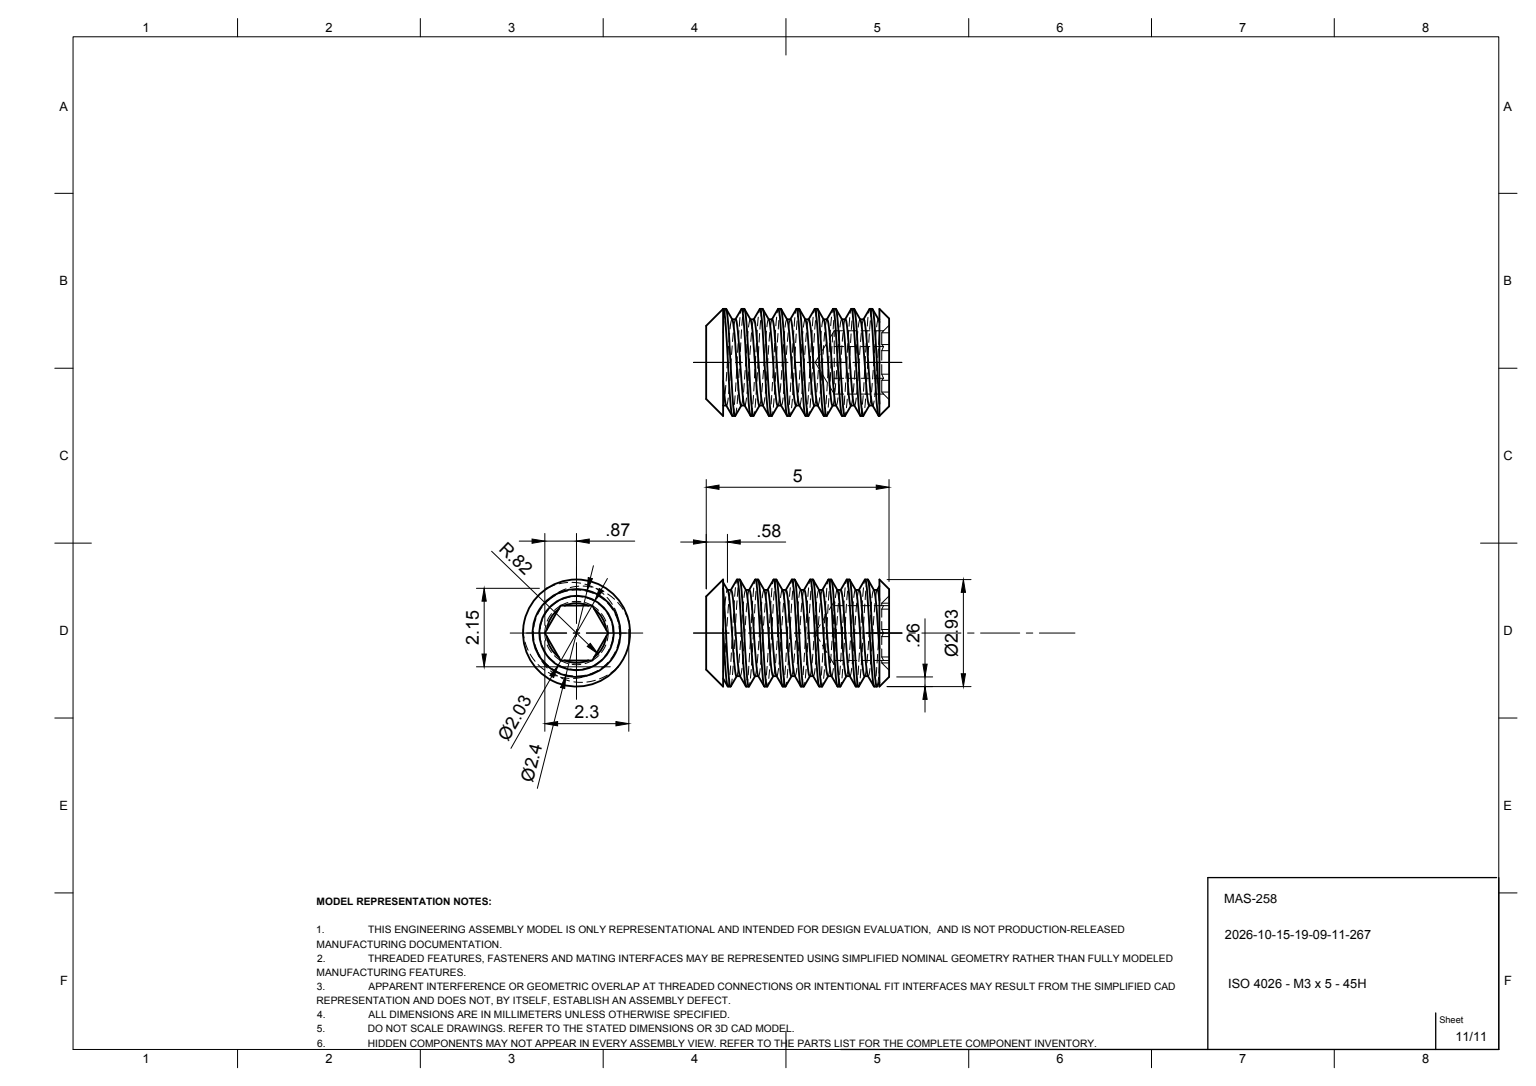
ISO-10303-21;
HEADER;
/* Generated by software containing ST-Developer
 * from STEP Tools, Inc. (www.steptools.com) 
 */

FILE_DESCRIPTION(
/* description */ (''),
/* implementation_level */ '2;1');

FILE_NAME(
/* name */ 'ISO 4026 - M3 x 5 - 45H.step',
/* time_stamp */ '2026-10-15T12:29:06-07:00',
/* author */ (''),
/* organization */ (''),
/* preprocessor_version */ 'ST-DEVELOPER v20.2',
/* originating_system */ 'Autodesk Translation Framework v15.15.0.0',
/* authorisation */ '');

FILE_SCHEMA (('AUTOMOTIVE_DESIGN { 1 0 10303 214 3 1 1 }'));
ENDSEC;

DATA;
#10=MECHANICAL_DESIGN_GEOMETRIC_PRESENTATION_REPRESENTATION('',(#1747),#135282);
#104=(
BOUNDED_CURVE()
B_SPLINE_CURVE(2,(#84021,#84022,#84023),.UNSPECIFIED.,.F.,.F.)
B_SPLINE_CURVE_WITH_KNOTS((3,3),(0.,0.0136874154102722),.UNSPECIFIED.)
CURVE()
GEOMETRIC_REPRESENTATION_ITEM()
RATIONAL_B_SPLINE_CURVE((1.,1.00669106236244,1.00897713804967))
REPRESENTATION_ITEM('')
);
#105=(
BOUNDED_CURVE()
B_SPLINE_CURVE(2,(#84027,#84028,#84029),.UNSPECIFIED.,.F.,.F.)
B_SPLINE_CURVE_WITH_KNOTS((3,3),(0.0278942541126666,0.0415816695229379),
 .UNSPECIFIED.)
CURVE()
GEOMETRIC_REPRESENTATION_ITEM()
RATIONAL_B_SPLINE_CURVE((1.00897713804926,1.00669106236213,1.))
REPRESENTATION_ITEM('')
);
#106=(
BOUNDED_CURVE()
B_SPLINE_CURVE(2,(#84031,#84032,#84033),.UNSPECIFIED.,.F.,.F.)
B_SPLINE_CURVE_WITH_KNOTS((3,3),(0.,0.0136874154102634),.UNSPECIFIED.)
CURVE()
GEOMETRIC_REPRESENTATION_ITEM()
RATIONAL_B_SPLINE_CURVE((1.,1.00669106236278,1.00897713805013))
REPRESENTATION_ITEM('')
);
#107=(
BOUNDED_CURVE()
B_SPLINE_CURVE(2,(#84037,#84038,#84039),.UNSPECIFIED.,.F.,.F.)
B_SPLINE_CURVE_WITH_KNOTS((3,3),(0.0278942541126795,0.04158166952294),
 .UNSPECIFIED.)
CURVE()
GEOMETRIC_REPRESENTATION_ITEM()
RATIONAL_B_SPLINE_CURVE((1.00897713805013,1.00669106236278,1.))
REPRESENTATION_ITEM('')
);
#108=(
BOUNDED_CURVE()
B_SPLINE_CURVE(2,(#84041,#84042,#84043),.UNSPECIFIED.,.F.,.F.)
B_SPLINE_CURVE_WITH_KNOTS((3,3),(0.,0.0136874154102606),.UNSPECIFIED.)
CURVE()
GEOMETRIC_REPRESENTATION_ITEM()
RATIONAL_B_SPLINE_CURVE((1.,1.00669106236282,1.00897713805019))
REPRESENTATION_ITEM('')
);
#109=(
BOUNDED_CURVE()
B_SPLINE_CURVE(2,(#84047,#84048,#84049),.UNSPECIFIED.,.F.,.F.)
B_SPLINE_CURVE_WITH_KNOTS((3,3),(0.0278942541126748,0.0415816695229379),
 .UNSPECIFIED.)
CURVE()
GEOMETRIC_REPRESENTATION_ITEM()
RATIONAL_B_SPLINE_CURVE((1.00897713805094,1.00669106236338,1.))
REPRESENTATION_ITEM('')
);
#110=(
BOUNDED_CURVE()
B_SPLINE_CURVE(2,(#84051,#84052,#84053),.UNSPECIFIED.,.F.,.F.)
B_SPLINE_CURVE_WITH_KNOTS((3,3),(0.,0.0136874154102637),.UNSPECIFIED.)
CURVE()
GEOMETRIC_REPRESENTATION_ITEM()
RATIONAL_B_SPLINE_CURVE((1.,1.00669106236329,1.00897713805081))
REPRESENTATION_ITEM('')
);
#111=(
BOUNDED_CURVE()
B_SPLINE_CURVE(2,(#84057,#84058,#84059),.UNSPECIFIED.,.F.,.F.)
B_SPLINE_CURVE_WITH_KNOTS((3,3),(0.0278942541126709,0.0415816695229372),
 .UNSPECIFIED.)
CURVE()
GEOMETRIC_REPRESENTATION_ITEM()
RATIONAL_B_SPLINE_CURVE((1.0089771380492,1.00669106236209,1.))
REPRESENTATION_ITEM('')
);
#112=(
BOUNDED_CURVE()
B_SPLINE_CURVE(2,(#84061,#84062,#84063),.UNSPECIFIED.,.F.,.F.)
B_SPLINE_CURVE_WITH_KNOTS((3,3),(0.,0.0136874154102607),.UNSPECIFIED.)
CURVE()
GEOMETRIC_REPRESENTATION_ITEM()
RATIONAL_B_SPLINE_CURVE((1.,1.00669106236278,1.00897713805013))
REPRESENTATION_ITEM('')
);
#113=(
BOUNDED_CURVE()
B_SPLINE_CURVE(2,(#84067,#84068,#84069),.UNSPECIFIED.,.F.,.F.)
B_SPLINE_CURVE_WITH_KNOTS((3,3),(0.0278942541126766,0.04158166952294),
 .UNSPECIFIED.)
CURVE()
GEOMETRIC_REPRESENTATION_ITEM()
RATIONAL_B_SPLINE_CURVE((1.00897713805013,1.00669106236278,1.))
REPRESENTATION_ITEM('')
);
#114=(
BOUNDED_CURVE()
B_SPLINE_CURVE(2,(#84071,#84072,#84073),.UNSPECIFIED.,.F.,.F.)
B_SPLINE_CURVE_WITH_KNOTS((3,3),(0.,0.0136874154102674),.UNSPECIFIED.)
CURVE()
GEOMETRIC_REPRESENTATION_ITEM()
RATIONAL_B_SPLINE_CURVE((1.,1.0066910623627,1.00897713805002))
REPRESENTATION_ITEM('')
);
#115=(
BOUNDED_CURVE()
B_SPLINE_CURVE(2,(#84076,#84077,#84078),.UNSPECIFIED.,.F.,.F.)
B_SPLINE_CURVE_WITH_KNOTS((3,3),(0.0278942541126671,0.0415816695229421),
 .UNSPECIFIED.)
CURVE()
GEOMETRIC_REPRESENTATION_ITEM()
RATIONAL_B_SPLINE_CURVE((1.00897713804893,1.00669106236189,1.))
REPRESENTATION_ITEM('')
);
#609=B_SPLINE_SURFACE_WITH_KNOTS('',3,3,((#83357,#83358,#83359,#83360,#83361,
#83362,#83363,#83364,#83365,#83366,#83367,#83368,#83369,#83370,#83371,#83372,
#83373,#83374,#83375,#83376,#83377,#83378,#83379,#83380,#83381,#83382,#83383,
#83384,#83385,#83386,#83387,#83388,#83389,#83390,#83391,#83392,#83393,#83394,
#83395,#83396,#83397,#83398,#83399,#83400,#83401,#83402,#83403,#83404,#83405,
#83406,#83407,#83408,#83409,#83410,#83411,#83412,#83413,#83414,#83415),
(#83416,#83417,#83418,#83419,#83420,#83421,#83422,#83423,#83424,#83425,
#83426,#83427,#83428,#83429,#83430,#83431,#83432,#83433,#83434,#83435,#83436,
#83437,#83438,#83439,#83440,#83441,#83442,#83443,#83444,#83445,#83446,#83447,
#83448,#83449,#83450,#83451,#83452,#83453,#83454,#83455,#83456,#83457,#83458,
#83459,#83460,#83461,#83462,#83463,#83464,#83465,#83466,#83467,#83468,#83469,
#83470,#83471,#83472,#83473,#83474),(#83475,#83476,#83477,#83478,#83479,
#83480,#83481,#83482,#83483,#83484,#83485,#83486,#83487,#83488,#83489,#83490,
#83491,#83492,#83493,#83494,#83495,#83496,#83497,#83498,#83499,#83500,#83501,
#83502,#83503,#83504,#83505,#83506,#83507,#83508,#83509,#83510,#83511,#83512,
#83513,#83514,#83515,#83516,#83517,#83518,#83519,#83520,#83521,#83522,#83523,
#83524,#83525,#83526,#83527,#83528,#83529,#83530,#83531,#83532,#83533),
(#83534,#83535,#83536,#83537,#83538,#83539,#83540,#83541,#83542,#83543,
#83544,#83545,#83546,#83547,#83548,#83549,#83550,#83551,#83552,#83553,#83554,
#83555,#83556,#83557,#83558,#83559,#83560,#83561,#83562,#83563,#83564,#83565,
#83566,#83567,#83568,#83569,#83570,#83571,#83572,#83573,#83574,#83575,#83576,
#83577,#83578,#83579,#83580,#83581,#83582,#83583,#83584,#83585,#83586,#83587,
#83588,#83589,#83590,#83591,#83592)),.UNSPECIFIED.,.F.,.F.,.F.,(4,4),(4,
1,1,1,1,1,1,1,1,1,1,1,1,1,1,1,1,1,1,1,1,1,1,1,1,1,1,1,1,1,1,1,1,1,1,1,1,
1,1,1,1,1,1,1,1,1,1,1,1,1,1,1,1,1,1,1,4),(-0.000249795523849274,0.0332892348118687),
(8.30174248738077,9.29791605267402,10.2937959510397,11.2896758494053,12.285555747771,
13.2814356461366,14.2773155445023,15.2731954428679,16.2690753412336,17.2649552395992,
18.2608351379649,19.2567150363305,20.2525949346962,21.2484748330618,22.2443547314275,
23.2402346297932,24.2361145281588,25.2319944265245,26.2278743248901,27.2237542232558,
28.2196341216214,29.2155140199871,30.2113939183527,31.2072738167184,32.203153715084,
33.1990336134497,34.1949135118153,35.190793410181,36.1866733085466,37.1825532069123,
38.1784331052779,39.1743130036436,40.1701929020092,41.1660728003749,42.1619526987405,
43.1578325971062,44.1537124954719,45.1495923938375,46.1454722922032,47.1413521905688,
48.1372320889345,49.1331119873001,50.1289918856658,51.1248717840314,52.1207516823971,
53.1166315807627,54.1125114791284,55.108391377494,56.1042712758597,57.1001511742253,
58.096031072591,59.0919109709566,60.0877908693223,61.0836707676879,62.0795506660536,
63.0754305644193,64.0715602583087),.UNSPECIFIED.);
#610=B_SPLINE_SURFACE_WITH_KNOTS('',3,3,((#83776,#83777,#83778,#83779,#83780,
#83781,#83782,#83783,#83784,#83785,#83786,#83787,#83788,#83789,#83790,#83791,
#83792,#83793,#83794,#83795,#83796,#83797,#83798,#83799,#83800,#83801,#83802,
#83803,#83804,#83805,#83806,#83807,#83808,#83809,#83810,#83811,#83812,#83813,
#83814,#83815,#83816,#83817,#83818,#83819,#83820,#83821,#83822,#83823,#83824,
#83825,#83826,#83827,#83828,#83829,#83830,#83831,#83832,#83833,#83834),
(#83835,#83836,#83837,#83838,#83839,#83840,#83841,#83842,#83843,#83844,
#83845,#83846,#83847,#83848,#83849,#83850,#83851,#83852,#83853,#83854,#83855,
#83856,#83857,#83858,#83859,#83860,#83861,#83862,#83863,#83864,#83865,#83866,
#83867,#83868,#83869,#83870,#83871,#83872,#83873,#83874,#83875,#83876,#83877,
#83878,#83879,#83880,#83881,#83882,#83883,#83884,#83885,#83886,#83887,#83888,
#83889,#83890,#83891,#83892,#83893),(#83894,#83895,#83896,#83897,#83898,
#83899,#83900,#83901,#83902,#83903,#83904,#83905,#83906,#83907,#83908,#83909,
#83910,#83911,#83912,#83913,#83914,#83915,#83916,#83917,#83918,#83919,#83920,
#83921,#83922,#83923,#83924,#83925,#83926,#83927,#83928,#83929,#83930,#83931,
#83932,#83933,#83934,#83935,#83936,#83937,#83938,#83939,#83940,#83941,#83942,
#83943,#83944,#83945,#83946,#83947,#83948,#83949,#83950,#83951,#83952),
(#83953,#83954,#83955,#83956,#83957,#83958,#83959,#83960,#83961,#83962,
#83963,#83964,#83965,#83966,#83967,#83968,#83969,#83970,#83971,#83972,#83973,
#83974,#83975,#83976,#83977,#83978,#83979,#83980,#83981,#83982,#83983,#83984,
#83985,#83986,#83987,#83988,#83989,#83990,#83991,#83992,#83993,#83994,#83995,
#83996,#83997,#83998,#83999,#84000,#84001,#84002,#84003,#84004,#84005,#84006,
#84007,#84008,#84009,#84010,#84011)),.UNSPECIFIED.,.F.,.F.,.F.,(4,4),(4,
1,1,1,1,1,1,1,1,1,1,1,1,1,1,1,1,1,1,1,1,1,1,1,1,1,1,1,1,1,1,1,1,1,1,1,1,
1,1,1,1,1,1,1,1,1,1,1,1,1,1,1,1,1,1,1,4),(-0.00050668484467729,0.0332453436260118),
(11.6156899717586,12.6118196458661,13.6076995442317,14.6035794425974,15.599459340963,
16.5953392393287,17.5912191376943,18.58709903606,19.5829789344256,20.5788588327913,
21.5747387311569,22.5706186295226,23.5664985278882,24.5623784262539,25.5582583246196,
26.5541382229852,27.5500181213509,28.5458980197165,29.5417779180822,30.5376578164478,
31.5335377148135,32.5294176131791,33.5252975115448,34.5211774099104,35.5170573082761,
36.5129372066417,37.5088171050074,38.504697003373,39.5005769017387,40.4964568001043,
41.49233669847,42.4882165968357,43.4840964952013,44.479976393567,45.4758562919326,
46.4717361902983,47.4676160886639,48.4634959870296,49.4593758853952,50.4552557837609,
51.4511356821265,52.4470155804922,53.4428954788578,54.4387753772235,55.4346552755891,
56.4305351739548,57.4264150723205,58.4222949706861,59.4181748690518,60.4140547674174,
61.4099346657831,62.4058145641487,63.4016944625144,64.39757436088,65.3934542592457,
66.3893341576113,67.3855077216014),.UNSPECIFIED.);
#1376=B_SPLINE_CURVE_WITH_KNOTS('',3,(#77159,#77160,#77161,#77162,#77163,
#77164,#77165,#77166,#77167,#77168,#77169,#77170,#77171,#77172,#77173,#77174,
#77175,#77176,#77177,#77178,#77179,#77180,#77181,#77182,#77183,#77184,#77185,
#77186,#77187,#77188,#77189,#77190,#77191,#77192,#77193,#77194,#77195,#77196,
#77197,#77198,#77199,#77200,#77201,#77202,#77203,#77204,#77205,#77206,#77207,
#77208,#77209,#77210,#77211,#77212,#77213,#77214,#77215,#77216),
 .UNSPECIFIED.,.F.,.F.,(4,2,2,2,2,2,2,2,2,2,2,2,2,2,2,2,2,2,2,2,2,2,2,2,
2,2,2,2,4),(-1.21754206946651,-1.17821980543779,-1.16405746250061,-1.15855947211459,
-1.1545321686619,-1.15022795752816,-1.14324756109432,-1.11173425539269,
-1.09692945396154,-1.08835253727485,-1.08512595789204,-1.08284305354597,
-1.08021521852638,-1.07520106907232,-1.05375326158949,-1.03212994516716,
-1.01905512594296,-1.01371235037151,-1.00971978407183,-1.00537977987688,
-0.998174601131823,-0.963190262851774,-0.950068242946656,-0.942099905926401,
-0.938979922381813,-0.936737330856261,-0.934120072671351,-0.929211478009695,
-0.921419482998929),.UNSPECIFIED.);
#1377=B_SPLINE_CURVE_WITH_KNOTS('',3,(#77219,#77220,#77221,#77222,#77223,
#77224,#77225,#77226,#77227,#77228,#77229,#77230,#77231,#77232,#77233,#77234,
#77235,#77236,#77237,#77238,#77239,#77240,#77241,#77242,#77243,#77244,#77245,
#77246,#77247,#77248,#77249),.UNSPECIFIED.,.F.,.F.,(4,3,3,3,3,3,3,3,3,3,
4),(0.,0.115845454600529,0.231625391685987,0.347372408915667,0.4631235693031,
0.578915929492123,0.69488330926515,0.810943764469935,0.927248476443398,
0.99587989836565,1.12274180646096),.UNSPECIFIED.);
#1378=B_SPLINE_CURVE_WITH_KNOTS('',3,(#77254,#77255,#77256,#77257,#77258,
#77259,#77260,#77261,#77262,#77263,#77264,#77265,#77266,#77267,#77268,#77269,
#77270,#77271,#77272,#77273,#77274,#77275,#77276,#77277,#77278,#77279,#77280,
#77281,#77282,#77283,#77284,#77285,#77286,#77287,#77288,#77289,#77290,#77291,
#77292,#77293,#77294,#77295,#77296,#77297,#77298,#77299,#77300,#77301,#77302,
#77303,#77304,#77305,#77306,#77307,#77308,#77309,#77310,#77311,#77312,#77313,
#77314,#77315,#77316,#77317,#77318,#77319,#77320,#77321,#77322,#77323,#77324,
#77325,#77326,#77327,#77328,#77329,#77330,#77331,#77332,#77333,#77334,#77335,
#77336,#77337,#77338,#77339,#77340,#77341,#77342,#77343,#77344,#77345,#77346,
#77347,#77348,#77349,#77350,#77351,#77352,#77353,#77354,#77355,#77356,#77357,
#77358,#77359,#77360,#77361,#77362,#77363,#77364,#77365,#77366,#77367,#77368,
#77369,#77370,#77371,#77372,#77373,#77374,#77375,#77376,#77377,#77378,#77379,
#77380,#77381,#77382,#77383,#77384,#77385,#77386,#77387,#77388,#77389,#77390,
#77391,#77392,#77393,#77394,#77395,#77396,#77397,#77398,#77399,#77400,#77401,
#77402,#77403,#77404,#77405,#77406,#77407,#77408,#77409,#77410,#77411,#77412,
#77413,#77414,#77415,#77416,#77417,#77418,#77419,#77420,#77421,#77422,#77423,
#77424,#77425),.UNSPECIFIED.,.F.,.F.,(4,2,2,2,2,2,2,2,2,2,2,2,2,2,2,2,2,
2,2,2,2,2,2,2,2,2,2,2,2,2,2,2,2,2,2,2,2,2,2,2,2,2,2,2,2,2,2,2,2,2,2,2,2,
2,2,2,2,2,2,2,2,2,2,2,2,2,2,2,2,2,2,2,2,2,2,2,2,2,2,2,2,2,2,2,2,4),(-0.921419482998929,
-0.907688316791177,-0.885977525693296,-0.872886081562645,-0.867573627709282,
-0.863620021806596,-0.859340338471167,-0.852285820281842,-0.817068960538186,
-0.803848529175472,-0.795853892356727,-0.792748022050185,-0.7905163487824,
-0.787901135493465,-0.783029899170039,-0.763563232406315,-0.745175363618844,
-0.727769961376288,-0.721951181979324,-0.717894343967278,-0.713735439938429,
-0.707376468863512,-0.68265736518924,-0.66121073259976,-0.650652455375354,
-0.647221057566939,-0.644928541426486,-0.642442848946966,-0.638067258217649,
-0.608821864626192,-0.58498089779175,-0.577643940843088,-0.573291994864995,
-0.569330639238763,-0.564094456953282,-0.551677011438918,-0.53193566151644,
-0.507251176775778,-0.502465995418774,-0.499868632875132,-0.497623283392536,
-0.494462217094089,-0.486137962898804,-0.472047790880579,-0.43783436812367,
-0.431066025429978,-0.426831354822855,-0.422832748507351,-0.41731951470546,
-0.40276097029277,-0.376056281360347,-0.359534421781043,-0.355618511890536,
-0.353232508861721,-0.350881150748675,-0.347133669219491,-0.332694769079542,
-0.314588300276116,-0.290783010636688,-0.284507014961167,-0.280367699863515,
-0.276304767597177,-0.270432530198454,-0.252375906212504,-0.234530960463338,
-0.2153034103759,-0.210445276682928,-0.207832350266125,-0.205589527875254,
-0.202453875215916,-0.194323277172034,-0.180756703969854,-0.145451744314263,
-0.138838184308752,-0.134632742059005,-0.130615121903102,-0.124997860543144,
-0.109547987206611,-0.0788702916803572,-0.0669285629089969,-0.063284529861049,
-0.0611845516338545,-0.0588379538520908,-0.0551131392442454,-0.0410185576883546,
-6.1401681533555E-5),.UNSPECIFIED.);
#1379=B_SPLINE_CURVE_WITH_KNOTS('',3,(#77426,#77427,#77428,#77429,#77430,
#77431,#77432,#77433,#77434,#77435,#77436,#77437,#77438,#77439,#77440,#77441,
#77442,#77443,#77444,#77445,#77446,#77447,#77448,#77449,#77450,#77451,#77452,
#77453,#77454,#77455,#77456,#77457,#77458,#77459,#77460,#77461,#77462,#77463,
#77464,#77465,#77466,#77467,#77468,#77469,#77470,#77471,#77472,#77473,#77474,
#77475,#77476,#77477,#77478,#77479,#77480,#77481,#77482,#77483,#77484,#77485,
#77486,#77487,#77488,#77489,#77490,#77491,#77492,#77493,#77494,#77495,#77496,
#77497,#77498,#77499,#77500,#77501,#77502,#77503,#77504,#77505,#77506,#77507,
#77508,#77509,#77510,#77511,#77512,#77513,#77514,#77515,#77516,#77517,#77518,
#77519,#77520,#77521,#77522,#77523,#77524,#77525,#77526,#77527,#77528,#77529,
#77530,#77531,#77532,#77533,#77534,#77535,#77536,#77537,#77538,#77539,#77540,
#77541,#77542,#77543,#77544,#77545,#77546,#77547,#77548,#77549,#77550,#77551,
#77552,#77553,#77554,#77555,#77556,#77557,#77558,#77559,#77560,#77561,#77562,
#77563,#77564,#77565,#77566,#77567,#77568,#77569,#77570,#77571,#77572,#77573,
#77574,#77575,#77576,#77577,#77578,#77579,#77580,#77581,#77582,#77583,#77584,
#77585,#77586,#77587,#77588,#77589,#77590,#77591,#77592,#77593,#77594,#77595,
#77596,#77597,#77598,#77599,#77600,#77601,#77602,#77603,#77604,#77605,#77606,
#77607,#77608,#77609,#77610,#77611,#77612,#77613,#77614,#77615,#77616,#77617,
#77618,#77619,#77620,#77621,#77622,#77623,#77624,#77625,#77626,#77627,#77628,
#77629,#77630,#77631,#77632,#77633,#77634,#77635,#77636,#77637,#77638,#77639),
 .UNSPECIFIED.,.F.,.F.,(4,3,3,3,3,3,3,3,3,3,3,3,3,3,3,3,3,3,3,3,3,3,3,3,
3,3,3,3,3,3,3,3,3,3,3,3,3,3,3,3,3,3,3,3,3,3,3,3,3,3,3,3,3,3,3,3,3,3,3,3,
3,3,3,3,3,3,3,3,3,3,3,4),(1.12274180646096,1.23373504789904,1.34459002212884,
1.45535479623447,1.55989672892336,1.56607726185873,1.67688568467484,1.78773354109534,
1.89879266001346,1.99171671473048,1.9917597967313,2.09518566569704,2.10522016410668,
2.21847423059868,2.33161337714145,2.4446824646528,2.55772625044323,2.67087099529545,
2.78406492035342,2.89747197121009,2.9876011371121,2.98763969509696,3.09165900030874,
3.10124740420088,3.21465736692644,3.32795751893579,3.44119241833077,3.55440652592882,
3.6677272400545,3.7811005346835,3.89469031251206,3.9834802329205,3.98351959346261,
4.08724850520171,4.09685637681465,4.20998806900548,4.32300567198192,4.43595426307203,
4.54887881688974,4.66190726618895,4.77498633572913,4.88828238191216,4.97935950968077,
4.97939949182826,5.08314209235908,5.09284419837543,5.20608568010895,5.31921413328377,
5.43227443626529,5.54531136614965,5.65845232226374,5.77164415146343,5.88505194316747,
5.97523993044046,5.97527939019391,6.07908252879731,6.08873073478065,6.20197956676853,
6.3151158004847,6.42818430022515,6.54122982955544,6.65437994550042,6.76758125938584,
6.88099895560384,6.97111969950722,6.97115928855956,7.07900809076849,7.09416685512428,
7.21066939468956,7.21683096983575,7.33897298823794,7.40592711304532),
 .UNSPECIFIED.);
#1380=B_SPLINE_CURVE_WITH_KNOTS('',3,(#77644,#77645,#77646,#77647,#77648,
#77649,#77650,#77651,#77652,#77653,#77654,#77655,#77656,#77657,#77658,#77659,
#77660,#77661,#77662,#77663,#77664,#77665,#77666,#77667,#77668,#77669,#77670,
#77671,#77672,#77673,#77674,#77675,#77676,#77677,#77678,#77679,#77680,#77681,
#77682,#77683,#77684,#77685,#77686,#77687,#77688,#77689,#77690,#77691,#77692,
#77693,#77694,#77695,#77696,#77697,#77698,#77699,#77700,#77701,#77702,#77703,
#77704,#77705,#77706,#77707,#77708,#77709,#77710,#77711,#77712,#77713,#77714,
#77715,#77716,#77717,#77718,#77719,#77720,#77721,#77722,#77723,#77724,#77725,
#77726,#77727,#77728,#77729,#77730,#77731,#77732,#77733,#77734,#77735,#77736,
#77737,#77738,#77739,#77740,#77741,#77742,#77743,#77744,#77745,#77746,#77747,
#77748,#77749,#77750,#77751,#77752,#77753,#77754,#77755,#77756,#77757,#77758,
#77759,#77760,#77761,#77762,#77763,#77764,#77765,#77766,#77767,#77768,#77769,
#77770,#77771,#77772,#77773,#77774,#77775,#77776,#77777,#77778,#77779,#77780,
#77781,#77782,#77783,#77784,#77785,#77786,#77787,#77788,#77789,#77790,#77791,
#77792,#77793,#77794,#77795,#77796,#77797,#77798,#77799,#77800,#77801,#77802,
#77803,#77804,#77805,#77806,#77807,#77808,#77809,#77810,#77811,#77812,#77813,
#77814,#77815,#77816,#77817,#77818,#77819,#77820,#77821,#77822,#77823,#77824,
#77825,#77826,#77827,#77828,#77829,#77830,#77831,#77832,#77833,#77834,#77835,
#77836,#77837,#77838,#77839,#77840,#77841,#77842,#77843,#77844,#77845,#77846,
#77847,#77848,#77849,#77850,#77851,#77852,#77853,#77854),.UNSPECIFIED.,
 .F.,.F.,(4,3,3,3,3,3,3,3,3,3,3,3,3,3,3,3,3,3,3,3,3,3,3,3,3,3,3,3,3,3,3,
3,3,3,3,3,3,3,3,3,3,3,3,3,3,3,3,3,3,3,3,3,3,3,3,3,3,3,3,3,3,3,3,3,3,3,3,
3,3,3,4),(-16.6574965103488,-16.5463313103564,-16.4343301060372,-16.322344109605,
-16.2102494790042,-16.0980936348029,-15.9924244225728,-15.9857348554638,
-15.934117974039,-15.9340783738505,-15.8303032419388,-15.8206442770722,
-15.7074132532074,-15.5942951569007,-15.4812450908478,-15.3682182588957,
-15.2550871008504,-15.1419049191215,-15.0285064012669,-14.938238075336,
-14.9381984754848,-14.8344232571971,-14.8247643455127,-14.7115332877515,
-14.5984151571454,-14.4853650564546,-14.3723381895906,-14.2592069964952,
-14.1460247795845,-14.0326262267835,-13.942358177767,-13.9423185771191,
-13.8385435760761,-13.8288846569355,-13.7156538090858,-13.6025358883135,
-13.4894859970134,-13.3764593387315,-13.2633283513034,-13.1501463387721,
-13.0367479856472,-12.9464782790693,-12.9464386787535,-12.8426635582421,
-12.8330044289798,-12.7197732542598,-12.6066550085104,-12.4936047946711,
-12.380577816835,-12.2674465169873,-12.1542641954907,-12.0408655429596,
-11.9505983780519,-11.9505587803878,-11.8467830017773,-11.8371243762114,
-11.7238930404563,-11.6107746297512,-11.4977242473709,-11.384697097739,
-11.2715656225024,-11.1583831233508,-11.0449842917532,-10.9547184870581,
-10.9546788820222,-10.8497976193126,-10.8389884949821,-10.7230435781436,
-10.6077612699342,-10.4914850487812,-10.3752088276281),.UNSPECIFIED.);
#1381=B_SPLINE_CURVE_WITH_KNOTS('',3,(#77855,#77856,#77857,#77858,#77859,
#77860,#77861,#77862,#77863,#77864,#77865,#77866,#77867,#77868,#77869,#77870,
#77871,#77872,#77873,#77874,#77875,#77876,#77877,#77878,#77879,#77880,#77881,
#77882,#77883,#77884,#77885,#77886,#77887,#77888,#77889,#77890,#77891,#77892,
#77893,#77894,#77895,#77896,#77897,#77898,#77899,#77900,#77901,#77902,#77903,
#77904,#77905,#77906,#77907,#77908,#77909,#77910,#77911,#77912,#77913,#77914,
#77915,#77916,#77917,#77918,#77919,#77920,#77921,#77922,#77923,#77924,#77925,
#77926,#77927,#77928,#77929,#77930,#77931,#77932,#77933,#77934,#77935,#77936,
#77937,#77938,#77939,#77940,#77941,#77942,#77943,#77944,#77945,#77946,#77947,
#77948,#77949,#77950,#77951,#77952,#77953,#77954,#77955,#77956,#77957,#77958,
#77959,#77960,#77961,#77962,#77963,#77964,#77965,#77966,#77967,#77968,#77969,
#77970,#77971,#77972,#77973,#77974,#77975,#77976,#77977,#77978,#77979,#77980,
#77981,#77982,#77983,#77984,#77985,#77986,#77987,#77988,#77989,#77990,#77991,
#77992,#77993,#77994,#77995,#77996,#77997,#77998,#77999,#78000,#78001,#78002,
#78003,#78004,#78005,#78006,#78007,#78008,#78009,#78010,#78011,#78012,#78013,
#78014,#78015,#78016,#78017,#78018,#78019,#78020,#78021,#78022,#78023,#78024,
#78025,#78026,#78027,#78028,#78029,#78030,#78031,#78032,#78033,#78034,#78035,
#78036,#78037,#78038),.UNSPECIFIED.,.F.,.F.,(4,2,2,2,2,2,2,2,2,2,2,2,2,
2,2,2,2,2,2,2,2,2,2,2,2,2,2,2,2,2,2,2,2,2,2,2,2,2,2,2,2,2,2,2,2,2,2,2,2,
2,2,2,2,2,2,2,2,2,2,2,2,2,2,2,2,2,2,2,2,2,2,2,2,2,2,2,2,2,2,2,2,2,2,2,2,
2,2,2,2,2,2,4),(7.55331046094257E-5,0.00311488062742005,0.00589275104345637,
0.00957822560877077,0.0136874178462499,0.0196924847782724,0.0409279650768497,
0.0549894800395652,0.0692347333575978,0.0750056140336835,0.0794705133763708,
0.0819628446481993,0.0841961839693353,0.0869680298364656,0.0940489209653037,
0.129814111425115,0.146099950504705,0.151785217588427,0.155795564055968,
0.159453751928995,0.165433805290373,0.182940478931749,0.207240700533897,
0.222307455662279,0.226079429552293,0.228426586761477,0.23078666401458,
0.234620974103604,0.249432251355507,0.277557223302338,0.292445953223121,
0.297979106518716,0.301963020846168,0.306155184921126,0.312793013872007,
0.347827135873415,0.361540513352248,0.369716897813443,0.372846972694969,
0.375076835859076,0.377660756070977,0.382430268818484,0.405438098633203,
0.426320205326456,0.439129906572397,0.44439978553307,0.448343075832583,
0.452631913781975,0.459751362689939,0.494720362864264,0.507857683034686,
0.51581555707109,0.518915196993098,0.521141161944093,0.523742195593142,
0.528592249214605,0.547902250767208,0.565126197412152,0.583669666253345,
0.589560417299322,0.593607282150156,0.597705592918242,0.603867947078983,
0.624922258499583,0.655514298780022,0.662278005328982,0.665197397890851,
0.667196094429105,0.669816617220415,0.67475964111456,0.696085820423846,
0.717922799335886,0.731055622848822,0.736369783015217,0.740319640023491,
0.744590515419098,0.751619654650834,0.783667918036271,0.798887961548889,
0.80760501751015,0.810806816097925,0.813046735586465,0.815593959750254,
0.820191227049956,0.846466054625532,0.865368695833238,0.877457066491806,
0.882624456523596,0.886554289123994,0.890890438772885,0.898244410878047,
0.921379800955709),.UNSPECIFIED.);
#1382=B_SPLINE_CURVE_WITH_KNOTS('',3,(#78044,#78045,#78046,#78047,#78048,
#78049,#78050,#78051,#78052,#78053,#78054,#78055,#78056,#78057,#78058,#78059,
#78060,#78061,#78062,#78063,#78064,#78065,#78066,#78067,#78068,#78069,#78070,
#78071,#78072,#78073,#78074,#78075,#78076,#78077,#78078,#78079,#78080,#78081,
#78082,#78083,#78084,#78085,#78086,#78087,#78088,#78089,#78090,#78091,#78092,
#78093,#78094,#78095,#78096,#78097,#78098,#78099,#78100,#78101,#78102,#78103,
#78104,#78105,#78106,#78107,#78108,#78109,#78110,#78111,#78112,#78113,#78114,
#78115,#78116,#78117,#78118,#78119,#78120,#78121,#78122,#78123,#78124,#78125,
#78126,#78127,#78128,#78129,#78130,#78131,#78132,#78133,#78134,#78135,#78136,
#78137,#78138,#78139,#78140,#78141,#78142,#78143,#78144,#78145,#78146,#78147,
#78148,#78149,#78150,#78151,#78152,#78153,#78154,#78155,#78156,#78157,#78158,
#78159,#78160,#78161,#78162,#78163,#78164,#78165,#78166,#78167,#78168,#78169,
#78170,#78171,#78172,#78173,#78174,#78175,#78176,#78177,#78178,#78179,#78180,
#78181,#78182,#78183,#78184,#78185,#78186,#78187,#78188,#78189,#78190,#78191,
#78192,#78193,#78194,#78195,#78196,#78197,#78198,#78199,#78200,#78201,#78202,
#78203,#78204,#78205,#78206,#78207,#78208,#78209,#78210,#78211,#78212,#78213,
#78214,#78215,#78216,#78217,#78218,#78219,#78220,#78221,#78222,#78223),
 .UNSPECIFIED.,.F.,.F.,(4,2,2,2,2,2,2,2,2,2,2,2,2,2,2,2,2,2,2,2,2,2,2,2,
2,2,2,2,2,2,2,2,2,2,2,2,2,2,2,2,2,2,2,2,2,2,2,2,2,2,2,2,2,2,2,2,2,2,2,2,
2,2,2,2,2,2,2,2,2,2,2,2,2,2,2,2,2,2,2,2,2,2,2,2,2,2,2,2,2,4),(0.921350305018577,
0.921389876624562,0.924778351317925,0.927037052310556,0.929523336688975,
0.933909319231592,0.956539494608926,0.987309347251915,0.994485423914873,
0.998803284581335,1.00277147317402,1.00807376621736,1.02097866000226,1.04210375396098,
1.0645803887481,1.06942020706886,1.07202853433207,1.0742712679726,1.07741171247261,
1.08558062454395,1.09925152423885,1.13435370175234,1.14099825146805,1.14520924348174,
1.14922237985182,1.15481702416113,1.17007308473251,1.19982027276487,1.21271906572539,
1.21644741108376,1.21856275817168,1.22089123008652,1.22452877455692,1.23742122425125,
1.27188899511206,1.28349027612361,1.28869318828847,1.29266019279346,1.29698089226977,
1.30417190236956,1.32646153627304,1.35215637825488,1.35995878365049,1.36312058726059,
1.36536602189029,1.36796236389115,1.37288653830946,1.39177683800695,1.42619710890516,
1.43293802757295,1.43716799625277,1.44117067547864,1.44670370535482,1.46142612404115,
1.48881206170003,1.50445213009386,1.50832697709802,1.51070479095477,1.51306379954949,
1.51685016199031,1.53193445644289,1.55624909699754,1.57386860269962,1.57980106586157,
1.58346687670161,1.58751537895101,1.59331612571466,1.61059459442548,1.62861744095523,
1.64849768185189,1.65339889357475,1.65601991617009,1.6582594648806,1.66137646992562,
1.66937874648447,1.68261100872528,1.71804363796523,1.72485063701832,1.72909376915813,
1.73308998369107,1.73858333515089,1.75297381136775,1.7790423411234,1.79629129359712,
1.80023499046673,1.80262740654097,1.80497314347554,1.8086963080364,1.82277639645548,
1.84239058989693),.UNSPECIFIED.);
#1383=B_SPLINE_CURVE_WITH_KNOTS('',3,(#78224,#78225,#78226,#78227),
 .UNSPECIFIED.,.F.,.F.,(4,4),(-16.6583941348077,-16.6574965103488),
 .UNSPECIFIED.);
#1384=B_SPLINE_CURVE_WITH_KNOTS('',3,(#78229,#78230,#78231,#78232,#78233,
#78234,#78235,#78236,#78237,#78238,#78239,#78240,#78241,#78242,#78243,#78244,
#78245,#78246,#78247,#78248,#78249,#78250,#78251,#78252,#78253,#78254,#78255,
#78256,#78257,#78258,#78259,#78260,#78261,#78262,#78263,#78264,#78265,#78266,
#78267,#78268,#78269,#78270,#78271,#78272,#78273,#78274,#78275,#78276,#78277,
#78278,#78279,#78280,#78281,#78282,#78283,#78284,#78285,#78286,#78287,#78288,
#78289,#78290,#78291,#78292,#78293,#78294,#78295,#78296,#78297,#78298,#78299,
#78300,#78301,#78302,#78303,#78304,#78305,#78306,#78307,#78308,#78309,#78310,
#78311,#78312,#78313,#78314,#78315,#78316,#78317,#78318,#78319,#78320,#78321,
#78322,#78323,#78324,#78325,#78326,#78327,#78328,#78329,#78330,#78331,#78332,
#78333,#78334,#78335,#78336,#78337,#78338,#78339,#78340,#78341,#78342,#78343,
#78344,#78345,#78346,#78347,#78348,#78349,#78350,#78351,#78352,#78353,#78354,
#78355,#78356,#78357,#78358,#78359,#78360,#78361,#78362,#78363,#78364,#78365,
#78366,#78367,#78368,#78369,#78370,#78371,#78372,#78373,#78374,#78375,#78376,
#78377,#78378,#78379,#78380,#78381,#78382,#78383,#78384,#78385,#78386,#78387,
#78388,#78389,#78390,#78391,#78392,#78393,#78394,#78395,#78396,#78397,#78398,
#78399,#78400,#78401,#78402,#78403,#78404,#78405,#78406,#78407,#78408,#78409,
#78410,#78411,#78412,#78413,#78414),.UNSPECIFIED.,.F.,.F.,(4,2,2,2,2,2,
2,2,2,2,2,2,2,2,2,2,2,2,2,2,2,2,2,2,2,2,2,2,2,2,2,2,2,2,2,2,2,2,2,2,2,2,
2,2,2,2,2,2,2,2,2,2,2,2,2,2,2,2,2,2,2,2,2,2,2,2,2,2,2,2,2,2,2,2,2,2,2,2,
2,2,2,2,2,2,2,2,2,2,2,2,2,2,4),(0.921379800955709,0.921511462072376,0.949406248900438,
0.954915878085833,0.957616084348176,0.959806098671794,0.962742035540181,
0.96960888206462,0.980108126735474,1.00265005569605,1.02138548779191,1.02742513364255,
1.03109303754262,1.03509348211883,1.04072477727184,1.05649993293572,1.08901049958424,
1.09907574790631,1.10253013184978,1.10479041416925,1.10722834732382,1.11142941842079,
1.13312603579934,1.16548672629248,1.17248247257583,1.17674652018402,1.1806986241325,
1.1860290933367,1.19928598585736,1.22150457988203,1.24240677180674,1.24725670356296,
1.24985764546148,1.25208359260461,1.25518332106303,1.26314120661243,1.27627928776522,
1.3112403102158,1.31837539785881,1.32266744792816,1.32660980377609,1.33187256392618,
1.34463145702576,1.36536819263287,1.38857317872476,1.39333372078013,1.39591574062321,
1.39814594896,1.40127939764684,1.40948097186301,1.42326311865662,1.45817393361484,
1.46483153706146,1.46902739883502,1.47300880978117,1.4785285638421,1.49330621716269,
1.52096743689291,1.53631940261687,1.5401709433473,1.54253445619872,1.54487702556269,
1.54863004027595,1.56338839100655,1.58122608546742,1.6050017060548,1.61125098564634,
1.61536591180166,1.61939852067159,1.6252131035489,1.64287033869637,1.6606426259535,
1.68037916149352,1.68525719244088,1.68786396930375,1.69008857146817,1.69317790260395,
1.70106276347702,1.71401242767589,1.74818141044997,1.75581602328968,1.76024956431239,
1.7641593971117,1.76914879252055,1.78008055903901,1.79616279955146,1.81413094267229,
1.82842328418419,1.8322129424923,1.83456320436152,1.83660820322032,1.8392493161768,
1.84253082468574),.UNSPECIFIED.);
#1385=B_SPLINE_CURVE_WITH_KNOTS('',3,(#78415,#78416,#78417,#78418),
 .UNSPECIFIED.,.F.,.F.,(4,4),(0.000123955660990716,0.0001645492752207),
 .UNSPECIFIED.);
#1386=B_SPLINE_CURVE_WITH_KNOTS('',3,(#78424,#78425,#78426,#78427),
 .UNSPECIFIED.,.F.,.F.,(4,4),(1.84262518595721,1.84272753034819),
 .UNSPECIFIED.);
#1387=B_SPLINE_CURVE_WITH_KNOTS('',3,(#78428,#78429,#78430,#78431,#78432,
#78433,#78434,#78435,#78436,#78437,#78438,#78439,#78440,#78441,#78442,#78443,
#78444,#78445,#78446,#78447,#78448,#78449,#78450,#78451,#78452,#78453,#78454,
#78455,#78456,#78457,#78458,#78459,#78460,#78461,#78462,#78463,#78464,#78465,
#78466,#78467,#78468,#78469,#78470,#78471,#78472,#78473,#78474,#78475,#78476,
#78477,#78478,#78479,#78480,#78481,#78482,#78483,#78484,#78485,#78486,#78487,
#78488,#78489,#78490,#78491,#78492,#78493,#78494,#78495,#78496,#78497,#78498,
#78499,#78500,#78501,#78502,#78503,#78504,#78505,#78506,#78507,#78508,#78509,
#78510,#78511,#78512,#78513,#78514,#78515,#78516,#78517,#78518,#78519,#78520,
#78521,#78522,#78523,#78524,#78525,#78526,#78527,#78528,#78529,#78530,#78531,
#78532,#78533,#78534,#78535,#78536,#78537,#78538,#78539,#78540,#78541,#78542,
#78543,#78544,#78545,#78546,#78547,#78548,#78549,#78550,#78551,#78552,#78553,
#78554,#78555,#78556,#78557,#78558,#78559,#78560,#78561,#78562,#78563,#78564,
#78565,#78566,#78567,#78568,#78569,#78570,#78571,#78572,#78573,#78574,#78575,
#78576,#78577,#78578,#78579,#78580,#78581,#78582,#78583,#78584,#78585,#78586,
#78587,#78588,#78589,#78590,#78591,#78592,#78593,#78594,#78595,#78596,#78597,
#78598,#78599),.UNSPECIFIED.,.F.,.F.,(4,2,2,2,2,2,2,2,2,2,2,2,2,2,2,2,2,
2,2,2,2,2,2,2,2,2,2,2,2,2,2,2,2,2,2,2,2,2,2,2,2,2,2,2,2,2,2,2,2,2,2,2,2,
2,2,2,2,2,2,2,2,2,2,2,2,2,2,2,2,2,2,2,2,2,2,2,2,2,2,2,2,2,2,2,2,4),(0.000101250613919574,
0.0302450781019042,0.0444693089741603,0.048202616836321,0.0505509261682221,
0.0529418146572406,0.0568763595433419,0.0738308452279146,0.100165398608602,
0.114628320004093,0.120131598164091,0.124130240185373,0.128371621848128,
0.135166089952892,0.169197205263441,0.183373526745438,0.191729771658096,
0.194895901941542,0.197142258991893,0.199737091617328,0.204512301270677,
0.227753295369034,0.248457049667915,0.26121689088981,0.266499614624906,
0.270465432826506,0.27479249297983,0.282012960789868,0.318171579784247,
0.334826615024971,0.339497205227342,0.342042612703549,0.344303756540027,
0.347570816901137,0.356059279481411,0.390234599894148,0.406298758104433,
0.411981482289126,0.416010022219744,0.419698990950769,0.425764705896488,
0.444622609706147,0.467061494019179,0.482443352428587,0.4862472681405,0.488610382004106,
0.490697520615568,0.494271250091231,0.505416415789197,0.536846216390167,
0.552439637728479,0.558072084942697,0.562091870391891,0.56629202441881,
0.57288091121604,0.608347517683316,0.621836962244223,0.629938062082391,
0.633069279511645,0.635311051863348,0.637924964797009,0.642790613214213,
0.663545652246991,0.684417200905839,0.698805868700279,0.704300132714303,
0.708297292275137,0.712541668231052,0.719351275541517,0.753270451451571,
0.767501439975446,0.775877538070527,0.779046303895663,0.781292986687984,
0.78388634654955,0.788654740534721,0.813455991135851,0.833121567861134,
0.845508422174809,0.850738386794919,0.854697108755072,0.859048102965697,
0.86638800917551,0.891151523568089,0.911193271661736,0.921350305018577),
 .UNSPECIFIED.);
#1388=B_SPLINE_CURVE_WITH_KNOTS('',3,(#78600,#78601,#78602,#78603,#78604,
#78605,#78606,#78607,#78608,#78609,#78610,#78611,#78612,#78613,#78614,#78615,
#78616,#78617,#78618,#78619,#78620,#78621,#78622,#78623,#78624,#78625,#78626,
#78627,#78628,#78629,#78630,#78631,#78632,#78633,#78634,#78635,#78636,#78637,
#78638,#78639,#78640,#78641,#78642,#78643,#78644,#78645,#78646,#78647,#78648,
#78649,#78650,#78651,#78652,#78653,#78654,#78655,#78656,#78657,#78658,#78659,
#78660,#78661,#78662,#78663,#78664,#78665,#78666,#78667,#78668,#78669,#78670,
#78671,#78672,#78673,#78674,#78675,#78676,#78677,#78678,#78679,#78680,#78681,
#78682,#78683,#78684,#78685,#78686,#78687,#78688,#78689,#78690,#78691,#78692,
#78693,#78694,#78695,#78696,#78697,#78698,#78699,#78700,#78701,#78702,#78703,
#78704,#78705,#78706,#78707,#78708,#78709,#78710,#78711,#78712,#78713,#78714,
#78715,#78716,#78717,#78718,#78719,#78720,#78721,#78722,#78723,#78724,#78725,
#78726,#78727,#78728,#78729,#78730,#78731,#78732,#78733,#78734,#78735,#78736,
#78737,#78738,#78739,#78740,#78741,#78742,#78743,#78744,#78745,#78746,#78747,
#78748,#78749,#78750,#78751,#78752,#78753,#78754,#78755,#78756,#78757,#78758,
#78759,#78760,#78761,#78762,#78763,#78764,#78765,#78766,#78767,#78768,#78769,
#78770,#78771,#78772,#78773),.UNSPECIFIED.,.F.,.F.,(4,2,2,2,2,2,2,2,2,2,
2,2,2,2,2,2,2,2,2,2,2,2,2,2,2,2,2,2,2,2,2,2,2,2,2,2,2,2,2,2,2,2,2,2,2,2,
2,2,2,2,2,2,2,2,2,2,2,2,2,2,2,2,2,2,2,2,2,2,2,2,2,2,2,2,2,2,2,2,2,2,2,2,
2,2,2,2,4),(0.0001645492752207,0.0231231113283336,0.0440247145262724,0.0568414829277775,
0.0621126527407258,0.0660564396362311,0.0703453847668487,0.0774640022785633,
0.108660747718192,0.131319845940176,0.135489869597789,0.137921304680615,
0.140185427288329,0.14366028213544,0.153913582838174,0.182803578276252,
0.201388672488877,0.207282905464499,0.211330470171896,0.215428123865974,
0.221586788162412,0.24252798283675,0.273214312903204,0.280000499247005,
0.28292355142068,0.285112828225382,0.287823363414176,0.293387548960966,
0.324723500013775,0.339563594116051,0.349934723300853,0.354832419533883,
0.358734943685334,0.363229968466276,0.371159132904426,0.407708492072248,
0.42402670893179,0.427865641516943,0.430226702815742,0.432291046781632,
0.435786717467062,0.446240905938236,0.478381687212749,0.494094307894705,
0.499719202510841,0.503718595034805,0.507883224011601,0.514382956291043,
0.550350705476149,0.563629030650189,0.571641195575328,0.574748671206292,
0.576975784506754,0.579572707208546,0.584402893756101,0.603309224116719,
0.619578186751874,0.632818447115015,0.642418762535818,0.647183402032388,
0.650700407219525,0.65515200889598,0.662871020297927,0.696919740217704,
0.709838242108691,0.71771166935532,0.720799650228814,0.72302441774324,0.725632684635717,
0.730516651035866,0.753022988740741,0.774118812094353,0.78700277371131,
0.792283367704293,0.796228638313861,0.800513891447624,0.807613466615827,
0.839008140632725,0.85459062049883,0.863431683566498,0.866649425094912,
0.868891847886336,0.871431721516379,0.875994372056908,0.902899908240868,
0.921434484064485,0.921536811180233),.UNSPECIFIED.);
#1389=B_SPLINE_CURVE_WITH_KNOTS('',3,(#78778,#78779,#78780,#78781,#78782,
#78783,#78784,#78785,#78786,#78787,#78788,#78789,#78790,#78791,#78792,#78793,
#78794,#78795,#78796,#78797,#78798,#78799,#78800,#78801,#78802,#78803,#78804,
#78805,#78806,#78807,#78808,#78809,#78810,#78811,#78812,#78813,#78814,#78815,
#78816,#78817,#78818,#78819,#78820,#78821,#78822,#78823,#78824,#78825,#78826,
#78827,#78828,#78829,#78830,#78831,#78832,#78833,#78834,#78835,#78836,#78837,
#78838,#78839,#78840,#78841,#78842,#78843,#78844,#78845,#78846,#78847,#78848,
#78849,#78850,#78851,#78852,#78853,#78854,#78855,#78856,#78857,#78858,#78859,
#78860,#78861,#78862,#78863,#78864,#78865,#78866,#78867,#78868,#78869,#78870,
#78871,#78872,#78873,#78874,#78875,#78876,#78877,#78878,#78879,#78880,#78881,
#78882,#78883,#78884,#78885,#78886,#78887,#78888,#78889,#78890,#78891,#78892,
#78893,#78894,#78895,#78896,#78897,#78898,#78899,#78900,#78901,#78902,#78903,
#78904,#78905,#78906,#78907,#78908,#78909,#78910,#78911,#78912,#78913,#78914,
#78915,#78916,#78917,#78918,#78919,#78920,#78921,#78922,#78923,#78924,#78925,
#78926,#78927,#78928,#78929,#78930,#78931,#78932,#78933,#78934,#78935,#78936,
#78937,#78938,#78939,#78940,#78941,#78942,#78943,#78944,#78945,#78946,#78947,
#78948,#78949,#78950,#78951,#78952,#78953,#78954,#78955,#78956,#78957,#78958,
#78959),.UNSPECIFIED.,.F.,.F.,(4,2,2,2,2,2,2,2,2,2,2,2,2,2,2,2,2,2,2,2,
2,2,2,2,2,2,2,2,2,2,2,2,2,2,2,2,2,2,2,2,2,2,2,2,2,2,2,2,2,2,2,2,2,2,2,2,
2,2,2,2,2,2,2,2,2,2,2,2,2,2,2,2,2,2,2,2,2,2,2,2,2,2,2,2,2,2,2,2,2,2,4),
(0.921425937241738,0.935047588256698,0.940596973306458,0.944602639488585,
0.948827892202315,0.955543837834373,0.963625969364764,0.981492657083748,
1.00956823508816,1.01407697961797,1.01658874030863,1.01886211690919,1.02220611035665,
1.03200166121431,1.0506028430488,1.07733983428292,1.0846753778969,1.08902528628111,
1.09298389631013,1.09821502602709,1.11061271826728,1.13030873267281,1.15501536779979,
1.15979223001154,1.16238724385352,1.16463319329929,1.1677980888709,1.17614649239289,
1.19030271680065,1.22439648347554,1.2311842498732,1.23542395882675,1.23942267523241,
1.24492875803767,1.25942023585298,1.2858747359802,1.30265034347765,1.30657720259476,
1.30896627169807,1.31131558884073,1.31505481806986,1.32937156117902,1.34754896807697,
1.37142222633636,1.37770318371716,1.38184237853992,1.38590260595661,1.39176618685812,
1.40974047130409,1.42744414604826,1.44686941447829,1.45173788682739,1.45435223758731,
1.45659358839019,1.45972323955726,1.4678142219022,1.48127828301263,1.51682186482659,
1.52340141545502,1.52759940482106,1.53161972987439,1.53725736973447,1.55290470618805,
1.58464369795291,1.59544347409396,1.5989852568477,1.60106655126147,1.60343745002039,
1.60727905533835,1.62336514281784,1.65875083645647,1.6667510328446,1.67167856689287,
1.67560529463892,1.68013003452993,1.68835039969846,1.71359658097977,1.73932021414089,
1.7439548620375,1.7465194259263,1.74877365808267,1.75199791340774,1.7607997997127,
1.77624126834546,1.80922584955855,1.81562822009077,1.81979101679094,1.82351117961273,
1.82747030048524,1.83372067269811,1.84262518595721),.UNSPECIFIED.);
#1390=B_SPLINE_CURVE_WITH_KNOTS('',3,(#78960,#78961,#78962,#78963,#78964,
#78965,#78966,#78967,#78968,#78969,#78970,#78971,#78972,#78973,#78974,#78975,
#78976,#78977,#78978,#78979,#78980,#78981,#78982,#78983,#78984,#78985,#78986,
#78987,#78988,#78989,#78990,#78991,#78992,#78993,#78994,#78995,#78996,#78997,
#78998,#78999,#79000,#79001,#79002,#79003,#79004,#79005,#79006,#79007,#79008,
#79009,#79010,#79011,#79012,#79013,#79014,#79015,#79016,#79017,#79018,#79019,
#79020,#79021,#79022,#79023,#79024,#79025,#79026,#79027,#79028,#79029,#79030,
#79031,#79032,#79033,#79034,#79035,#79036,#79037,#79038,#79039,#79040,#79041,
#79042,#79043,#79044,#79045,#79046,#79047,#79048,#79049,#79050,#79051,#79052,
#79053,#79054,#79055,#79056,#79057,#79058,#79059,#79060,#79061,#79062,#79063,
#79064,#79065,#79066,#79067,#79068,#79069,#79070,#79071,#79072,#79073,#79074,
#79075,#79076,#79077,#79078,#79079,#79080,#79081,#79082,#79083,#79084,#79085,
#79086,#79087,#79088,#79089,#79090,#79091,#79092,#79093,#79094,#79095,#79096,
#79097,#79098,#79099,#79100,#79101,#79102,#79103,#79104,#79105,#79106,#79107,
#79108,#79109,#79110,#79111,#79112,#79113,#79114,#79115,#79116,#79117,#79118,
#79119,#79120,#79121,#79122,#79123,#79124,#79125,#79126,#79127,#79128,#79129,
#79130,#79131,#79132,#79133,#79134,#79135,#79136,#79137,#79138,#79139),
 .UNSPECIFIED.,.F.,.F.,(4,2,2,2,2,2,2,2,2,2,2,2,2,2,2,2,2,2,2,2,2,2,2,2,
2,2,2,2,2,2,2,2,2,2,2,2,2,2,2,2,2,2,2,2,2,2,2,2,2,2,2,2,2,2,2,2,2,2,2,2,
2,2,2,2,2,2,2,2,2,2,2,2,2,2,2,2,2,2,2,2,2,2,2,2,2,2,2,2,2,4),(0.921536811180233,
0.933102305825647,0.93829814936006,0.942244392776091,0.946526181407856,
0.953609051144324,0.975225115898132,1.00636807831321,1.01114863381681,1.01373509769844,
1.01596460421077,1.01909092016773,1.02723855626277,1.04087524380193,1.07610123448567,
1.08271456454244,1.08690191698484,1.09088854307265,1.09643757221683,1.11146515620285,
1.14020497718251,1.15427347636024,1.1580719595924,1.16042437349447,1.16277828739304,
1.16658391377995,1.18225107578502,1.21552044046769,1.22607044466416,1.23099793363849,
1.23490269947428,1.23937704554867,1.24742687727401,1.27418521079061,1.29851254812712,
1.30324974413601,1.30582693994069,1.30805858526487,1.31120167090468,1.31947285944942,
1.33344233575875,1.36796840418727,1.37468191474462,1.37888924183572,1.38286548417652,
1.38835180196037,1.40284329110401,1.42934183738193,1.4461111482636,1.45002365352312,
1.45240028330528,1.45473148007281,1.45842948352441,1.47233375164659,1.50578096121556,
1.51730256505604,1.52247392006901,1.52641636542503,1.53070854130175,1.53784399265397,
1.55985146052565,1.58490301413319,1.59346807218349,1.5967335364347,1.59898318655205,
1.60150084039512,1.60608435904497,1.61206071541396,1.62719168951254,1.65942690059912,
1.66643651562949,1.6707031660692,1.67465395077992,1.6799768566265,1.69317879305881,
1.7152293506433,1.73637636394252,1.74122156651758,1.74382140746739,1.74604740527106,
1.74914854381478,1.75711740949147,1.77028454270463,1.80305818921991,1.81057782345509,
1.81535723619063,1.81925261036891,1.82294237665107,1.82746270499088,1.84281035796432),
 .UNSPECIFIED.);
#1391=B_SPLINE_CURVE_WITH_KNOTS('',3,(#79144,#79145,#79146,#79147,#79148,
#79149,#79150,#79151,#79152,#79153,#79154,#79155,#79156,#79157,#79158,#79159,
#79160,#79161,#79162,#79163,#79164,#79165,#79166,#79167,#79168,#79169,#79170,
#79171,#79172,#79173,#79174,#79175,#79176,#79177,#79178,#79179,#79180,#79181,
#79182,#79183,#79184,#79185,#79186,#79187,#79188,#79189,#79190,#79191,#79192,
#79193,#79194,#79195,#79196,#79197,#79198,#79199,#79200,#79201,#79202,#79203,
#79204,#79205,#79206,#79207,#79208,#79209,#79210,#79211,#79212,#79213,#79214,
#79215,#79216,#79217,#79218,#79219,#79220,#79221,#79222,#79223,#79224,#79225,
#79226,#79227,#79228,#79229,#79230,#79231,#79232,#79233,#79234,#79235,#79236,
#79237,#79238,#79239,#79240,#79241,#79242,#79243,#79244,#79245,#79246,#79247,
#79248,#79249,#79250,#79251,#79252,#79253,#79254,#79255,#79256,#79257,#79258,
#79259,#79260,#79261,#79262,#79263,#79264,#79265,#79266,#79267,#79268,#79269,
#79270,#79271,#79272,#79273,#79274,#79275,#79276,#79277,#79278,#79279,#79280,
#79281,#79282,#79283,#79284,#79285,#79286,#79287,#79288,#79289,#79290,#79291,
#79292,#79293,#79294,#79295,#79296,#79297,#79298,#79299,#79300,#79301,#79302,
#79303,#79304,#79305,#79306,#79307,#79308,#79309,#79310,#79311,#79312,#79313,
#79314,#79315,#79316,#79317,#79318,#79319),.UNSPECIFIED.,.F.,.F.,(4,2,2,
2,2,2,2,2,2,2,2,2,2,2,2,2,2,2,2,2,2,2,2,2,2,2,2,2,2,2,2,2,2,2,2,2,2,2,2,
2,2,2,2,2,2,2,2,2,2,2,2,2,2,2,2,2,2,2,2,2,2,2,2,2,2,2,2,2,2,2,2,2,2,2,2,
2,2,2,2,2,2,2,2,2,2,2,2,4),(0.000151238077915164,0.00640778730925637,0.0241768538239276,
0.0443967716212503,0.0590010604211495,0.064521123245535,0.0685223682871949,
0.0727579144485144,0.0795236907992127,0.113759664550157,0.127834666857619,
0.136153776683449,0.139314846465747,0.141560478828986,0.144157909720819,
0.148945579093672,0.173563724311456,0.193328512494067,0.205751787152006,
0.210986928466309,0.214946285907897,0.219294769585089,0.226622332152765,
0.254155110444918,0.272168588386821,0.281791588150937,0.285115860822626,
0.287386046279402,0.289906115344984,0.294454548663721,0.32219268496662,
0.345957217577991,0.354028451919345,0.358524384173052,0.362454721541285,
0.367425137127329,0.378125390087704,0.411182228591696,0.426792792689984,
0.430609147265738,0.432974769041553,0.435059838106147,0.438622607759043,
0.449646953942215,0.481189474948909,0.496803212158547,0.502437544228046,
0.506457399582265,0.510656521033133,0.517241402763472,0.552728545424471,
0.566205989494761,0.574302306092487,0.577432697203122,0.579674215979176,
0.582288240746136,0.587155034969317,0.606549158563455,0.624289437562284,
0.642286709307247,0.64815265127695,0.652213355222013,0.656352072615005,
0.662630417998326,0.686469790386345,0.70461978232871,0.718970555238927,
0.722711782011883,0.725061547901424,0.72715827122535,0.730786062017507,
0.742569403168577,0.773388740911311,0.78886397038524,0.794483058935702,
0.798500239609215,0.802703698255418,0.809310815798728,0.844644609390707,
0.858192513107553,0.866315337534283,0.869449333425159,0.871691242973195,
0.874303083820267,0.879159761816994,0.89837576450849,0.921314446213366,
0.921425937241738),.UNSPECIFIED.);
#1392=B_SPLINE_CURVE_WITH_KNOTS('',3,(#79321,#79322,#79323,#79324),
 .UNSPECIFIED.,.F.,.F.,(4,4),(1.84281035796432,1.84292178567195),
 .UNSPECIFIED.);
#1393=B_SPLINE_CURVE_WITH_KNOTS('',3,(#79325,#79326,#79327,#79328,#79329,
#79330,#79331,#79332,#79333,#79334,#79335,#79336,#79337,#79338,#79339,#79340,
#79341,#79342,#79343,#79344,#79345,#79346,#79347,#79348,#79349,#79350,#79351,
#79352,#79353,#79354,#79355,#79356,#79357,#79358,#79359,#79360,#79361,#79362,
#79363,#79364,#79365,#79366,#79367,#79368,#79369,#79370,#79371,#79372,#79373,
#79374,#79375,#79376,#79377,#79378,#79379,#79380,#79381,#79382,#79383,#79384,
#79385,#79386,#79387,#79388,#79389,#79390,#79391,#79392,#79393,#79394,#79395,
#79396,#79397,#79398,#79399,#79400,#79401,#79402,#79403,#79404,#79405,#79406,
#79407,#79408,#79409,#79410,#79411,#79412,#79413,#79414,#79415,#79416,#79417,
#79418,#79419,#79420,#79421,#79422,#79423,#79424,#79425,#79426,#79427,#79428,
#79429,#79430,#79431,#79432,#79433,#79434,#79435,#79436,#79437,#79438,#79439,
#79440,#79441,#79442,#79443,#79444,#79445,#79446,#79447,#79448,#79449,#79450,
#79451,#79452,#79453,#79454,#79455,#79456,#79457,#79458,#79459,#79460,#79461,
#79462,#79463,#79464,#79465,#79466,#79467,#79468,#79469,#79470,#79471,#79472,
#79473,#79474,#79475,#79476,#79477,#79478,#79479,#79480,#79481,#79482,#79483,
#79484,#79485,#79486,#79487,#79488,#79489,#79490,#79491,#79492,#79493,#79494,
#79495,#79496,#79497,#79498),.UNSPECIFIED.,.F.,.F.,(4,2,2,2,2,2,2,2,2,2,
2,2,2,2,2,2,2,2,2,2,2,2,2,2,2,2,2,2,2,2,2,2,2,2,2,2,2,2,2,2,2,2,2,2,2,2,
2,2,2,2,2,2,2,2,2,2,2,2,2,2,2,2,2,2,2,2,2,2,2,2,2,2,2,2,2,2,2,2,2,2,2,2,
2,2,2,2,4),(9.51235209599495E-5,0.0254712809801649,0.036344157606092,0.0433755455167485,
0.0463376544890454,0.0485498550574796,0.051240824885174,0.0567007971363031,
0.0881640135096535,0.10302453771775,0.113405108105549,0.118304349458389,
0.122171220469519,0.126651569142186,0.134509915824775,0.168374895491002,
0.181248800535287,0.189104648942411,0.192189999063907,0.194414328269927,
0.197023845472009,0.201914280949435,0.224412910071305,0.255222317976374,
0.261936602416707,0.266143988178005,0.270119998901647,0.275605528739687,
0.289023923727613,0.32138809083701,0.333994082834365,0.337595368661739,
0.339906772155914,0.342308150281517,0.346337149371391,0.368338412255291,
0.390887833173197,0.404251145501673,0.409595843611872,0.413550050819569,
0.417808465770291,0.424776318516942,0.457346218286631,0.472286149789644,
0.480905779082826,0.484094930147705,0.486332944179747,0.488886250864103,
0.49351202097049,0.519250868680626,0.538470628798861,0.550679285488755,
0.555864135195988,0.559796109285014,0.564123666843638,0.571435193356866,
0.598732957987925,0.616943959622223,0.626615219183135,0.629932692322875,
0.632190900907919,0.634686592727932,0.639164003504284,0.667453160389326,
0.685248457400381,0.696900922679556,0.702002996726931,0.705924664579863,
0.71029350628798,0.717811876018003,0.752234438789054,0.765241567059644,
0.773148921190863,0.776241360224881,0.77846633646503,0.781071218632888,
0.785940392266249,0.805559282827188,0.828216195149896,0.842104568460713,
0.847516653777062,0.851480837172484,0.855713344411704,0.862553637736423,
0.89612254154228,0.917253116128758,0.921229644102655),.UNSPECIFIED.);
#1394=B_SPLINE_CURVE_WITH_KNOTS('',3,(#79504,#79505,#79506,#79507,#79508,
#79509,#79510,#79511,#79512,#79513,#79514,#79515,#79516,#79517,#79518,#79519,
#79520,#79521,#79522,#79523,#79524,#79525,#79526,#79527,#79528,#79529,#79530,
#79531,#79532,#79533,#79534,#79535,#79536,#79537,#79538,#79539,#79540,#79541,
#79542,#79543,#79544,#79545,#79546,#79547,#79548,#79549,#79550,#79551,#79552,
#79553,#79554,#79555,#79556,#79557,#79558,#79559,#79560,#79561,#79562,#79563,
#79564,#79565,#79566,#79567,#79568,#79569,#79570,#79571,#79572,#79573,#79574,
#79575,#79576,#79577,#79578,#79579,#79580,#79581,#79582,#79583,#79584,#79585,
#79586,#79587,#79588,#79589,#79590,#79591,#79592,#79593,#79594,#79595,#79596,
#79597,#79598,#79599,#79600,#79601,#79602,#79603,#79604,#79605,#79606,#79607,
#79608,#79609,#79610,#79611,#79612,#79613,#79614,#79615,#79616,#79617,#79618,
#79619,#79620,#79621,#79622,#79623,#79624,#79625,#79626,#79627,#79628,#79629,
#79630,#79631,#79632,#79633,#79634,#79635,#79636,#79637,#79638,#79639,#79640,
#79641,#79642,#79643,#79644,#79645,#79646,#79647,#79648,#79649,#79650,#79651,
#79652,#79653,#79654,#79655,#79656,#79657,#79658,#79659,#79660,#79661,#79662,
#79663,#79664,#79665,#79666,#79667,#79668,#79669,#79670,#79671,#79672,#79673,
#79674,#79675,#79676,#79677,#79678,#79679,#79680,#79681,#79682,#79683,#79684,
#79685,#79686,#79687),.UNSPECIFIED.,.F.,.F.,(4,2,2,2,2,2,2,2,2,2,2,2,2,
2,2,2,2,2,2,2,2,2,2,2,2,2,2,2,2,2,2,2,2,2,2,2,2,2,2,2,2,2,2,2,2,2,2,2,2,
2,2,2,2,2,2,2,2,2,2,2,2,2,2,2,2,2,2,2,2,2,2,2,2,2,2,2,2,2,2,2,2,2,2,2,2,
2,2,2,2,2,2,4),(0.921842322598426,0.921971004497343,0.953992808066859,0.95863137835825,
0.961196190559706,0.963450209066568,0.96667227576309,0.975452321063484,
0.990826999153283,1.02258444635569,1.02966656685149,1.03396661469429,1.03794294671248,
1.04329390430075,1.05654948664906,1.07872654003213,1.09963636127533,1.10449896000988,
1.10711284661048,1.10935544198543,1.11248945502758,1.12060776202534,1.13414219482962,
1.16954541820336,1.17614788821059,1.18035113388906,1.18436999604957,1.18999463742742,
1.20551365643492,1.23655745542615,1.24809404399398,1.25170122820025,1.25379448311335,
1.25614950189284,1.25991490605654,1.27463773786905,1.29250516226475,1.31626705750933,
1.32253758684407,1.32667515477448,1.33073766666332,1.33661152548057,1.35469749621604,
1.37258465769031,1.39173335279365,1.39658698975407,1.39919843186789,1.40144092021604,
1.40457695660832,1.4127109907312,1.42628742327495,1.46160319547748,1.46821889530715,
1.47242474818155,1.4764420752362,1.48205780680045,1.49749644282553,1.52813234737186,
1.54009096004661,1.54373725114703,1.54583768562363,1.54818391752498,1.55190670803212,
1.56596634234,1.60015381234387,1.61129708631472,1.61633952572813,1.62027689499638,
1.62472830561035,1.6325711421564,1.64252632257581,1.66957029060646,1.68563487863911,
1.68953089677225,1.69191363141661,1.69426928176339,1.69803771557473,1.71281034555871,
1.73063199953393,1.75438234934481,1.76065187104284,1.76478925975218,1.76885197036206,
1.7747268198483,1.79282492422776,1.8166379608318,1.824977963108,1.83309108917276,
1.83630120185999,1.83851390674685,1.84074373157238,1.84320277452714),
 .UNSPECIFIED.);
#1395=B_SPLINE_CURVE_WITH_KNOTS('',3,(#79688,#79689,#79690,#79691),
 .UNSPECIFIED.,.F.,.F.,(4,4),(0.000126975314923754,0.000151238077915164),
 .UNSPECIFIED.);
#1396=B_SPLINE_CURVE_WITH_KNOTS('',3,(#79693,#79694,#79695,#79696,#79697,
#79698,#79699,#79700,#79701,#79702,#79703,#79704,#79705,#79706,#79707,#79708,
#79709,#79710,#79711,#79712,#79713,#79714,#79715,#79716,#79717,#79718,#79719,
#79720,#79721,#79722,#79723,#79724,#79725,#79726,#79727,#79728,#79729,#79730,
#79731,#79732,#79733,#79734,#79735,#79736,#79737,#79738,#79739,#79740,#79741,
#79742,#79743,#79744,#79745,#79746,#79747,#79748,#79749,#79750,#79751,#79752,
#79753,#79754,#79755,#79756,#79757,#79758,#79759,#79760,#79761,#79762,#79763,
#79764,#79765,#79766,#79767,#79768,#79769,#79770,#79771,#79772,#79773,#79774,
#79775,#79776,#79777,#79778,#79779,#79780,#79781,#79782,#79783,#79784,#79785,
#79786,#79787,#79788,#79789,#79790,#79791,#79792,#79793,#79794,#79795,#79796,
#79797,#79798,#79799,#79800,#79801,#79802,#79803,#79804,#79805,#79806,#79807,
#79808,#79809,#79810,#79811,#79812,#79813,#79814,#79815,#79816,#79817,#79818,
#79819,#79820,#79821,#79822,#79823,#79824,#79825,#79826,#79827,#79828,#79829,
#79830,#79831,#79832,#79833,#79834,#79835,#79836,#79837,#79838,#79839,#79840,
#79841,#79842,#79843,#79844,#79845,#79846,#79847,#79848,#79849,#79850,#79851,
#79852,#79853,#79854,#79855,#79856,#79857,#79858,#79859,#79860,#79861,#79862,
#79863,#79864,#79865,#79866,#79867,#79868,#79869,#79870,#79871,#79872,#79873,
#79874,#79875,#79876,#79877,#79878),.UNSPECIFIED.,.F.,.F.,(4,2,2,2,2,2,
2,2,2,2,2,2,2,2,2,2,2,2,2,2,2,2,2,2,2,2,2,2,2,2,2,2,2,2,2,2,2,2,2,2,2,2,
2,2,2,2,2,2,2,2,2,2,2,2,2,2,2,2,2,2,2,2,2,2,2,2,2,2,2,2,2,2,2,2,2,2,2,2,
2,2,2,2,2,2,2,2,2,2,2,2,2,2,4),(0.921229644102655,0.921252861741337,0.923647958621843,
0.925963893240356,0.92958803755803,0.9424822474088,0.977059571664178,0.988600431906422,
0.993774773620674,0.997717424179817,1.00200779006674,1.00913525694689,1.03108540419854,
1.05601803235829,1.06472589268181,1.0680103578849,1.0702629688971,1.07277213983572,
1.07731506511373,1.08322095399415,1.09804365324033,1.13085739837009,1.13779700975506,
1.14204933806114,1.14600506734153,1.15136306540535,1.16483280765513,1.18772466977566,
1.20759536430365,1.21248386352344,1.21509268159662,1.2173166054511,1.22040173936432,
1.22825836083793,1.24113624670114,1.27500920657182,1.28286768889638,1.28734752976231,
1.29121360756154,1.29611137448384,1.3064872218076,1.32133792104234,1.35278193480356,
1.35823782508062,1.36092764899221,1.36313937728964,1.36610152882785,1.37313577565245,
1.38401722438189,1.41905708523396,1.4280787614883,1.43279225763882,1.43668544448536,
1.44132861139383,1.45026601369845,1.46221771666168,1.47991780114922,1.49960777676112,
1.50448173207187,1.50708739755177,1.50931178499273,1.51240179746173,1.52029366159329,
1.53326247170346,1.56751420358692,1.57508125479721,1.57950022734373,1.58341166315637,
1.58842308980116,1.59949579375397,1.61590354368184,1.64226795947809,1.64923120363644,
1.65198465555012,1.65423578332787,1.65674773842603,1.66130505856827,1.66723622154103,
1.68217083741537,1.71476876415928,1.72172914268572,1.72598528623175,1.72993883950468,
1.73528495096963,1.74866756738684,1.77128479313777,1.79315816394817,1.79717905604436,
1.79957825716694,1.80188984567116,1.80549507613821,1.81815989221302,1.84218579280452),
 .UNSPECIFIED.);
#1397=B_SPLINE_CURVE_WITH_KNOTS('',3,(#79879,#79880,#79881,#79882),
 .UNSPECIFIED.,.F.,.F.,(4,4),(8.31121291700962E-5,0.000212271119411096),
 .UNSPECIFIED.);
#1398=B_SPLINE_CURVE_WITH_KNOTS('',3,(#79887,#79888,#79889,#79890,#79891,
#79892,#79893,#79894,#79895,#79896,#79897,#79898,#79899,#79900,#79901,#79902,
#79903,#79904,#79905,#79906,#79907,#79908,#79909,#79910,#79911,#79912,#79913,
#79914,#79915,#79916,#79917,#79918,#79919,#79920,#79921,#79922,#79923,#79924,
#79925,#79926,#79927,#79928,#79929,#79930,#79931,#79932,#79933,#79934,#79935,
#79936,#79937,#79938,#79939,#79940,#79941,#79942,#79943,#79944,#79945,#79946,
#79947,#79948,#79949,#79950,#79951,#79952,#79953,#79954,#79955,#79956,#79957,
#79958,#79959,#79960,#79961,#79962,#79963,#79964,#79965,#79966,#79967,#79968,
#79969,#79970,#79971,#79972,#79973,#79974,#79975,#79976,#79977,#79978,#79979,
#79980,#79981,#79982,#79983,#79984,#79985,#79986,#79987,#79988,#79989,#79990,
#79991,#79992,#79993,#79994,#79995,#79996,#79997,#79998,#79999,#80000,#80001,
#80002,#80003,#80004,#80005,#80006,#80007,#80008,#80009,#80010,#80011,#80012,
#80013,#80014,#80015,#80016,#80017,#80018,#80019,#80020,#80021,#80022,#80023,
#80024,#80025,#80026,#80027,#80028,#80029,#80030,#80031,#80032,#80033,#80034,
#80035,#80036,#80037,#80038,#80039,#80040,#80041,#80042,#80043,#80044,#80045,
#80046,#80047,#80048,#80049,#80050,#80051,#80052,#80053,#80054,#80055,#80056,
#80057,#80058,#80059,#80060,#80061,#80062,#80063,#80064,#80065,#80066,#80067,
#80068),.UNSPECIFIED.,.F.,.F.,(4,2,2,2,2,2,2,2,2,2,2,2,2,2,2,2,2,2,2,2,
2,2,2,2,2,2,2,2,2,2,2,2,2,2,2,2,2,2,2,2,2,2,2,2,2,2,2,2,2,2,2,2,2,2,2,2,
2,2,2,2,2,2,2,2,2,2,2,2,2,2,2,2,2,2,2,2,2,2,2,2,2,2,2,2,2,2,2,2,2,2,4),
(0.000409495598106863,0.00411624641659977,0.00763961738565761,0.0112036564741097,
0.0151649190678298,0.0211020083759937,0.0401696307536014,0.0696775020094234,
0.0808615608811188,0.0842468300984096,0.0864683303915771,0.0888753657548912,
0.0929102841698461,0.1151298837162,0.13769433779516,0.151127845037877,0.15653232530443,
0.160545597077753,0.164885726680577,0.172045944542388,0.201674149848935,
0.217525111103473,0.226457858934173,0.229730217775301,0.232019891080921,
0.234623937612574,0.239519452166005,0.257980716661014,0.281866326541254,
0.295650904773997,0.30108708962904,0.305093059636614,0.309395012481321,
0.316411725077301,0.351641300955629,0.364817368041932,0.372806612421837,
0.375929395255939,0.378172261243137,0.380787642424671,0.385687728159702,
0.405590755672584,0.428461440360474,0.441926331415388,0.447288278283224,
0.451248924134294,0.455508397536511,0.46246369176431,0.497800596861752,
0.511045504275207,0.519049549901295,0.522156552013692,0.524388250971347,
0.527002496885108,0.531869713372902,0.551271791746638,0.569022418895147,
0.581147515764566,0.590189786786111,0.594875004103136,0.598799592790457,
0.603548366629588,0.612638933064306,0.647472553043876,0.663425292944995,
0.667264405827028,0.66963865230539,0.671724945080156,0.675284495131672,
0.686249434792894,0.717842019912523,0.73346494739358,0.73910226002657,0.743124524387538,
0.747326509768823,0.753916794824024,0.789411244238249,0.802900186259938,
0.811002065689626,0.814133937038144,0.816375819054558,0.818988612152688,
0.823851887188071,0.843188569044613,0.860438188133539,0.878909724832397,
0.884814292786726,0.888880771019699,0.893008252364856,0.899235153875353,
0.921842322598426),.UNSPECIFIED.);
#1399=B_SPLINE_CURVE_WITH_KNOTS('',3,(#80069,#80070,#80071,#80072,#80073,
#80074,#80075,#80076,#80077,#80078,#80079,#80080,#80081,#80082,#80083,#80084,
#80085,#80086,#80087,#80088,#80089,#80090,#80091,#80092,#80093,#80094,#80095,
#80096,#80097,#80098,#80099,#80100,#80101,#80102,#80103,#80104,#80105,#80106,
#80107,#80108,#80109,#80110,#80111,#80112,#80113,#80114,#80115,#80116,#80117,
#80118,#80119,#80120,#80121,#80122,#80123,#80124,#80125,#80126,#80127,#80128,
#80129,#80130,#80131,#80132,#80133,#80134,#80135,#80136,#80137,#80138,#80139,
#80140,#80141,#80142,#80143,#80144,#80145,#80146,#80147,#80148,#80149,#80150,
#80151,#80152,#80153,#80154,#80155,#80156,#80157,#80158,#80159,#80160,#80161,
#80162,#80163,#80164,#80165,#80166,#80167,#80168,#80169,#80170,#80171,#80172,
#80173,#80174,#80175,#80176,#80177,#80178,#80179,#80180,#80181,#80182,#80183,
#80184,#80185,#80186,#80187,#80188,#80189,#80190,#80191,#80192,#80193,#80194,
#80195,#80196,#80197,#80198,#80199,#80200,#80201,#80202,#80203,#80204,#80205,
#80206,#80207,#80208,#80209,#80210,#80211,#80212,#80213,#80214,#80215,#80216,
#80217,#80218,#80219,#80220,#80221,#80222,#80223,#80224,#80225,#80226,#80227,
#80228,#80229,#80230,#80231,#80232,#80233,#80234,#80235,#80236,#80237,#80238,
#80239,#80240,#80241,#80242,#80243,#80244,#80245,#80246,#80247,#80248,#80249,
#80250,#80251,#80252),.UNSPECIFIED.,.F.,.F.,(4,2,2,2,2,2,2,2,2,2,2,2,2,
2,2,2,2,2,2,2,2,2,2,2,2,2,2,2,2,2,2,2,2,2,2,2,2,2,2,2,2,2,2,2,2,2,2,2,2,
2,2,2,2,2,2,2,2,2,2,2,2,2,2,2,2,2,2,2,2,2,2,2,2,2,2,2,2,2,2,2,2,2,2,2,2,
2,2,2,2,2,2,4),(0.000212271119411096,0.0184268769916361,0.0236198335754554,
0.0275033491686757,0.0314545942917832,0.0357215569034563,0.0427312808188781,
0.0770023918457398,0.0907424764220856,0.0989289238335929,0.102060439672156,
0.10429061668719,0.106874158474456,0.111640871476838,0.136168695473555,
0.156036812196146,0.168486747688842,0.173706794257779,0.17764386491016,
0.181956000702848,0.189188684272954,0.218973749821132,0.235507685860731,
0.244662825852073,0.247919720916535,0.250168463491246,0.252691371725201,
0.25729738996751,0.289759207007853,0.304846801269719,0.315331942567293,
0.320249118054466,0.324118070074919,0.328587599438841,0.336391443921904,
0.370329630345493,0.383220768259483,0.391083377394536,0.394169727893822,
0.396393713088988,0.399000675774037,0.403883778725287,0.423689832784035,
0.44151716200985,0.45336605122852,0.462248390380849,0.466880445984012,0.470772425874221,
0.475494243934464,0.484563724267043,0.522621234162304,0.535893049872872,
0.539544970708945,0.541866135222855,0.544254344338416,0.548219381464529,
0.567633765934114,0.598862226160437,0.608110550277805,0.612813124860416,
0.616708997101244,0.621369365724602,0.630109692230653,0.641888483931618,
0.659838638339606,0.679589654221265,0.684470598521228,0.687079480259172,
0.689309007572819,0.692409143629907,0.700341149783576,0.713410856060205,
0.748164606225848,0.755388263697132,0.759701958755032,0.763645254168221,
0.768881291304163,0.781417411278475,0.8015094835942,0.825737252797056,0.830476980431821,
0.833054615275502,0.835275731146635,0.838393724790873,0.846560243905356,
0.860258557245317,0.895607680430056,0.90222007170262,0.906392735315957,
0.9103542814628,0.915848105643038,0.92152398119564),.UNSPECIFIED.);
#1400=B_SPLINE_CURVE_WITH_KNOTS('',3,(#80258,#80259,#80260,#80261,#80262,
#80263,#80264,#80265,#80266,#80267,#80268,#80269,#80270,#80271,#80272,#80273,
#80274,#80275,#80276,#80277,#80278,#80279,#80280,#80281,#80282,#80283,#80284,
#80285,#80286,#80287,#80288,#80289,#80290,#80291,#80292,#80293,#80294,#80295,
#80296,#80297,#80298,#80299,#80300,#80301,#80302,#80303,#80304,#80305,#80306,
#80307,#80308,#80309,#80310,#80311,#80312,#80313,#80314,#80315,#80316,#80317,
#80318,#80319,#80320,#80321,#80322,#80323,#80324,#80325,#80326,#80327,#80328,
#80329,#80330,#80331,#80332,#80333,#80334,#80335,#80336,#80337,#80338,#80339,
#80340,#80341,#80342,#80343,#80344,#80345,#80346,#80347,#80348,#80349,#80350,
#80351,#80352,#80353,#80354,#80355,#80356,#80357,#80358,#80359,#80360,#80361,
#80362,#80363,#80364,#80365,#80366,#80367,#80368,#80369,#80370,#80371,#80372,
#80373,#80374,#80375,#80376,#80377,#80378,#80379,#80380,#80381,#80382,#80383,
#80384,#80385,#80386,#80387),.UNSPECIFIED.,.F.,.F.,(4,2,2,2,2,2,2,2,2,2,
2,2,2,2,2,2,2,2,2,2,2,2,2,2,2,2,2,2,2,2,2,2,2,2,2,2,2,2,2,2,2,2,2,2,2,2,
2,2,2,2,2,2,2,2,2,2,2,2,2,2,2,2,2,2,4),(-0.589266859322642,-0.583170718802222,
-0.579282628579395,-0.576924566074347,-0.57452032528388,-0.570412233191057,
-0.565139040401791,-0.55198759141902,-0.528926529180157,-0.522537395514901,
-0.518409672101166,-0.51436475306196,-0.50843254142529,-0.48635380224999,
-0.46600745613857,-0.461886461509982,-0.459478543697714,-0.457114571232146,
-0.453217738090236,-0.435024959395931,-0.411351068044394,-0.405015281957827,
-0.400894937262368,-0.396837082845925,-0.390846789372038,-0.369237742364032,
-0.348468253784916,-0.344366071710034,-0.341963344537253,-0.339618433922597,
-0.335756960468933,-0.330900902638634,-0.319540174427223,-0.292928533939326,
-0.286899037196489,-0.28325680050945,-0.279254808303444,-0.27347579982458,
-0.251111995620155,-0.230726430683364,-0.226613577869565,-0.224214201521056,
-0.221850241821066,-0.217964566466566,-0.213079026155885,-0.201639775208353,
-0.175312646047459,-0.169228113439053,-0.165548630702281,-0.161499412822675,
-0.155632464107968,-0.132699692598671,-0.113296622916967,-0.109066948012962,
-0.106625296331815,-0.104230015179095,-0.100293912091128,-0.0834054084904788,
-0.0590223232485894,-0.0528309458458233,-0.0487145198233409,-0.0445880120408051,
-0.0383459587393695,-0.0308954481058898,-5.3213449454262E-5),
 .UNSPECIFIED.);
#1401=B_SPLINE_CURVE_WITH_KNOTS('',3,(#80390,#80391,#80392,#80393,#80394,
#80395,#80396,#80397,#80398,#80399,#80400,#80401,#80402,#80403,#80404,#80405,
#80406,#80407,#80408,#80409,#80410,#80411,#80412,#80413,#80414,#80415,#80416,
#80417,#80418,#80419,#80420,#80421,#80422,#80423,#80424,#80425,#80426,#80427,
#80428,#80429,#80430,#80431,#80432,#80433,#80434,#80435,#80436,#80437,#80438,
#80439,#80440,#80441,#80442,#80443,#80444,#80445,#80446,#80447,#80448,#80449,
#80450,#80451,#80452,#80453,#80454,#80455,#80456,#80457,#80458,#80459,#80460,
#80461,#80462,#80463,#80464,#80465,#80466,#80467,#80468,#80469,#80470,#80471,
#80472,#80473,#80474,#80475,#80476,#80477,#80478,#80479,#80480,#80481,#80482,
#80483,#80484,#80485),.UNSPECIFIED.,.F.,.F.,(4,2,2,2,2,2,2,2,2,2,2,2,2,
2,2,2,2,2,2,2,2,2,2,2,2,2,2,2,2,2,2,2,2,2,2,2,2,2,2,2,2,2,2,2,2,2,2,4),
(-4.19276052999992,-4.18994930679582,-4.18594508777967,-4.16986863132682,
-4.15061368004302,-4.14354516891226,-4.13898217474332,-4.13444468871921,
-4.12758398506696,-4.10080057567627,-4.08183773106484,-4.07790888789601,
-4.07551930049204,-4.07316304090163,-4.06917333893694,-4.04805153823428,
-4.02702609715168,-4.0213060269127,-4.01739784825908,-4.01341394757536,
-4.0072877679487,-3.98038949311294,-3.9627452339993,-3.9591534892204,-3.95690556319255,
-3.95448562980752,-3.95031807462353,-3.93056727411159,-3.90816359210308,
-3.90200162654388,-3.89787209907124,-3.89370785084629,-3.88734825741719,
-3.86478161281914,-3.8519079261705,-3.84668583278294,-3.84259510490349,
-3.84015915922247,-3.83772960223034,-3.83360376691708,-3.81293046552367,
-3.79818007879994,-3.79123456879836,-3.78530836193634,-3.78123107649018,
-3.77753256329089,-3.77142850268503,-3.74878577142885),.UNSPECIFIED.);
#1402=B_SPLINE_CURVE_WITH_KNOTS('',3,(#80490,#80491,#80492,#80493,#80494,
#80495,#80496,#80497,#80498,#80499,#80500,#80501,#80502,#80503,#80504,#80505,
#80506,#80507,#80508,#80509,#80510,#80511,#80512,#80513,#80514,#80515,#80516,
#80517,#80518,#80519,#80520,#80521,#80522,#80523,#80524,#80525,#80526,#80527,
#80528,#80529,#80530,#80531,#80532,#80533,#80534,#80535,#80536,#80537,#80538,
#80539,#80540,#80541,#80542,#80543,#80544,#80545,#80546,#80547,#80548,#80549,
#80550,#80551,#80552,#80553,#80554,#80555,#80556,#80557,#80558,#80559,#80560,
#80561,#80562,#80563,#80564,#80565,#80566,#80567,#80568,#80569,#80570,#80571,
#80572,#80573,#80574,#80575,#80576,#80577,#80578,#80579,#80580,#80581,#80582,
#80583,#80584,#80585,#80586,#80587,#80588,#80589,#80590,#80591,#80592,#80593,
#80594,#80595,#80596,#80597,#80598,#80599,#80600,#80601,#80602,#80603,#80604,
#80605,#80606,#80607,#80608,#80609,#80610,#80611,#80612,#80613,#80614,#80615,
#80616,#80617,#80618,#80619,#80620,#80621,#80622,#80623,#80624,#80625,#80626,
#80627,#80628,#80629,#80630,#80631,#80632,#80633,#80634,#80635,#80636,#80637,
#80638,#80639,#80640,#80641,#80642,#80643,#80644,#80645,#80646,#80647,#80648,
#80649,#80650,#80651,#80652,#80653,#80654,#80655,#80656,#80657),
 .UNSPECIFIED.,.F.,.F.,(4,2,2,2,2,2,2,2,2,2,2,2,2,2,2,2,2,2,2,2,2,2,2,2,
2,2,2,2,2,2,2,2,2,2,2,2,2,2,2,2,2,2,2,2,2,2,2,2,2,2,2,2,2,2,2,2,2,2,2,2,
2,2,2,2,2,2,2,2,2,2,2,2,2,2,2,2,2,2,2,2,2,2,2,4),(-1.33107822423028,-1.3050320018944,
-1.29352334269686,-1.28862725477286,-1.28473927003311,-1.28238102649599,
-1.27997764655231,-1.27586998909895,-1.25527317844522,-1.24040299895147,
-1.23344479071331,-1.22752376544648,-1.22348303462989,-1.21935697758132,
-1.21296521024282,-1.19000648247202,-1.17679209785019,-1.17150596072924,
-1.167391345638,-1.16498651647294,-1.16262929642075,-1.15874699505247,-1.13586594724723,
-1.12214752262523,-1.11548487203495,-1.10974961776421,-1.10574044463247,
-1.10156804175507,-1.09492964179377,-1.06354709468678,-1.05596461857385,
-1.0506361941307,-1.04799435732233,-1.0457517447292,-1.0425264939916,-1.03300562585385,
-1.01250018669264,-1.00745771142861,-0.99629042329858,-0.991266084053232,
-0.987344994471621,-0.982927031662876,-0.974978443716631,-0.945943537066251,
-0.935095497126092,-0.93162620033597,-0.929369219910836,-0.926848823166088,
-0.92216173012559,-0.915839981154276,-0.896890053774975,-0.879939422309999,
-0.874368673094545,-0.870385474534947,-0.866163061257192,-0.859262813163703,
-0.836215843092881,-0.817929596279315,-0.814260367344161,-0.812172704452408,
-0.809788344228874,-0.80577706139847,-0.800671402384763,-0.7882705433584,
-0.7639355910793,-0.757650361450218,-0.753542860816598,-0.749483832103811,
-0.743466064666463,-0.720266428187892,-0.701448604858594,-0.697198526567655,
-0.69476553986039,-0.692431470813763,-0.688662429614172,-0.683967144826868,
-0.673267357442596,-0.64537574701729,-0.639534887130647,-0.635549041738243,
-0.631415436602443,-0.624978196448166,-0.60603202519002,-0.589266859322642),
 .UNSPECIFIED.);
#1403=B_SPLINE_CURVE_WITH_KNOTS('',3,(#80658,#80659,#80660,#80661,#80662,
#80663,#80664,#80665,#80666,#80667,#80668,#80669,#80670,#80671,#80672,#80673,
#80674,#80675,#80676,#80677,#80678,#80679,#80680,#80681,#80682,#80683,#80684,
#80685,#80686,#80687,#80688,#80689,#80690,#80691,#80692,#80693,#80694,#80695,
#80696,#80697,#80698,#80699,#80700,#80701,#80702,#80703,#80704,#80705,#80706,
#80707,#80708,#80709,#80710,#80711,#80712,#80713,#80714,#80715,#80716,#80717,
#80718,#80719,#80720,#80721,#80722,#80723,#80724,#80725,#80726,#80727,#80728,
#80729,#80730,#80731,#80732,#80733,#80734,#80735,#80736,#80737,#80738,#80739,
#80740,#80741,#80742,#80743,#80744,#80745,#80746,#80747,#80748,#80749,#80750,
#80751,#80752,#80753,#80754,#80755,#80756,#80757,#80758,#80759,#80760,#80761,
#80762,#80763,#80764,#80765,#80766,#80767,#80768,#80769,#80770,#80771,#80772,
#80773,#80774,#80775,#80776,#80777,#80778,#80779,#80780,#80781,#80782,#80783,
#80784,#80785,#80786,#80787,#80788,#80789,#80790,#80791,#80792,#80793,#80794,
#80795,#80796,#80797,#80798,#80799,#80800,#80801,#80802,#80803,#80804,#80805,
#80806,#80807,#80808,#80809,#80810,#80811,#80812,#80813,#80814,#80815,#80816,
#80817,#80818,#80819,#80820,#80821,#80822,#80823,#80824,#80825,#80826,#80827,
#80828,#80829,#80830,#80831),.UNSPECIFIED.,.F.,.F.,(4,2,2,2,2,2,2,2,2,2,
2,2,2,2,2,2,2,2,2,2,2,2,2,2,2,2,2,2,2,2,2,2,2,2,2,2,2,2,2,2,2,2,2,2,2,2,
2,2,2,2,2,2,2,2,2,2,2,2,2,2,2,2,2,2,2,2,2,2,2,2,2,2,2,2,2,2,2,2,2,2,2,2,
2,2,2,2,4),(-3.74878577142885,-3.74513268586829,-3.73368516973695,-3.72879060302111,
-3.72489574378074,-3.72252099603933,-3.72010128721677,-3.71593252466715,
-3.6962709835695,-3.6808830932062,-3.67379693917892,-3.66779525735489,-3.66373675479838,
-3.65962168377017,-3.65330880991156,-3.62900949669526,-3.61108907877409,
-3.60719463421898,-3.60483402410306,-3.60241642523591,-3.59828561734588,
-3.5779777972868,-3.55623228815388,-3.55011924059378,-3.54602175634493,
-3.54189259994483,-3.53560409840515,-3.51121683643263,-3.49369077938276,
-3.48974210793145,-3.4873584592989,-3.4849397112567,-3.48081012651282,-3.46045026784276,
-3.4386217365211,-3.43259050123225,-3.42851016267578,-3.4243693682092,-3.41800433983943,
-3.39433840732508,-3.3756601741496,-3.37194792679964,-3.36961426406217,
-3.36714145326678,-3.36273622494596,-3.34552910478588,-3.32880988610618,
-3.32140918127248,-3.31520775321776,-3.31109996549892,-3.30699802673909,
-3.30082904944937,-3.27525597638523,-3.2634835716586,-3.25851721587624,
-3.25458366732408,-3.2522074408767,-3.24979151647253,-3.24566953670843,
-3.22513373692306,-3.21024022498641,-3.20326485573878,-3.19732507142642,
-3.19326147317916,-3.18959120945997,-3.18357432911096,-3.15683174931789,
-3.14563307576243,-3.14080486450673,-3.13695218847295,-3.13459080225662,
-3.13215408713309,-3.12793120403522,-3.10855641959898,-3.09304243394775,
-3.08591678787807,-3.07988378275844,-3.07580424071015,-3.0716659719809,
-3.06530866194832,-3.04157478379966,-3.0233397238207,-3.01943395513676,
-3.01706231224811,-3.0146391799905,-3.01048184697966,-3.00705510852159),
 .UNSPECIFIED.);
#1404=B_SPLINE_CURVE_WITH_KNOTS('',3,(#80836,#80837,#80838,#80839,#80840,
#80841,#80842,#80843,#80844,#80845,#80846,#80847,#80848,#80849,#80850,#80851,
#80852,#80853,#80854,#80855,#80856,#80857,#80858,#80859,#80860,#80861,#80862,
#80863,#80864,#80865,#80866,#80867,#80868,#80869,#80870,#80871,#80872,#80873,
#80874,#80875,#80876,#80877,#80878,#80879,#80880,#80881,#80882,#80883,#80884,
#80885,#80886,#80887,#80888,#80889,#80890,#80891,#80892,#80893,#80894,#80895,
#80896,#80897,#80898,#80899,#80900,#80901,#80902,#80903,#80904,#80905,#80906,
#80907,#80908,#80909,#80910,#80911,#80912,#80913,#80914,#80915,#80916,#80917,
#80918,#80919,#80920,#80921,#80922,#80923,#80924,#80925,#80926,#80927,#80928,
#80929,#80930,#80931,#80932,#80933,#80934,#80935,#80936,#80937,#80938,#80939,
#80940,#80941,#80942,#80943,#80944,#80945,#80946,#80947,#80948,#80949,#80950,
#80951,#80952,#80953,#80954,#80955,#80956,#80957,#80958,#80959,#80960,#80961,
#80962,#80963,#80964,#80965,#80966,#80967,#80968,#80969,#80970,#80971,#80972,
#80973,#80974,#80975,#80976,#80977,#80978,#80979,#80980,#80981,#80982,#80983,
#80984,#80985,#80986,#80987,#80988,#80989,#80990,#80991,#80992,#80993,#80994,
#80995,#80996,#80997,#80998,#80999),.UNSPECIFIED.,.F.,.F.,(4,2,2,2,2,2,
2,2,2,2,2,2,2,2,2,2,2,2,2,2,2,2,2,2,2,2,2,2,2,2,2,2,2,2,2,2,2,2,2,2,2,2,
2,2,2,2,2,2,2,2,2,2,2,2,2,2,2,2,2,2,2,2,2,2,2,2,2,2,2,2,2,2,2,2,2,2,2,2,
2,2,2,4),(-2.07270848450232,-2.05637947900051,-2.05041870419527,-2.04637147445068,
-2.04225505343102,-2.03591271074969,-2.01900120304341,-1.99397215540331,
-1.99006327819747,-1.98770094498518,-1.98530267068136,-1.98121909476245,
-1.9602542642696,-1.93879416667414,-1.93285129288563,-1.9288071244785,-1.92468663844824,
-1.91832282391021,-1.89492544567431,-1.88197921092116,-1.87675187753393,
-1.8726711616138,-1.87027351041234,-1.86791062294112,-1.8639991628537,-1.84138088300711,
-1.82231447415694,-1.8158623812433,-1.81172544622901,-1.80774035593035,
-1.80190771595934,-1.77396521320056,-1.76329097847408,-1.75860209243932,
-1.75483715834937,-1.75250358932328,-1.75006987929346,-1.74581338271324,
-1.72667238834097,-1.71104858767693,-1.70390826063274,-1.69787418030314,
-1.6938137410089,-1.68971226005504,-1.68345198973634,-1.65885125465335,
-1.64142704406966,-1.63747153795965,-1.635099585313,-1.63271141137436,-1.62867733838942,
-1.60716657590448,-1.58643072462178,-1.58036082221973,-1.57629391359855,
-1.57219943018413,-1.5659776091017,-1.54101187658049,-1.52382727082877,
-1.51989520821546,-1.51752802383727,-1.51513466295542,-1.5110755888295,
-1.48981970540655,-1.46859311414981,-1.46265374384937,-1.45860994192361,
-1.45448823171113,-1.44811913016952,-1.4308368298893,-1.40617903421335,
-1.40229525404027,-1.39993784924348,-1.39753348908643,-1.39342103817434,
-1.37293331858767,-1.35070763700637,-1.34491619039688,-1.34089785200684,
-1.33723427328462,-1.33114995542605,-1.33107822423028),.UNSPECIFIED.);
#1405=B_SPLINE_CURVE_WITH_KNOTS('',3,(#81000,#81001,#81002,#81003,#81004,
#81005,#81006,#81007,#81008,#81009,#81010,#81011,#81012,#81013,#81014,#81015,
#81016,#81017,#81018,#81019,#81020,#81021,#81022,#81023,#81024,#81025,#81026,
#81027,#81028,#81029,#81030,#81031,#81032,#81033,#81034,#81035,#81036,#81037,
#81038,#81039,#81040,#81041,#81042,#81043,#81044,#81045,#81046,#81047,#81048,
#81049,#81050,#81051,#81052,#81053,#81054,#81055,#81056,#81057,#81058,#81059,
#81060,#81061,#81062,#81063,#81064,#81065,#81066,#81067,#81068,#81069,#81070,
#81071,#81072,#81073,#81074,#81075,#81076,#81077,#81078,#81079,#81080,#81081,
#81082,#81083,#81084,#81085,#81086,#81087,#81088,#81089,#81090,#81091,#81092,
#81093,#81094,#81095,#81096,#81097,#81098,#81099,#81100,#81101,#81102,#81103,
#81104,#81105,#81106,#81107,#81108,#81109,#81110,#81111,#81112,#81113,#81114,
#81115,#81116,#81117,#81118,#81119,#81120,#81121,#81122,#81123,#81124,#81125,
#81126,#81127,#81128,#81129,#81130,#81131,#81132,#81133,#81134,#81135,#81136,
#81137,#81138,#81139,#81140,#81141,#81142,#81143,#81144,#81145,#81146,#81147,
#81148,#81149,#81150,#81151,#81152,#81153,#81154,#81155,#81156,#81157,#81158,
#81159,#81160,#81161,#81162,#81163,#81164,#81165),.UNSPECIFIED.,.F.,.F.,
(4,2,2,2,2,2,2,2,2,2,2,2,2,2,2,2,2,2,2,2,2,2,2,2,2,2,2,2,2,2,2,2,2,2,2,
2,2,2,2,2,2,2,2,2,2,2,2,2,2,2,2,2,2,2,2,2,2,2,2,2,2,2,2,2,2,2,2,2,2,2,2,
2,2,2,2,2,2,2,2,2,2,2,4),(-3.00705510852159,-2.99066778701684,-2.97535706723338,
-2.96828011428466,-2.96227735705098,-2.95820333716234,-2.9540589908238,
-2.9476677608138,-2.92440443875771,-2.90605684392387,-2.90199760030823,
-2.89959460569648,-2.89749579459065,-2.893812614373,-2.87538609653752,-2.85857897514339,
-2.85115740883379,-2.84494223005598,-2.84082979221944,-2.83672630758988,
-2.83056066040117,-2.80495584792262,-2.79320589740186,-2.78824406211796,
-2.78431261076756,-2.7819355940785,-2.77951792592766,-2.77538828798524,
-2.75504082516254,-2.74003446454397,-2.73303124844353,-2.727074172347,-2.72300772256983,
-2.71885246721819,-2.71240459472735,-2.69054132386259,-2.67067293183992,
-2.66673775545666,-2.66435999039269,-2.66194316037602,-2.65781774004939,
-2.63734685283338,-2.61547407786365,-2.60950158177183,-2.60543244923887,
-2.60128067696156,-2.59485153613769,-2.57229696340073,-2.55884039432496,
-2.55349409043209,-2.54934006442613,-2.54691740584065,-2.54454476056624,
-2.540635024459,-2.51789603891595,-2.49890838366919,-2.49244803036325,-2.48829042305874,
-2.48427283417218,-2.47836517267547,-2.45081600945923,-2.43997171718694,
-2.43523173627998,-2.4314315041655,-2.42908066210213,-2.42663059159411,
-2.42234272789024,-2.40333497306155,-2.38765371948162,-2.38048792560325,
-2.37442983460341,-2.3703454847996,-2.36621179171921,-2.35988125592821,
-2.33581952172769,-2.31772508169142,-2.31388477411611,-2.31152598528055,
-2.30908621145489,-2.30484908733473,-2.28666045454533,-2.27038572531952,
-2.26522078838353),.UNSPECIFIED.);
#1406=B_SPLINE_CURVE_WITH_KNOTS('',3,(#81171,#81172,#81173,#81174,#81175,
#81176,#81177,#81178,#81179,#81180,#81181,#81182,#81183,#81184,#81185,#81186,
#81187,#81188,#81189,#81190,#81191,#81192,#81193,#81194,#81195,#81196,#81197,
#81198,#81199,#81200,#81201,#81202,#81203,#81204,#81205,#81206,#81207,#81208,
#81209,#81210,#81211,#81212,#81213,#81214,#81215,#81216,#81217,#81218,#81219,
#81220,#81221,#81222,#81223,#81224,#81225,#81226,#81227,#81228,#81229,#81230,
#81231,#81232,#81233,#81234,#81235,#81236,#81237,#81238,#81239,#81240,#81241,
#81242,#81243,#81244,#81245,#81246,#81247,#81248,#81249,#81250,#81251,#81252,
#81253,#81254,#81255,#81256,#81257,#81258,#81259,#81260,#81261,#81262,#81263,
#81264,#81265,#81266,#81267,#81268,#81269,#81270,#81271,#81272,#81273,#81274,
#81275,#81276,#81277,#81278,#81279,#81280,#81281,#81282,#81283,#81284,#81285,
#81286,#81287,#81288,#81289,#81290,#81291,#81292,#81293,#81294,#81295,#81296,
#81297,#81298,#81299,#81300,#81301,#81302,#81303,#81304,#81305,#81306,#81307,
#81308,#81309,#81310,#81311,#81312,#81313,#81314,#81315,#81316,#81317,#81318,
#81319,#81320),.UNSPECIFIED.,.F.,.F.,(4,2,2,2,2,2,2,2,2,2,2,2,2,2,2,2,2,
2,2,2,2,2,2,2,2,2,2,2,2,2,2,2,2,2,2,2,2,2,2,2,2,2,2,2,2,2,2,2,2,2,2,2,2,
2,2,2,2,2,2,2,2,2,2,2,2,2,2,2,2,2,2,2,2,2,4),(-0.702969042438947,-0.701710412156898,
-0.699304623373738,-0.696946789994431,-0.693063925851947,-0.675881103467728,
-0.650796750698558,-0.644587498125185,-0.640494108134618,-0.636422922864456,
-0.630336176978641,-0.60886710145751,-0.58820624356317,-0.584098319843403,
-0.581694293400333,-0.579334819354786,-0.575444035329181,-0.557324263373413,
-0.533436234334152,-0.527108439139577,-0.522993158497826,-0.518941020346384,
-0.512961586389197,-0.491995501255123,-0.470471222025247,-0.466433132016482,
-0.464043431903924,-0.461670750216529,-0.457715418868478,-0.443561735531553,
-0.415153030706521,-0.409143632244394,-0.405491093668681,-0.401458881544609,
-0.395593521140241,-0.374220510307328,-0.352888789319575,-0.348831777321994,
-0.346438183941091,-0.344069178654129,-0.340131772873462,-0.322381201113179,
-0.298148375546142,-0.291850957097087,-0.287741225879504,-0.283684262644293,
-0.277677933974262,-0.256200256198579,-0.235353036769286,-0.231255926029211,
-0.228854042713106,-0.226492452653876,-0.22259162930125,-0.204814033399233,
-0.18052728933845,-0.174234695293368,-0.17012577339749,-0.166067910415485,
-0.160056974156436,-0.138653700615305,-0.117730904718132,-0.113638918266303,
-0.111238046138738,-0.108875434001243,-0.104969789486363,-0.100045096670016,
-0.0884202357153979,-0.0625486134681136,-0.0564319505365755,-0.0523550865526347,
-0.048266814175015,-0.0420873623547596,-0.0347113065829079,-0.0181409958602746,
-1.00000007552392E-6),.UNSPECIFIED.);
#1407=B_SPLINE_CURVE_WITH_KNOTS('',3,(#81321,#81322,#81323,#81324,#81325,
#81326,#81327,#81328,#81329,#81330,#81331,#81332,#81333,#81334,#81335,#81336,
#81337,#81338),.UNSPECIFIED.,.F.,.F.,(4,2,2,2,2,2,2,2,4),(-2.1117112384367,
-2.10803374113042,-2.10593836275868,-2.10373839514592,-2.10054077715998,
-2.09188679008812,-2.08281374733337,-2.07698764942234,-2.07270848450232),
 .UNSPECIFIED.);
#1408=B_SPLINE_CURVE_WITH_KNOTS('',3,(#81339,#81340,#81341,#81342,#81343,
#81344,#81345,#81346,#81347,#81348,#81349,#81350,#81351,#81352,#81353,#81354,
#81355,#81356,#81357,#81358,#81359,#81360,#81361,#81362,#81363,#81364,#81365,
#81366,#81367,#81368,#81369,#81370,#81371,#81372,#81373,#81374,#81375,#81376,
#81377,#81378,#81379,#81380,#81381,#81382,#81383,#81384,#81385,#81386,#81387,
#81388,#81389,#81390,#81391,#81392,#81393,#81394,#81395,#81396,#81397,#81398,
#81399,#81400,#81401,#81402,#81403,#81404,#81405,#81406,#81407,#81408,#81409,
#81410,#81411,#81412,#81413,#81414,#81415,#81416,#81417,#81418,#81419,#81420,
#81421,#81422,#81423,#81424,#81425,#81426,#81427,#81428,#81429,#81430,#81431,
#81432,#81433,#81434,#81435,#81436,#81437,#81438,#81439,#81440,#81441,#81442,
#81443,#81444,#81445,#81446,#81447,#81448,#81449,#81450,#81451,#81452,#81453,
#81454,#81455,#81456,#81457,#81458,#81459,#81460,#81461,#81462,#81463,#81464,
#81465,#81466,#81467,#81468,#81469,#81470,#81471,#81472,#81473,#81474,#81475,
#81476,#81477,#81478,#81479,#81480,#81481,#81482,#81483,#81484,#81485,#81486,
#81487,#81488,#81489,#81490,#81491,#81492,#81493,#81494,#81495,#81496,#81497,
#81498,#81499,#81500,#81501,#81502),.UNSPECIFIED.,.F.,.F.,(4,2,2,2,2,2,
2,2,2,2,2,2,2,2,2,2,2,2,2,2,2,2,2,2,2,2,2,2,2,2,2,2,2,2,2,2,2,2,2,2,2,2,
2,2,2,2,2,2,2,2,2,2,2,2,2,2,2,2,2,2,2,2,2,2,2,2,2,2,2,2,2,2,2,2,2,2,2,2,
2,2,2,4),(-2.26522078838353,-2.26308259399794,-2.25693981258274,-2.25284023844681,
-2.24872310822732,-2.24248348732369,-2.21750899752247,-2.20543732093632,
-2.20039952742394,-2.1964235329202,-2.19403734234458,-2.19162935858353,
-2.18754755221769,-2.16640898644128,-2.14528568850764,-2.13923643914338,
-2.13515356477946,-2.13101788062724,-2.12467702396361,-2.09653581488787,
-2.08206501963415,-2.07846030043459,-2.07616926507124,-2.07366955470286,
-2.06913589658524,-2.06310929138984,-2.04607122842413,-2.02841709108233,
-2.02201797082035,-2.01787146061176,-2.01379734268439,-2.00779834596808,
-1.98670039739742,-1.96536878402952,-1.96130208973809,-1.95889716275352,
-1.9565078201508,-1.95251701460299,-1.93475222207607,-1.91066124033276,
-1.90433542056805,-1.90020236482691,-1.89611681467631,-1.89005348759323,
-1.87021973428132,-1.84747068003657,-1.84355865588313,-1.84118535254758,
-1.83876269661744,-1.83460999337062,-1.8140591977983,-1.79330225303937,
-1.78685491281584,-1.78269934330518,-1.7786320627314,-1.77267286688305,
-1.75185578865277,-1.73006736381159,-1.72604729590666,-1.72365191112282,
-1.72125300185075,-1.71721599286741,-1.70024448108599,-1.67525693782621,
-1.66902112061544,-1.66490444095437,-1.66080373410641,-1.65465621681128,
-1.64734474690047,-1.63103832060014,-1.61286868402723,-1.60862889674959,
-1.60618844063525,-1.60382972574878,-1.5999907989241,-1.581928508261,-1.55784573596996,
-1.55151885739459,-1.54738549450721,-1.54329992039968,-1.53723709969949,
-1.52324866675719),.UNSPECIFIED.);
#1409=B_SPLINE_CURVE_WITH_KNOTS('',3,(#81507,#81508,#81509,#81510,#81511,
#81512,#81513,#81514,#81515,#81516,#81517,#81518,#81519,#81520,#81521,#81522,
#81523,#81524,#81525,#81526,#81527,#81528,#81529,#81530,#81531,#81532,#81533,
#81534,#81535,#81536,#81537,#81538,#81539,#81540,#81541,#81542,#81543,#81544,
#81545,#81546,#81547,#81548,#81549,#81550,#81551,#81552,#81553,#81554,#81555,
#81556,#81557,#81558,#81559,#81560,#81561,#81562,#81563,#81564,#81565,#81566,
#81567,#81568,#81569,#81570,#81571,#81572,#81573,#81574,#81575,#81576,#81577,
#81578,#81579,#81580,#81581,#81582,#81583,#81584,#81585,#81586,#81587,#81588,
#81589,#81590,#81591,#81592,#81593,#81594,#81595,#81596,#81597,#81598,#81599,
#81600,#81601,#81602,#81603,#81604,#81605,#81606,#81607,#81608,#81609,#81610,
#81611,#81612,#81613,#81614,#81615,#81616,#81617,#81618,#81619,#81620,#81621,
#81622,#81623,#81624,#81625,#81626,#81627,#81628,#81629,#81630,#81631,#81632,
#81633,#81634,#81635,#81636,#81637,#81638,#81639,#81640,#81641,#81642,#81643,
#81644,#81645,#81646,#81647,#81648,#81649,#81650,#81651,#81652,#81653,#81654,
#81655,#81656,#81657,#81658,#81659,#81660,#81661,#81662,#81663,#81664,#81665,
#81666,#81667,#81668,#81669,#81670),.UNSPECIFIED.,.F.,.F.,(4,2,2,2,2,2,
2,2,2,2,2,2,2,2,2,2,2,2,2,2,2,2,2,2,2,2,2,2,2,2,2,2,2,2,2,2,2,2,2,2,2,2,
2,2,2,2,2,2,2,2,2,2,2,2,2,2,2,2,2,2,2,2,2,2,2,2,2,2,2,2,2,2,2,2,2,2,2,2,
2,2,2,4),(-1.44487526904064,-1.43062984737927,-1.41166932931502,-1.40738566975182,
-1.40494593260971,-1.40261535681389,-1.39886860241393,-1.38034851879148,
-1.35661436093033,-1.35027508300439,-1.34615806805642,-1.34210834452718,
-1.33614034048275,-1.31407616250411,-1.29378691300726,-1.28966528623936,
-1.28725860501692,-1.28490189182519,-1.28102395582219,-1.27614599694567,
-1.26471335572167,-1.23845100779924,-1.23238592469723,-1.22872469179893,
-1.224701890561,-1.21888964878338,-1.21210482210727,-1.19792500750346,-1.17595889299071,
-1.1719687088649,-1.16958908958452,-1.16720714548371,-1.16320585665983,
-1.15811723983238,-1.14579098721926,-1.12130193050571,-1.11503026308992,
-1.11092564053181,-1.10686519674277,-1.10083722408066,-1.09370686577349,
-1.07813340894207,-1.05882589996639,-1.05459191763482,-1.05216222693181,
-1.04982406904773,-1.04603904753365,-1.02759080370476,-1.00385776998816,
-0.997518042517896,-0.993400815502081,-0.989350940765807,-0.983382823305888,
-0.961874524430739,-0.940974418390339,-0.936881568598389,-0.934480732566327,
-0.932118705269316,-0.928214880816489,-0.923293047667827,-0.911678893979217,
-0.885792076631254,-0.879678596145071,-0.876009379186951,-0.871993660070933,
-0.86622411731811,-0.844011970483475,-0.823407319914528,-0.81929679327984,
-0.816892282487142,-0.814533376066198,-0.810645143388851,-0.791982867570228,
-0.768730887866824,-0.762356001231897,-0.758232079599996,-0.754187146462191,
-0.748248162228047,-0.741261224667227,-0.726281828059949,-0.705827098954992,
-0.702969042438947),.UNSPECIFIED.);
#1410=B_SPLINE_CURVE_WITH_KNOTS('',3,(#81671,#81672,#81673,#81674,#81675,
#81676,#81677,#81678,#81679,#81680,#81681,#81682,#81683,#81684,#81685,#81686,
#81687,#81688,#81689,#81690,#81691,#81692,#81693,#81694,#81695,#81696,#81697,
#81698,#81699,#81700,#81701,#81702,#81703,#81704,#81705,#81706,#81707,#81708,
#81709,#81710,#81711,#81712,#81713,#81714,#81715,#81716,#81717,#81718,#81719,
#81720,#81721,#81722,#81723,#81724,#81725,#81726,#81727,#81728,#81729,#81730,
#81731,#81732,#81733,#81734,#81735,#81736,#81737,#81738,#81739,#81740,#81741,
#81742,#81743,#81744,#81745,#81746,#81747,#81748,#81749,#81750,#81751,#81752,
#81753,#81754,#81755,#81756,#81757,#81758,#81759,#81760,#81761,#81762,#81763,
#81764,#81765,#81766,#81767,#81768,#81769,#81770,#81771,#81772,#81773,#81774,
#81775,#81776,#81777,#81778,#81779,#81780,#81781,#81782,#81783,#81784,#81785,
#81786,#81787,#81788,#81789,#81790,#81791,#81792,#81793,#81794,#81795,#81796,
#81797,#81798,#81799,#81800,#81801,#81802,#81803,#81804,#81805,#81806,#81807,
#81808,#81809,#81810,#81811,#81812,#81813,#81814,#81815,#81816,#81817,#81818,
#81819,#81820,#81821,#81822,#81823,#81824,#81825,#81826,#81827,#81828,#81829,
#81830,#81831,#81832,#81833,#81834,#81835,#81836,#81837,#81838,#81839,#81840),
 .UNSPECIFIED.,.F.,.F.,(4,2,2,2,2,2,2,2,2,2,2,2,2,2,2,2,2,2,2,2,2,2,2,2,
2,2,2,2,2,2,2,2,2,2,2,2,2,2,2,2,2,2,2,2,2,2,2,2,2,2,2,2,2,2,2,2,2,2,2,2,
2,2,2,2,2,2,2,2,2,2,2,2,2,2,2,2,2,2,2,2,2,2,2,2,4),(-1.52324866675719,-1.52033948694185,
-1.49491652761532,-1.49086149540555,-1.48845884410359,-1.48606693510808,
-1.48206423426943,-1.464576274536,-1.44016478020395,-1.43386843330214,-1.42974055809692,
-1.42564983927897,-1.4195587965746,-1.39891350013134,-1.37726247730706,
-1.37322738445059,-1.3708288110181,-1.36843281177055,-1.36441037142123,
-1.34646534694613,-1.3226601758809,-1.31630893348182,-1.31217090829117,
-1.30808887530338,-1.30204703954764,-1.28028628276023,-1.2598149297332,
-1.25568711508309,-1.2532694336227,-1.2508912980067,-1.24695636826099,-1.24198963825706,
-1.23021989051971,-1.20466919832499,-1.19849760428866,-1.19439229965558,
-1.19027961413292,-1.18406736747959,-1.17665043516656,-1.15987311712153,
-1.14271501280928,-1.13830323226994,-1.13582773944788,-1.13349360265352,
-1.12978172171059,-1.11115855411566,-1.08744806506716,-1.08108884163973,
-1.07694922259553,-1.07286822135788,-1.06683292266412,-1.05970369631855,
-1.0441831043046,-1.0247689918805,-1.02054565334965,-1.01810838082529,-1.01574667637118,
-1.01189359919665,-1.00706569330692,-0.995869645306252,-0.969116546126487,
-0.963099356335427,-0.959428488351477,-0.955363899608925,-0.949422276953992,
-0.942443702819668,-0.92754338698631,-0.906973265529007,-0.902849440832177,
-0.900432550286804,-0.898053627391007,-0.894114959012901,-0.889141887826747,
-0.877345590066338,-0.851847482107216,-0.845669416357442,-0.841562888099976,
-0.837451298463795,-0.831245387628963,-0.823838877088501,-0.807109187457589,
-0.789873717327814,-0.785464752593549,-0.782989798471485,-0.781189504183713),
 .UNSPECIFIED.);
#1411=B_SPLINE_CURVE_WITH_KNOTS('',3,(#81845,#81846,#81847,#81848,#81849,
#81850,#81851,#81852,#81853,#81854,#81855,#81856,#81857,#81858,#81859,#81860,
#81861,#81862,#81863,#81864,#81865,#81866,#81867,#81868,#81869,#81870,#81871,
#81872,#81873,#81874,#81875,#81876,#81877,#81878,#81879,#81880,#81881,#81882,
#81883,#81884,#81885,#81886,#81887,#81888,#81889,#81890,#81891,#81892,#81893,
#81894,#81895,#81896,#81897,#81898,#81899,#81900,#81901,#81902,#81903,#81904,
#81905,#81906,#81907,#81908,#81909,#81910,#81911,#81912,#81913,#81914,#81915,
#81916,#81917,#81918,#81919,#81920,#81921,#81922,#81923,#81924,#81925,#81926,
#81927,#81928,#81929,#81930,#81931,#81932,#81933,#81934,#81935,#81936,#81937,
#81938,#81939,#81940,#81941,#81942,#81943,#81944,#81945,#81946,#81947,#81948,
#81949,#81950,#81951,#81952,#81953,#81954,#81955,#81956,#81957,#81958,#81959,
#81960,#81961,#81962,#81963,#81964,#81965,#81966,#81967,#81968,#81969,#81970,
#81971,#81972,#81973,#81974,#81975,#81976,#81977,#81978,#81979,#81980,#81981,
#81982,#81983,#81984,#81985,#81986,#81987,#81988,#81989,#81990,#81991,#81992,
#81993,#81994,#81995,#81996,#81997,#81998,#81999,#82000,#82001,#82002,#82003,
#82004,#82005,#82006,#82007,#82008,#82009,#82010,#82011,#82012,#82013,#82014,
#82015,#82016,#82017,#82018,#82019,#82020),.UNSPECIFIED.,.F.,.F.,(4,2,2,
2,2,2,2,2,2,2,2,2,2,2,2,2,2,2,2,2,2,2,2,2,2,2,2,2,2,2,2,2,2,2,2,2,2,2,2,
2,2,2,2,2,2,2,2,2,2,2,2,2,2,2,2,2,2,2,2,2,2,2,2,2,2,2,2,2,2,2,2,2,2,2,2,
2,2,2,2,2,2,2,2,2,2,2,2,4),(-2.18666954650822,-2.18265430661059,-2.17468325395502,
-2.1702613950192,-2.16634123326651,-2.16132410480541,-2.15020514347348,
-2.14447159053473,-2.12444638312029,-2.11796898048221,-2.1132001078031,
-2.11066396280014,-2.10838765255901,-2.10493605848464,-2.09267281405792,
-2.07197258198025,-2.05955812829991,-2.0543982159289,-2.0504608443663,-2.04611481916996,
-2.03855579425183,-2.02444249740545,-1.99920150751317,-1.99512526147699,
-1.99272810294192,-1.99036352894282,-1.98644589225988,-1.98150026422559,
-1.96978503799143,-1.94411305634687,-1.93797456013878,-1.933894650906,-1.92981200322807,
-1.92365851057852,-1.90544749943925,-1.88345742636239,-1.87830264824371,
-1.87569276320194,-1.87344170959043,-1.87015480057966,-1.85999980296953,
-1.83600964276,-1.82414778657502,-1.81908582455218,-1.81516018202226,-1.81076274478065,
-1.8029276613258,-1.77430265071792,-1.77195557261618,-1.76247473502744,
-1.75918039220243,-1.75692824579638,-1.75432182041591,-1.74918606042188,
-1.74199495318082,-1.71567166662637,-1.70559280344456,-1.7008144805518,
-1.69691602218718,-1.69226136869109,-1.68295731706708,-1.66957680557475,
-1.64636771777372,-1.6423400942397,-1.6399528415437,-1.63757868581714,-1.63361475909319,
-1.61704110497047,-1.59135934274745,-1.58522148386188,-1.58114151147117,
-1.57705843394237,-1.57090355729544,-1.55053878980004,-1.52874292237262,
-1.52473443215855,-1.52235110593306,-1.51997306880478,-1.51599037480901,
-1.51093363831038,-1.4987455538975,-1.47399873796849,-1.46775386383331,
-1.46365430058627,-1.45958971446674,-1.45353777798196,-1.44636855480763,
-1.44487526904064),.UNSPECIFIED.);
#1412=B_SPLINE_CURVE_WITH_KNOTS('',3,(#82021,#82022,#82023,#82024,#82025,
#82026,#82027,#82028,#82029,#82030,#82031,#82032,#82033,#82034,#82035,#82036,
#82037,#82038,#82039,#82040,#82041,#82042,#82043,#82044,#82045,#82046,#82047,
#82048,#82049,#82050,#82051,#82052,#82053,#82054,#82055,#82056,#82057,#82058,
#82059,#82060,#82061,#82062,#82063,#82064,#82065,#82066,#82067,#82068,#82069,
#82070,#82071,#82072,#82073,#82074,#82075,#82076,#82077,#82078,#82079,#82080,
#82081,#82082,#82083,#82084,#82085,#82086,#82087,#82088,#82089,#82090,#82091,
#82092,#82093,#82094,#82095,#82096,#82097,#82098,#82099,#82100,#82101,#82102,
#82103,#82104,#82105,#82106,#82107,#82108,#82109,#82110,#82111,#82112,#82113,
#82114,#82115,#82116,#82117,#82118,#82119,#82120,#82121,#82122,#82123,#82124,
#82125,#82126,#82127,#82128,#82129,#82130,#82131,#82132,#82133,#82134,#82135,
#82136,#82137,#82138,#82139,#82140,#82141,#82142,#82143,#82144,#82145,#82146,
#82147,#82148,#82149,#82150,#82151,#82152,#82153,#82154,#82155,#82156,#82157,
#82158,#82159,#82160,#82161,#82162,#82163,#82164,#82165,#82166,#82167,#82168,
#82169,#82170,#82171,#82172,#82173,#82174,#82175,#82176,#82177,#82178,#82179,
#82180,#82181,#82182,#82183,#82184,#82185,#82186,#82187,#82188,#82189,#82190),
 .UNSPECIFIED.,.F.,.F.,(4,2,2,2,2,2,2,2,2,2,2,2,2,2,2,2,2,2,2,2,2,2,2,2,
2,2,2,2,2,2,2,2,2,2,2,2,2,2,2,2,2,2,2,2,2,2,2,2,2,2,2,2,2,2,2,2,2,2,2,2,
2,2,2,2,2,2,2,2,2,2,2,2,2,2,2,2,2,2,2,2,2,2,2,2,4),(-0.781189504183713,
-0.780655240613857,-0.776941305076245,-0.772346214995282,-0.762066513925456,
-0.733221143074392,-0.727502757707771,-0.723515724568544,-0.719307952888275,
-0.712583482918676,-0.704309153500262,-0.683011120065911,-0.670596162685293,
-0.667063335226089,-0.664784680501353,-0.662259524594123,-0.657598599701539,
-0.651336361507989,-0.63283805493482,-0.615360290646342,-0.609755522501097,
-0.605746772659503,-0.601494157462634,-0.594531425340019,-0.571028994014777,
-0.554561149728483,-0.55020148730562,-0.547736514630781,-0.545395355475079,
-0.541646881678502,-0.536994339466273,-0.52649342671482,-0.498172460105221,
-0.492377186122633,-0.488377701902321,-0.484190979180804,-0.477578411693701,
-0.469494672792845,-0.449330386791692,-0.435490534037347,-0.431901374537632,
-0.429612920216069,-0.427107573766107,-0.422546551843302,-0.416469818003131,
-0.399134176424358,-0.381844159685263,-0.375456601816089,-0.371311887830329,
-0.367235452957319,-0.361225258681097,-0.354136395734053,-0.338783707851385,
-0.319007134063997,-0.314840540477088,-0.312414950353729,-0.310043825312622,
-0.306143347690164,-0.288820184287301,-0.263951657589763,-0.257702282803172,
-0.253582946323682,-0.249484256515147,-0.243348992444438,-0.236057639434028,
-0.219840712904032,-0.201532657939523,-0.197292273574692,-0.194851596625662,
-0.192492786310851,-0.188653884258802,-0.170597841935886,-0.146503855945698,
-0.140177451709205,-0.136043989488405,-0.131958019614313,-0.125894034856154,
-0.104317490247526,-0.0836976283859776,-0.0795762443453795,-0.0771598789088768,
-0.0747805548886755,-0.0708397932613529,-0.0542443252368777,-0.0391649357543273),
 .UNSPECIFIED.);
#1413=B_SPLINE_CURVE_WITH_KNOTS('',3,(#82195,#82196,#82197,#82198,#82199,
#82200,#82201,#82202,#82203,#82204,#82205,#82206,#82207,#82208,#82209,#82210,
#82211,#82212,#82213,#82214,#82215,#82216,#82217,#82218,#82219,#82220,#82221,
#82222,#82223,#82224,#82225,#82226,#82227,#82228,#82229,#82230,#82231,#82232,
#82233,#82234,#82235,#82236,#82237,#82238,#82239,#82240,#82241,#82242,#82243,
#82244,#82245,#82246,#82247,#82248,#82249,#82250,#82251,#82252,#82253,#82254,
#82255,#82256,#82257,#82258,#82259,#82260,#82261,#82262,#82263,#82264,#82265,
#82266,#82267,#82268,#82269,#82270,#82271,#82272,#82273,#82274,#82275,#82276,
#82277,#82278,#82279,#82280,#82281,#82282,#82283,#82284,#82285,#82286,#82287,
#82288,#82289,#82290,#82291,#82292,#82293,#82294,#82295,#82296,#82297,#82298,
#82299,#82300,#82301,#82302,#82303,#82304,#82305,#82306,#82307,#82308,#82309,
#82310,#82311,#82312,#82313,#82314,#82315,#82316,#82317,#82318,#82319,#82320,
#82321,#82322,#82323,#82324,#82325,#82326,#82327,#82328,#82329,#82330,#82331,
#82332,#82333,#82334,#82335,#82336,#82337,#82338,#82339,#82340,#82341,#82342,
#82343,#82344,#82345,#82346,#82347,#82348,#82349,#82350,#82351,#82352,#82353,
#82354,#82355,#82356,#82357,#82358,#82359,#82360,#82361,#82362),
 .UNSPECIFIED.,.F.,.F.,(4,2,2,2,2,2,2,2,2,2,2,2,2,2,2,2,2,2,2,2,2,2,2,2,
2,2,2,2,2,2,2,2,2,2,2,2,2,2,2,2,2,2,2,2,2,2,2,2,2,2,2,2,2,2,2,2,2,2,2,2,
2,2,2,2,2,2,2,2,2,2,2,2,2,2,2,2,2,2,2,2,2,2,2,4),(-2.92834915174502,-2.92648539545499,
-2.90657057780971,-2.88440378746991,-2.87834464423708,-2.87427953806933,
-2.87018271217011,-2.86394878545922,-2.83909422789314,-2.82695520076427,
-2.82190997785814,-2.81793460290906,-2.81555847767098,-2.81317439141761,
-2.80916037975621,-2.78745591004364,-2.76686983205887,-2.76080249131816,
-2.75673596941759,-2.75264085626061,-2.74641599461634,-2.72147563514041,
-2.70444372036,-2.70041885332621,-2.69803253890805,-2.69565860262891,-2.69169391475909,
-2.66953917970941,-2.65547278015069,-2.64871870517574,-2.64292574917221,
-2.63890705093035,-2.63524358385147,-2.62916052005398,-2.60303018211162,
-2.59152658888631,-2.58663165037125,-2.58274430789586,-2.58038614041258,
-2.5779824849785,-2.57387378004309,-2.55329554679192,-2.53114252347342,
-2.52535505457331,-2.52133725612151,-2.51767274506948,-2.51158340607721,
-2.48550217216042,-2.47397517831889,-2.46907458387598,-2.46518390366944,
-2.46282504496422,-2.46042215164099,-2.45631714677906,-2.43566536328569,
-2.42082590755425,-2.41387522508392,-2.40795885290461,-2.40391883798699,
-2.39979155408719,-2.39339369901535,-2.37054695202645,-2.35125846276003,
-2.34750404798006,-2.34517231985751,-2.34273531303893,-2.33846368736868,
-2.32355460516355,-2.31000987357397,-2.29985826215516,-2.29210107993466,
-2.28771846644346,-2.28379029529415,-2.27870285381457,-2.26662145045314,
-2.26299184174589,-2.24220586632793,-2.23562527315064,-2.23080228818918,
-2.22825562140187,-2.22600963290834,-2.22260711010118,-2.21177168803733,
-2.18666954650822),.UNSPECIFIED.);
#1414=B_SPLINE_CURVE_WITH_KNOTS('',3,(#82364,#82365,#82366,#82367,#82368,
#82369,#82370,#82371,#82372,#82373,#82374,#82375,#82376,#82377),
 .UNSPECIFIED.,.F.,.F.,(4,2,2,2,2,2,4),(-0.0391649357543273,-0.028591756921446,
-0.0224048677175574,-0.0182968878252835,-0.014597475923147,-0.0105493853881568,
-1.00000004773365E-6),.UNSPECIFIED.);
#1415=B_SPLINE_CURVE_WITH_KNOTS('',3,(#82378,#82379,#82380,#82381,#82382,
#82383,#82384,#82385,#82386,#82387,#82388,#82389,#82390,#82391,#82392,#82393,
#82394,#82395,#82396,#82397,#82398,#82399,#82400,#82401,#82402,#82403,#82404,
#82405,#82406,#82407,#82408,#82409,#82410,#82411,#82412,#82413,#82414,#82415,
#82416,#82417,#82418,#82419,#82420,#82421,#82422,#82423,#82424,#82425,#82426,
#82427,#82428,#82429,#82430,#82431,#82432,#82433,#82434,#82435,#82436,#82437,
#82438,#82439,#82440,#82441,#82442,#82443,#82444,#82445,#82446,#82447,#82448,
#82449,#82450,#82451,#82452,#82453,#82454,#82455,#82456,#82457,#82458,#82459,
#82460,#82461,#82462,#82463,#82464,#82465,#82466,#82467,#82468,#82469,#82470,
#82471,#82472,#82473,#82474,#82475,#82476,#82477,#82478,#82479,#82480,#82481,
#82482,#82483,#82484,#82485,#82486,#82487,#82488,#82489,#82490,#82491,#82492,
#82493,#82494,#82495,#82496,#82497,#82498,#82499,#82500,#82501,#82502,#82503,
#82504,#82505,#82506,#82507,#82508,#82509,#82510,#82511,#82512,#82513,#82514,
#82515,#82516,#82517,#82518,#82519,#82520,#82521,#82522,#82523,#82524,#82525,
#82526,#82527,#82528,#82529,#82530,#82531,#82532,#82533,#82534,#82535,#82536,
#82537,#82538,#82539),.UNSPECIFIED.,.F.,.F.,(4,2,2,2,2,2,2,2,2,2,2,2,2,
2,2,2,2,2,2,2,2,2,2,2,2,2,2,2,2,2,2,2,2,2,2,2,2,2,2,2,2,2,2,2,2,2,2,2,2,
2,2,2,2,2,2,2,2,2,2,2,2,2,2,2,2,2,2,2,2,2,2,2,2,2,2,2,2,2,2,2,4),(-2.14624791579464,
-2.11682697548836,-2.11191450843237,-2.10801217294024,-2.10564120580342,
-2.10321708034896,-2.09905535929736,-2.07928053471196,-2.05878385807118,
-2.05182022040338,-2.04756841143487,-2.04356121279034,-2.0379600049088,
-2.02061003096647,-2.001997857921,-1.99571792954008,-1.99104833667306,-1.98852199165158,
-1.98624496507717,-1.98271872719268,-1.97035451983186,-1.94903929875685,
-1.94076551026284,-1.93404135305729,-1.92983454252486,-1.92584884944796,
-1.92013323004753,-1.89126559413484,-1.88098907506257,-1.87639513136064,
-1.87268248936122,-1.87034867987337,-1.8678743549837,-1.86346634259697,
-1.8462841980142,-1.82954674218639,-1.8221404544652,-1.81593460737231,-1.81182386836759,
-1.80771874310254,-1.80154399454501,-1.77601191669446,-1.7642245860807,
-1.75925383792374,-1.75531715352806,-1.75293909285403,-1.75052261720979,
-1.74639889067038,-1.72588776350962,-1.70411878866479,-1.69811592715585,
-1.69404148523728,-1.68989640962819,-1.68350336256872,-1.66025901138639,
-1.64189400989191,-1.63783412083529,-1.6354307787598,-1.63333181093117,
-1.62964835604535,-1.61123777804337,-1.59441803341239,-1.58699348297927,
-1.58077639757357,-1.57666346996609,-1.57256008239933,-1.56639577500432,
-1.54077333289484,-1.52902954345837,-1.52406903556741,-1.52013830817635,
-1.51776137542678,-1.51534336024632,-1.5112125542358,-1.49089173662272,
-1.46855338366538,-1.46272685059151,-1.4586826412617,-1.45499297466204,
-1.4488554269585,-1.44355213348337),.UNSPECIFIED.);
#1416=B_SPLINE_CURVE_WITH_KNOTS('',3,(#82544,#82545,#82546,#82547,#82548,
#82549,#82550,#82551,#82552,#82553,#82554,#82555,#82556,#82557,#82558,#82559,
#82560,#82561,#82562,#82563,#82564,#82565,#82566,#82567,#82568,#82569,#82570,
#82571,#82572,#82573,#82574,#82575,#82576,#82577,#82578,#82579,#82580,#82581,
#82582,#82583,#82584,#82585,#82586,#82587,#82588,#82589,#82590,#82591,#82592,
#82593,#82594,#82595,#82596,#82597,#82598,#82599,#82600,#82601,#82602,#82603,
#82604,#82605,#82606,#82607,#82608,#82609,#82610,#82611,#82612,#82613,#82614,
#82615,#82616,#82617,#82618,#82619,#82620,#82621,#82622,#82623,#82624,#82625,
#82626,#82627,#82628,#82629,#82630,#82631,#82632,#82633,#82634,#82635,#82636,
#82637,#82638,#82639,#82640,#82641,#82642,#82643,#82644,#82645,#82646,#82647,
#82648,#82649,#82650,#82651,#82652,#82653,#82654,#82655,#82656,#82657,#82658,
#82659,#82660,#82661,#82662,#82663,#82664,#82665,#82666,#82667,#82668,#82669,
#82670,#82671,#82672,#82673,#82674,#82675,#82676,#82677,#82678,#82679,#82680,
#82681,#82682,#82683,#82684,#82685,#82686,#82687,#82688,#82689,#82690,#82691,
#82692,#82693,#82694,#82695,#82696,#82697,#82698,#82699,#82700,#82701,#82702,
#82703,#82704,#82705,#82706,#82707,#82708,#82709,#82710,#82711,#82712,#82713),
 .UNSPECIFIED.,.F.,.F.,(4,2,2,2,2,2,2,2,2,2,2,2,2,2,2,2,2,2,2,2,2,2,2,2,
2,2,2,2,2,2,2,2,2,2,2,2,2,2,2,2,2,2,2,2,2,2,2,2,2,2,2,2,2,2,2,2,2,2,2,2,
2,2,2,2,2,2,2,2,2,2,2,2,2,2,2,2,2,2,2,2,2,2,2,2,4),(-3.66997076696365,-3.66294180694855,
-3.64426115795585,-3.64050467059312,-3.63818112719387,-3.63575399153715,
-3.63152917797224,-3.612213653117,-3.59665330604222,-3.58952479255085,-3.58349585925373,
-3.57943245828912,-3.5753224675822,-3.56903605589188,-3.54480508468909,
-3.53239640017913,-3.52728865662214,-3.52327589590202,-3.52088882330274,
-3.51850752236118,-3.51451282651347,-3.49262660089069,-3.47843969843768,
-3.47165429679745,-3.46584137656891,-3.46181817679182,-3.45815644616426,
-3.45209017892872,-3.4258089356034,-3.41437171898407,-3.40949255675202,
-3.4056143842269,-3.40325796395558,-3.40085359489583,-3.39673715889808,
-3.37639514003859,-3.36137687286919,-3.35438339029674,-3.34844121742013,
-3.34439872436269,-3.34028110822169,-3.33392473282489,-3.31041384368027,
-3.29175818348476,-3.28797315464772,-3.28563649178251,-3.28320878672761,
-3.27898223096482,-3.25967453651895,-3.23676792931688,-3.23084402376541,
-3.22680248622695,-3.22267645110078,-3.21628629275609,-3.19332372429606,
-3.17471753181634,-3.17066722116852,-3.16827529780673,-3.16590587466695,
-3.16196356985642,-3.13961256319151,-3.11943373479543,-3.1134164099454,
-3.10935878072073,-3.10525356706946,-3.09897397222717,-3.07456046435438,
-3.05691482608817,-3.05299613987827,-3.05063168832136,-3.04823552090782,
-3.04416238790833,-3.02306482803221,-3.00148036166669,-2.99564343064258,
-2.99161758065946,-2.98796242830071,-2.98192893430487,-2.95542319602778,
-2.94409808144442,-2.93924667132723,-2.93538510583023,-2.93303231518504,
-2.93062283455467,-2.92834915174502),.UNSPECIFIED.);
#1417=B_SPLINE_CURVE_WITH_KNOTS('',3,(#82714,#82715,#82716,#82717,#82718,
#82719,#82720,#82721,#82722,#82723,#82724,#82725,#82726,#82727,#82728,#82729,
#82730,#82731,#82732,#82733,#82734,#82735,#82736,#82737,#82738,#82739,#82740,
#82741,#82742,#82743,#82744,#82745,#82746,#82747,#82748,#82749,#82750,#82751,
#82752,#82753,#82754,#82755,#82756,#82757,#82758,#82759,#82760,#82761,#82762,
#82763,#82764,#82765,#82766,#82767,#82768,#82769,#82770,#82771,#82772,#82773,
#82774,#82775,#82776,#82777,#82778,#82779,#82780,#82781,#82782,#82783,#82784,
#82785,#82786,#82787,#82788,#82789,#82790,#82791,#82792,#82793,#82794,#82795,
#82796,#82797,#82798,#82799,#82800,#82801,#82802,#82803,#82804,#82805,#82806,
#82807,#82808,#82809,#82810,#82811,#82812,#82813,#82814,#82815,#82816,#82817,
#82818,#82819,#82820,#82821,#82822,#82823,#82824,#82825,#82826,#82827,#82828,
#82829,#82830,#82831,#82832,#82833,#82834,#82835,#82836,#82837,#82838,#82839,
#82840,#82841,#82842,#82843,#82844,#82845,#82846,#82847,#82848,#82849,#82850,
#82851,#82852,#82853,#82854,#82855,#82856,#82857,#82858,#82859,#82860,#82861,
#82862,#82863,#82864,#82865,#82866,#82867),.UNSPECIFIED.,.F.,.F.,(4,2,2,
2,2,2,2,2,2,2,2,2,2,2,2,2,2,2,2,2,2,2,2,2,2,2,2,2,2,2,2,2,2,2,2,2,2,2,2,
2,2,2,2,2,2,2,2,2,2,2,2,2,2,2,2,2,2,2,2,2,2,2,2,2,2,2,2,2,2,2,2,2,2,2,2,
2,4),(-1.44355213348337,-1.42301543780805,-1.40655434363128,-1.40257766687356,
-1.40019134752506,-1.39778355717221,-1.39370257389229,-1.37255529451872,
-1.35153902219749,-1.34544338593644,-1.34135230270311,-1.33722610537493,
-1.33093665219751,-1.30643778848766,-1.29411604231323,-1.28902046629015,
-1.28501082378166,-1.28261775410596,-1.28021701256442,-1.27617031134857,
-1.25466502244134,-1.23393195372578,-1.22784136521807,-1.22375115021584,
-1.21962388911123,-1.21332880743686,-1.18888661429008,-1.17127249369206,
-1.16734094647008,-1.16496377779633,-1.16254573364486,-1.15841528914934,
-1.1380780290576,-1.11605602989744,-1.11009331423373,-1.10602556694194,
-1.10187100172189,-1.0954285010926,-1.07326504094764,-1.05434362231351,
-1.05004722443417,-1.04759531103085,-1.04524565591727,-1.04145175831556,
-1.02328210548449,-0.999225218586492,-0.992896463345815,-0.988763089298828,
-0.984678413869209,-0.978618734925012,-0.971449588671737,-0.955757844739731,
-0.936736786583105,-0.932446677685336,-0.929996119836072,-0.92764540003064,
-0.923846597217638,-0.905564985962089,-0.88165398141841,-0.875311969236898,
-0.871175831619516,-0.867092669699315,-0.861043370105454,-0.84033442210889,
-0.818657937267153,-0.814625936221056,-0.81222798593872,-0.809830686461947,
-0.805803478545767,-0.788459744445454,-0.763940411053372,-0.757656361673641,
-0.753530381495941,-0.749436906878411,-0.743332543829005,-0.721970195697778,
-0.701564423551126),.UNSPECIFIED.);
#1418=B_SPLINE_CURVE_WITH_KNOTS('',3,(#82870,#82871,#82872,#82873,#82874,
#82875,#82876,#82877,#82878,#82879,#82880,#82881,#82882,#82883,#82884,#82885,
#82886,#82887,#82888,#82889,#82890,#82891,#82892,#82893,#82894,#82895,#82896,
#82897,#82898,#82899,#82900,#82901,#82902,#82903,#82904,#82905,#82906,#82907,
#82908,#82909,#82910,#82911,#82912,#82913,#82914,#82915,#82916,#82917,#82918,
#82919,#82920,#82921,#82922,#82923,#82924,#82925,#82926,#82927,#82928,#82929,
#82930,#82931,#82932,#82933,#82934,#82935,#82936,#82937,#82938,#82939,#82940,
#82941,#82942,#82943,#82944,#82945,#82946,#82947,#82948,#82949,#82950,#82951,
#82952,#82953,#82954,#82955,#82956,#82957,#82958,#82959,#82960,#82961,#82962,
#82963,#82964,#82965,#82966,#82967,#82968,#82969,#82970,#82971,#82972,#82973,
#82974,#82975,#82976,#82977,#82978,#82979,#82980,#82981,#82982,#82983,#82984,
#82985,#82986,#82987,#82988,#82989,#82990,#82991,#82992,#82993,#82994,#82995,
#82996,#82997,#82998,#82999,#83000,#83001,#83002,#83003,#83004,#83005,#83006,
#83007,#83008,#83009,#83010,#83011,#83012,#83013,#83014,#83015,#83016,#83017,
#83018,#83019,#83020,#83021,#83022,#83023,#83024,#83025),.UNSPECIFIED.,
 .F.,.F.,(4,2,2,2,2,2,2,2,2,2,2,2,2,2,2,2,2,2,2,2,2,2,2,2,2,2,2,2,2,2,2,
2,2,2,2,2,2,2,2,2,2,2,2,2,2,2,2,2,2,2,2,2,2,2,2,2,2,2,2,2,2,2,2,2,2,2,2,
2,2,2,2,2,2,2,2,2,2,4),(-0.701564423551126,-0.70120887792929,-0.697095716149052,
-0.694681121607495,-0.692302216844747,-0.688358159211799,-0.671215668528298,
-0.646207462961748,-0.639973371958886,-0.635858658508875,-0.63176077592468,
-0.625619644994713,-0.618317381956628,-0.602047279863736,-0.583817118074423,
-0.57957988052083,-0.577140638947338,-0.574781543544154,-0.570941971037803,
-0.552883380963188,-0.528778706105412,-0.522450294566862,-0.518315221127886,
-0.51422732897638,-0.508159518769005,-0.486448779636048,-0.465998345568823,
-0.461868937046329,-0.459449672004075,-0.457064787709155,-0.453113098979084,
-0.435276881029289,-0.411288538973521,-0.4049621879785,-0.400824959155111,
-0.396731659601096,-0.39064872841958,-0.368705608078459,-0.348488244140866,
-0.344351519882306,-0.341932094030867,-0.339571230028095,-0.335678923917613,
-0.330778486760952,-0.319266448756615,-0.292994857381811,-0.286904445355541,
-0.283235428695515,-0.279209860939718,-0.273405467744888,-0.251123711630572,
-0.230683987863599,-0.226561196860336,-0.22415020383434,-0.221765645110252,
-0.217826991987676,-0.212859430033859,-0.201111108768999,-0.175443825837061,
-0.16925949427639,-0.165546772028951,-0.161479507727689,-0.155621091119772,
-0.148784180969686,-0.134471932177159,-0.112908310051021,-0.10885362024273,
-0.106437488582663,-0.10398511976884,-0.0998182124646509,-0.0860912770649259,
-0.0578102541858007,-0.0521234685116127,-0.0480733705491654,-0.0437859888948185,
-0.0367789174125886,-0.0191482594977915,-9.9999999203515E-7),
 .UNSPECIFIED.);
#1419=B_SPLINE_CURVE_WITH_KNOTS('',3,(#83028,#83029,#83030,#83031,#83032,
#83033,#83034,#83035,#83036,#83037,#83038,#83039,#83040,#83041,#83042,#83043,
#83044,#83045,#83046,#83047,#83048,#83049,#83050,#83051,#83052,#83053,#83054,
#83055,#83056,#83057,#83058,#83059,#83060,#83061,#83062,#83063,#83064,#83065,
#83066,#83067,#83068,#83069,#83070,#83071,#83072,#83073,#83074,#83075,#83076,
#83077,#83078,#83079,#83080,#83081,#83082,#83083,#83084,#83085,#83086,#83087,
#83088,#83089,#83090,#83091,#83092,#83093,#83094,#83095,#83096,#83097,#83098,
#83099,#83100,#83101,#83102,#83103,#83104,#83105,#83106,#83107,#83108,#83109,
#83110,#83111,#83112,#83113,#83114,#83115,#83116,#83117,#83118,#83119,#83120,
#83121,#83122,#83123,#83124,#83125,#83126,#83127,#83128,#83129,#83130,#83131,
#83132,#83133,#83134,#83135,#83136,#83137,#83138,#83139,#83140,#83141,#83142,
#83143,#83144,#83145,#83146,#83147,#83148,#83149),.UNSPECIFIED.,.F.,.F.,
(4,2,2,2,2,2,2,2,2,2,2,2,2,2,2,2,2,2,2,2,2,2,2,2,2,2,2,2,2,2,2,2,2,2,2,
2,2,2,2,2,2,2,2,2,2,2,2,2,2,2,2,2,2,2,2,2,2,2,2,2,4),(-4.22604418082236,
-4.22327808819264,-4.21936102739766,-4.20446094842647,-4.18747903018636,
-4.1784044142109,-4.17352044405151,-4.16917793782232,-4.16354724173028,
-4.15022279373838,-4.1247504044384,-4.11405063405918,-4.1106751761705,-4.10840872753587,
-4.10591099704085,-4.10114736551919,-4.07911669802533,-4.05988874042377,
-4.05439438983799,-4.05054390573677,-4.04654084487888,-4.04021988412612,
-4.01078559856294,-3.99592082562229,-3.99242451620271,-3.99020252309191,
-3.98778065258953,-3.98355602167842,-3.96532102768477,-3.94893593290557,
-3.94159330497221,-3.9354178205971,-3.93130514256401,-3.92717969575918,
-3.92092861481171,-3.89716054925069,-3.87997595375218,-3.87594227719154,
-3.87352789074872,-3.87111022066475,-3.86699429741439,-3.84635401791738,
-3.82500461185571,-3.81891287446586,-3.8148259907035,-3.81070524239449,
-3.80442740071324,-3.77975359558416,-3.76221884051506,-3.75831568850624,
-3.75594897840387,-3.75355536725498,-3.74946674208105,-3.72866181678669,
-3.7139093692567,-3.70698993964141,-3.70109998253778,-3.69708028489806,
-3.69297748624435,-3.68663051522063,-3.66997076696365),.UNSPECIFIED.);
#1420=B_SPLINE_CURVE_WITH_KNOTS('',3,(#83152,#83153,#83154,#83155,#83156,
#83157,#83158,#83159,#83160,#83161,#83162,#83163,#83164,#83165,#83166,#83167,
#83168,#83169,#83170,#83171,#83172,#83173,#83174,#83175,#83176,#83177,#83178,
#83179,#83180,#83181,#83182,#83183,#83184,#83185,#83186,#83187,#83188,#83189,
#83190,#83191,#83192,#83193,#83194,#83195,#83196,#83197,#83198,#83199,#83200,
#83201,#83202,#83203,#83204,#83205,#83206,#83207,#83208,#83209,#83210,#83211,
#83212,#83213),.UNSPECIFIED.,.F.,.F.,(4,2,2,2,2,2,2,2,2,2,2,2,2,2,2,2,2,
2,2,2,2,2,2,2,2,2,2,2,2,2,4),(0.92152398119564,0.930542222948303,0.957906397135821,
0.973640877462175,0.977498361941586,0.979857594612128,0.982204734629106,
0.985951860520987,1.00046378666866,1.01856980625822,1.04243182151719,1.04871023144959,
1.05284712047941,1.05690439042067,1.0627623999138,1.08071549850968,1.09844311768674,
1.11777276359001,1.12263743664607,1.12525436516788,1.12752019267841,1.13070941500142,
1.13909585654484,1.15339032086897,1.18592444577795,1.192762696269,1.19702020211664,
1.20102944399565,1.20654207318242,1.22099205936091,1.25994577360142),
 .UNSPECIFIED.);
#1421=B_SPLINE_CURVE_WITH_KNOTS('',3,(#83216,#83217,#83218,#83219,#83220,
#83221,#83222,#83223,#83224,#83225,#83226,#83227,#83228,#83229,#83230,#83231,
#83232,#83233,#83234,#83235,#83236,#83237,#83238,#83239,#83240,#83241,#83242,
#83243,#83244,#83245,#83246,#83247,#83248,#83249,#83250,#83251,#83252,#83253,
#83254,#83255),.UNSPECIFIED.,.F.,.F.,(4,3,3,3,3,3,3,3,3,3,3,3,3,4),(-55.7692743084766,
-55.6534283704756,-55.5376479305359,-55.4219003996767,-55.3061487166547,
-55.1903558265821,-55.0743879116938,-54.9583269182872,-54.8420216706817,
-54.7733944101109,-54.6509097908543,-54.5288171495205,-54.4072911748158,
-54.357512134614),.UNSPECIFIED.);
#1422=B_SPLINE_CURVE_WITH_KNOTS('',3,(#83260,#83261,#83262,#83263,#83264,
#83265,#83266,#83267,#83268,#83269,#83270,#83271,#83272,#83273,#83274,#83275,
#83276,#83277,#83278,#83279,#83280,#83281,#83282,#83283,#83284,#83285,#83286,
#83287,#83288,#83289,#83290,#83291,#83292,#83293,#83294,#83295,#83296,#83297,
#83298,#83299,#83300,#83301,#83302,#83303,#83304,#83305,#83306,#83307,#83308,
#83309,#83310,#83311,#83312,#83313,#83314,#83315,#83316,#83317,#83318,#83319,
#83320,#83321,#83322,#83323,#83324,#83325,#83326,#83327,#83328,#83329,#83330,
#83331,#83332,#83333,#83334,#83335,#83336,#83337,#83338,#83339,#83340,#83341),
 .UNSPECIFIED.,.F.,.F.,(4,3,3,3,3,3,3,3,3,3,3,3,3,3,3,3,3,3,3,3,3,3,3,3,
3,3,3,4),(-0.272764230797882,-0.263475368935032,-0.246182477441445,-0.240296053772436,
-0.236376273825625,-0.219184076385875,-0.207427596460933,-0.200432152586668,
-0.196882035074211,-0.180129152494627,-0.163789452319017,-0.154125148485847,
-0.147447841209237,-0.144264614013768,-0.128407246391035,-0.125132236986337,
-0.108107959964319,-0.100850780960037,-0.0956258708151819,-0.0925979657742817,
-0.0768293113674334,-0.0611426794964475,-0.0532929528702713,-0.0475077680039616,
-0.044709499816088,-0.0296052680449404,-0.0148026340224702,0.),
 .UNSPECIFIED.);
#1423=B_SPLINE_CURVE_WITH_KNOTS('',3,(#83342,#83343,#83344,#83345,#83346,
#83347,#83348,#83349,#83350,#83351,#83352,#83353,#83354,#83355),
 .UNSPECIFIED.,.F.,.F.,(4,2,2,2,2,2,4),(9.99999998373441E-7,0.0491146626752611,
0.105092462623141,0.156860905302085,0.207178766483019,0.253689158846026,
0.301589346947622),.UNSPECIFIED.);
#1424=B_SPLINE_CURVE_WITH_KNOTS('',3,(#83593,#83594,#83595,#83596,#83597,
#83598),.UNSPECIFIED.,.F.,.F.,(4,2,4),(8.94639846984786E-5,0.00139415313563322,
0.00270203214836627),.UNSPECIFIED.);
#1425=B_SPLINE_CURVE_WITH_KNOTS('',3,(#83600,#83601,#83602,#83603,#83604,
#83605,#83606,#83607,#83608,#83609,#83610,#83611,#83612,#83613,#83614,#83615,
#83616,#83617,#83618,#83619,#83620,#83621,#83622,#83623,#83624,#83625,#83626,
#83627,#83628,#83629,#83630,#83631,#83632,#83633,#83634,#83635,#83636,#83637,
#83638,#83639,#83640,#83641,#83642,#83643,#83644,#83645,#83646,#83647,#83648,
#83649,#83650,#83651,#83652,#83653,#83654,#83655,#83656,#83657,#83658,#83659,
#83660,#83661,#83662,#83663,#83664,#83665,#83666,#83667,#83668,#83669,#83670,
#83671,#83672,#83673,#83674,#83675,#83676,#83677,#83678,#83679,#83680,#83681,
#83682,#83683,#83684),.UNSPECIFIED.,.F.,.F.,(4,3,3,3,3,3,3,3,3,3,3,3,3,
3,3,3,3,3,3,3,3,3,3,3,3,3,3,3,4),(-0.276631791712689,-0.266883590802822,
-0.252249399427331,-0.244999997209827,-0.241627787357496,-0.226344420306036,
-0.215574858042148,-0.211659554221128,-0.208411272807924,-0.192637118028121,
-0.176589721765353,-0.167489271872747,-0.162477936424474,-0.159585284717452,
-0.143058486365342,-0.14018792219493,-0.124233629563743,-0.116077598840496,
-0.111101224229059,-0.107818411217943,-0.0912654477597725,-0.0743517206583661,
-0.0648501306250925,-0.0586269416525286,-0.0554893882620879,-0.0380440320810531,
-0.0205562383343915,-0.0034758551960099,0.),.UNSPECIFIED.);
#1426=B_SPLINE_CURVE_WITH_KNOTS('',3,(#83685,#83686,#83687,#83688),
 .UNSPECIFIED.,.F.,.F.,(4,4),(-0.0126687472591452,0.),.UNSPECIFIED.);
#1427=B_SPLINE_CURVE_WITH_KNOTS('',3,(#83694,#83695,#83696,#83697,#83698,
#83699,#83700,#83701,#83702,#83703,#83704,#83705,#83706,#83707,#83708,#83709,
#83710,#83711,#83712,#83713,#83714,#83715,#83716,#83717,#83718,#83719,#83720,
#83721,#83722,#83723,#83724,#83725,#83726,#83727,#83728,#83729,#83730,#83731,
#83732,#83733,#83734,#83735,#83736,#83737,#83738,#83739,#83740,#83741,#83742,
#83743,#83744,#83745,#83746,#83747,#83748,#83749,#83750,#83751,#83752,#83753,
#83754,#83755,#83756,#83757,#83758,#83759,#83760,#83761,#83762,#83763,#83764,
#83765,#83766,#83767,#83768,#83769,#83770,#83771,#83772,#83773,#83774,#83775),
 .UNSPECIFIED.,.F.,.F.,(4,3,3,3,3,3,3,3,3,3,3,3,3,3,3,3,3,3,3,3,3,3,3,3,
3,3,3,4),(-0.272764372285567,-0.263475368935033,-0.246182477441449,-0.240296056377085,
-0.236376276566156,-0.219184079084204,-0.207427598821973,-0.200432157374891,
-0.196882034480836,-0.180129152830584,-0.163789459713166,-0.154125154031464,
-0.147447858424305,-0.144264611189609,-0.128407250478866,-0.12513223698636,
-0.108107874550581,-0.100850758306321,-0.0956258537310135,-0.0925979610886074,
-0.0768293076421143,-0.0611426692443636,-0.0532929493125631,-0.0475077621206312,
-0.0447094944615889,-0.0296052542868889,-0.0148026271434445,0.),
 .UNSPECIFIED.);
#1428=B_SPLINE_CURVE_WITH_KNOTS('',3,(#84012,#84013,#84014,#84015,#84016,
#84017),.UNSPECIFIED.,.F.,.F.,(4,2,4),(-0.0027018865616397,-0.00139407808319273,
-8.94593391793846E-5),.UNSPECIFIED.);
#1721=SHAPE_REPRESENTATION_RELATIONSHIP('SRR','None',#135345,#1734);
#1734=ADVANCED_BREP_SHAPE_REPRESENTATION('',(#1760),#135277);
#1747=STYLED_ITEM('',(#135419),#1760);
#1760=MANIFOLD_SOLID_BREP('Body1',#32083);
#1856=CYLINDRICAL_SURFACE('',#33413,1.4635);
#1857=CYLINDRICAL_SURFACE('',#33415,1.4635);
#1858=CYLINDRICAL_SURFACE('',#33416,1.4635);
#1859=CYLINDRICAL_SURFACE('',#33417,1.4635);
#1860=CYLINDRICAL_SURFACE('',#33418,1.4635);
#1861=CYLINDRICAL_SURFACE('',#33419,1.4635);
#1862=CYLINDRICAL_SURFACE('',#33420,1.4635);
#1863=CYLINDRICAL_SURFACE('',#33421,1.4635);
#1864=CYLINDRICAL_SURFACE('',#33422,1.4635);
#1865=CYLINDRICAL_SURFACE('',#33423,1.17775);
#1866=CYLINDRICAL_SURFACE('',#33425,1.17775);
#1867=CYLINDRICAL_SURFACE('',#33426,1.17775);
#1868=CYLINDRICAL_SURFACE('',#33427,1.17775);
#1869=CYLINDRICAL_SURFACE('',#33428,1.17775);
#1870=CYLINDRICAL_SURFACE('',#33429,1.17775);
#1871=CYLINDRICAL_SURFACE('',#33430,1.17775);
#1872=CYLINDRICAL_SURFACE('',#33431,1.17775);
#1873=CYLINDRICAL_SURFACE('',#33432,1.17775);
#1874=CYLINDRICAL_SURFACE('',#33434,1.4635);
#1875=CYLINDRICAL_SURFACE('',#33450,0.816025403784426);
#1876=CYLINDRICAL_SURFACE('',#33452,0.816025403784426);
#1877=CYLINDRICAL_SURFACE('',#33454,0.816025403784426);
#1878=CYLINDRICAL_SURFACE('',#33456,0.816025403784426);
#1879=CYLINDRICAL_SURFACE('',#33458,0.816025403784426);
#1880=CYLINDRICAL_SURFACE('',#33460,0.816025403784426);
#2214=FACE_BOUND('',#6601,.T.);
#3042=PLANE('',#33436);
#3043=PLANE('',#33439);
#3044=PLANE('',#33462);
#3045=PLANE('',#33463);
#3046=PLANE('',#33464);
#3047=PLANE('',#33465);
#3048=PLANE('',#33466);
#3049=PLANE('',#33467);
#3050=PLANE('',#33468);
#3051=PLANE('',#33469);
#3052=PLANE('',#33470);
#3053=PLANE('',#33471);
#3054=PLANE('',#33473);
#3055=PLANE('',#33475);
#3056=PLANE('',#33477);
#3057=PLANE('',#33479);
#3058=PLANE('',#33481);
#3059=PLANE('',#33484);
#3060=PLANE('',#33485);
#3061=PLANE('',#33486);
#3062=PLANE('',#33487);
#3063=PLANE('',#33492);
#4596=FACE_OUTER_BOUND('',#6548,.T.);
#4597=FACE_OUTER_BOUND('',#6549,.T.);
#4598=FACE_OUTER_BOUND('',#6550,.T.);
#4599=FACE_OUTER_BOUND('',#6551,.T.);
#4600=FACE_OUTER_BOUND('',#6552,.T.);
#4601=FACE_OUTER_BOUND('',#6553,.T.);
#4602=FACE_OUTER_BOUND('',#6554,.T.);
#4603=FACE_OUTER_BOUND('',#6555,.T.);
#4604=FACE_OUTER_BOUND('',#6556,.T.);
#4605=FACE_OUTER_BOUND('',#6557,.T.);
#4606=FACE_OUTER_BOUND('',#6558,.T.);
#4607=FACE_OUTER_BOUND('',#6559,.T.);
#4608=FACE_OUTER_BOUND('',#6560,.T.);
#4609=FACE_OUTER_BOUND('',#6561,.T.);
#4610=FACE_OUTER_BOUND('',#6562,.T.);
#4611=FACE_OUTER_BOUND('',#6563,.T.);
#4612=FACE_OUTER_BOUND('',#6564,.T.);
#4613=FACE_OUTER_BOUND('',#6565,.T.);
#4614=FACE_OUTER_BOUND('',#6566,.T.);
#4615=FACE_OUTER_BOUND('',#6567,.T.);
#4616=FACE_OUTER_BOUND('',#6568,.T.);
#4617=FACE_OUTER_BOUND('',#6569,.T.);
#4618=FACE_OUTER_BOUND('',#6570,.T.);
#4619=FACE_OUTER_BOUND('',#6571,.T.);
#4620=FACE_OUTER_BOUND('',#6572,.T.);
#4621=FACE_OUTER_BOUND('',#6573,.T.);
#4622=FACE_OUTER_BOUND('',#6574,.T.);
#4623=FACE_OUTER_BOUND('',#6575,.T.);
#4624=FACE_OUTER_BOUND('',#6576,.T.);
#4625=FACE_OUTER_BOUND('',#6577,.T.);
#4626=FACE_OUTER_BOUND('',#6578,.T.);
#4627=FACE_OUTER_BOUND('',#6579,.T.);
#4628=FACE_OUTER_BOUND('',#6580,.T.);
#4629=FACE_OUTER_BOUND('',#6581,.T.);
#4630=FACE_OUTER_BOUND('',#6582,.T.);
#4631=FACE_OUTER_BOUND('',#6583,.T.);
#4632=FACE_OUTER_BOUND('',#6584,.T.);
#4633=FACE_OUTER_BOUND('',#6585,.T.);
#4634=FACE_OUTER_BOUND('',#6586,.T.);
#4635=FACE_OUTER_BOUND('',#6587,.T.);
#4636=FACE_OUTER_BOUND('',#6588,.T.);
#4637=FACE_OUTER_BOUND('',#6589,.T.);
#4638=FACE_OUTER_BOUND('',#6590,.T.);
#4639=FACE_OUTER_BOUND('',#6591,.T.);
#4640=FACE_OUTER_BOUND('',#6592,.T.);
#4641=FACE_OUTER_BOUND('',#6593,.T.);
#4642=FACE_OUTER_BOUND('',#6594,.T.);
#4643=FACE_OUTER_BOUND('',#6595,.T.);
#4644=FACE_OUTER_BOUND('',#6596,.T.);
#4645=FACE_OUTER_BOUND('',#6597,.T.);
#4646=FACE_OUTER_BOUND('',#6598,.T.);
#4647=FACE_OUTER_BOUND('',#6599,.T.);
#4648=FACE_OUTER_BOUND('',#6600,.T.);
#6548=EDGE_LOOP('',(#27346,#27347,#27348,#27349));
#6549=EDGE_LOOP('',(#27350,#27351,#27352,#27353));
#6550=EDGE_LOOP('',(#27354,#27355,#27356,#27357));
#6551=EDGE_LOOP('',(#27358,#27359,#27360,#27361,#27362,#27363));
#6552=EDGE_LOOP('',(#27364,#27365,#27366,#27367,#27368));
#6553=EDGE_LOOP('',(#27369,#27370,#27371,#27372));
#6554=EDGE_LOOP('',(#27373,#27374,#27375,#27376,#27377));
#6555=EDGE_LOOP('',(#27378,#27379,#27380,#27381,#27382,#27383));
#6556=EDGE_LOOP('',(#27384,#27385,#27386,#27387));
#6557=EDGE_LOOP('',(#27388,#27389,#27390,#27391));
#6558=EDGE_LOOP('',(#27392,#27393,#27394,#27395));
#6559=EDGE_LOOP('',(#27396,#27397,#27398,#27399));
#6560=EDGE_LOOP('',(#27400,#27401,#27402,#27403,#27404));
#6561=EDGE_LOOP('',(#27405,#27406,#27407,#27408));
#6562=EDGE_LOOP('',(#27409,#27410,#27411,#27412));
#6563=EDGE_LOOP('',(#27413,#27414,#27415,#27416,#27417));
#6564=EDGE_LOOP('',(#27418,#27419,#27420,#27421));
#6565=EDGE_LOOP('',(#27422,#27423,#27424,#27425));
#6566=EDGE_LOOP('',(#27426,#27427,#27428,#27429));
#6567=EDGE_LOOP('',(#27430,#27431,#27432,#27433,#27434));
#6568=EDGE_LOOP('',(#27435,#27436,#27437,#27438,#27439,#27440,#27441,#27442,
#27443,#27444,#27445,#27446,#27447,#27448,#27449,#27450,#27451,#27452,#27453,
#27454,#27455,#27456,#27457,#27458,#27459,#27460,#27461));
#6569=EDGE_LOOP('',(#27462,#27463,#27464,#27465,#27466,#27467));
#6570=EDGE_LOOP('',(#27468,#27469,#27470,#27471,#27472,#27473,#27474,#27475,
#27476,#27477,#27478,#27479,#27480,#27481,#27482,#27483,#27484,#27485,#27486,
#27487,#27488,#27489,#27490,#27491,#27492,#27493));
#6571=EDGE_LOOP('',(#27494,#27495,#27496,#27497,#27498,#27499,#27500,#27501,
#27502,#27503,#27504,#27505,#27506,#27507,#27508,#27509,#27510,#27511,#27512,
#27513,#27514));
#6572=EDGE_LOOP('',(#27515,#27516,#27517,#27518));
#6573=EDGE_LOOP('',(#27519,#27520,#27521,#27522));
#6574=EDGE_LOOP('',(#27523,#27524,#27525,#27526));
#6575=EDGE_LOOP('',(#27527,#27528,#27529,#27530));
#6576=EDGE_LOOP('',(#27531,#27532,#27533,#27534));
#6577=EDGE_LOOP('',(#27535,#27536,#27537,#27538));
#6578=EDGE_LOOP('',(#27539,#27540,#27541,#27542,#27543,#27544,#27545,#27546));
#6579=EDGE_LOOP('',(#27547,#27548,#27549,#27550,#27551,#27552,#27553,#27554));
#6580=EDGE_LOOP('',(#27555,#27556,#27557,#27558,#27559,#27560,#27561,#27562));
#6581=EDGE_LOOP('',(#27563,#27564));
#6582=EDGE_LOOP('',(#27565,#27566));
#6583=EDGE_LOOP('',(#27567,#27568));
#6584=EDGE_LOOP('',(#27569,#27570));
#6585=EDGE_LOOP('',(#27571,#27572));
#6586=EDGE_LOOP('',(#27573,#27574));
#6587=EDGE_LOOP('',(#27575,#27576));
#6588=EDGE_LOOP('',(#27577,#27578));
#6589=EDGE_LOOP('',(#27579,#27580));
#6590=EDGE_LOOP('',(#27581,#27582));
#6591=EDGE_LOOP('',(#27583,#27584));
#6592=EDGE_LOOP('',(#27585,#27586));
#6593=EDGE_LOOP('',(#27587,#27588,#27589,#27590,#27591,#27592,#27593,#27594));
#6594=EDGE_LOOP('',(#27595,#27596,#27597,#27598,#27599,#27600,#27601,#27602));
#6595=EDGE_LOOP('',(#27603,#27604,#27605,#27606,#27607,#27608,#27609,#27610));
#6596=EDGE_LOOP('',(#27611,#27612,#27613,#27614,#27615,#27616,#27617,#27618));
#6597=EDGE_LOOP('',(#27619));
#6598=EDGE_LOOP('',(#27620,#27621,#27622,#27623,#27624,#27625,#27626));
#6599=EDGE_LOOP('',(#27627,#27628,#27629,#27630,#27631,#27632,#27633));
#6600=EDGE_LOOP('',(#27634));
#6601=EDGE_LOOP('',(#27635));
#9266=LINE('',#77157,#12103);
#9267=LINE('',#77253,#12104);
#9268=LINE('',#77643,#12105);
#9269=LINE('',#78042,#12106);
#9270=LINE('',#78422,#12107);
#9271=LINE('',#78777,#12108);
#9272=LINE('',#79143,#12109);
#9273=LINE('',#79502,#12110);
#9274=LINE('',#79886,#12111);
#9275=LINE('',#80256,#12112);
#9276=LINE('',#80489,#12113);
#9277=LINE('',#80835,#12114);
#9278=LINE('',#81169,#12115);
#9279=LINE('',#81506,#12116);
#9280=LINE('',#81844,#12117);
#9281=LINE('',#82194,#12118);
#9282=LINE('',#82543,#12119);
#9283=LINE('',#84080,#12120);
#9284=LINE('',#84084,#12121);
#9285=LINE('',#84086,#12122);
#9286=LINE('',#84090,#12123);
#9287=LINE('',#84093,#12124);
#9288=LINE('',#84096,#12125);
#9289=LINE('',#84098,#12126);
#9290=LINE('',#84102,#12127);
#9291=LINE('',#84105,#12128);
#9292=LINE('',#84108,#12129);
#9293=LINE('',#84110,#12130);
#9294=LINE('',#84114,#12131);
#9295=LINE('',#84117,#12132);
#9296=LINE('',#84119,#12133);
#9297=LINE('',#84121,#12134);
#9298=LINE('',#84123,#12135);
#9299=LINE('',#84124,#12136);
#9300=LINE('',#84126,#12137);
#9301=LINE('',#84128,#12138);
#9302=LINE('',#84129,#12139);
#9303=LINE('',#84131,#12140);
#9304=LINE('',#84133,#12141);
#9305=LINE('',#84134,#12142);
#9306=LINE('',#84138,#12143);
#9307=LINE('',#84141,#12144);
#9308=LINE('',#84143,#12145);
#9309=LINE('',#84147,#12146);
#9310=LINE('',#84150,#12147);
#9311=LINE('',#84159,#12148);
#9312=LINE('',#84163,#12149);
#9313=LINE('',#84165,#12150);
#9314=LINE('',#84166,#12151);
#9315=LINE('',#84173,#12152);
#9316=LINE('',#84176,#12153);
#12103=VECTOR('',#38784,1.4635);
#12104=VECTOR('',#38789,1.4635);
#12105=VECTOR('',#38792,1.4635);
#12106=VECTOR('',#38795,1.4635);
#12107=VECTOR('',#38798,1.4635);
#12108=VECTOR('',#38801,1.4635);
#12109=VECTOR('',#38804,1.4635);
#12110=VECTOR('',#38807,1.4635);
#12111=VECTOR('',#38810,1.4635);
#12112=VECTOR('',#38813,1.17775);
#12113=VECTOR('',#38818,1.17775);
#12114=VECTOR('',#38821,1.17775);
#12115=VECTOR('',#38824,1.17775);
#12116=VECTOR('',#38827,1.17775);
#12117=VECTOR('',#38830,1.17775);
#12118=VECTOR('',#38833,1.17775);
#12119=VECTOR('',#38836,1.17775);
#12120=VECTOR('',#38871,0.916025403784424);
#12121=VECTOR('',#38876,10.);
#12122=VECTOR('',#38877,10.);
#12123=VECTOR('',#38882,10.);
#12124=VECTOR('',#38885,10.);
#12125=VECTOR('',#38888,10.);
#12126=VECTOR('',#38889,10.);
#12127=VECTOR('',#38894,10.);
#12128=VECTOR('',#38897,10.);
#12129=VECTOR('',#38900,10.);
#12130=VECTOR('',#38901,10.);
#12131=VECTOR('',#38906,10.);
#12132=VECTOR('',#38909,10.);
#12133=VECTOR('',#38912,10.);
#12134=VECTOR('',#38913,10.);
#12135=VECTOR('',#38914,10.);
#12136=VECTOR('',#38915,10.);
#12137=VECTOR('',#38918,10.);
#12138=VECTOR('',#38919,10.);
#12139=VECTOR('',#38920,10.);
#12140=VECTOR('',#38923,10.);
#12141=VECTOR('',#38924,10.);
#12142=VECTOR('',#38925,10.);
#12143=VECTOR('',#38932,10.);
#12144=VECTOR('',#38937,10.);
#12145=VECTOR('',#38940,10.);
#12146=VECTOR('',#38943,10.);
#12147=VECTOR('',#38948,10.);
#12148=VECTOR('',#38965,10.);
#12149=VECTOR('',#38970,0.433012701892235);
#12150=VECTOR('',#38973,10.);
#12151=VECTOR('',#38974,10.);
#12152=VECTOR('',#38985,1.25);
#12153=VECTOR('',#38988,1.35);
#12954=CIRCLE('',#33414,1.4635);
#12955=CIRCLE('',#33424,1.17775);
#12956=CIRCLE('',#33433,1.17775);
#12957=CIRCLE('',#33435,1.4635);
#12958=CIRCLE('',#33437,1.4635);
#12959=CIRCLE('',#33438,1.4635);
#12960=CIRCLE('',#33440,1.4635);
#12961=CIRCLE('',#33441,1.4635);
#12962=CIRCLE('',#33443,0.816025403784426);
#12963=CIRCLE('',#33444,0.816025403784426);
#12964=CIRCLE('',#33445,0.816025403784426);
#12965=CIRCLE('',#33446,0.816025403784426);
#12966=CIRCLE('',#33447,0.816025403784426);
#12967=CIRCLE('',#33448,0.816025403784426);
#12968=CIRCLE('',#33449,1.01602540378442);
#12969=CIRCLE('',#33451,0.816025403784426);
#12970=CIRCLE('',#33453,0.816025403784426);
#12971=CIRCLE('',#33455,0.816025403784426);
#12972=CIRCLE('',#33457,0.816025403784426);
#12973=CIRCLE('',#33459,0.816025403784426);
#12974=CIRCLE('',#33461,0.816025403784426);
#12975=CIRCLE('',#33472,0.866025403784452);
#12976=CIRCLE('',#33474,0.866025403784452);
#12977=CIRCLE('',#33476,0.866025403784452);
#12978=CIRCLE('',#33478,0.866025403784452);
#12979=CIRCLE('',#33480,0.866025403784452);
#12980=CIRCLE('',#33482,0.866025403784452);
#12981=CIRCLE('',#33488,0.999999999999996);
#12982=CIRCLE('',#33491,1.19999999999999);
#15369=VERTEX_POINT('',#77155);
#15370=VERTEX_POINT('',#77156);
#15371=VERTEX_POINT('',#77158);
#15372=VERTEX_POINT('',#77217);
#15373=VERTEX_POINT('',#77251);
#15374=VERTEX_POINT('',#77252);
#15375=VERTEX_POINT('',#77641);
#15376=VERTEX_POINT('',#77642);
#15377=VERTEX_POINT('',#78040);
#15378=VERTEX_POINT('',#78041);
#15379=VERTEX_POINT('',#78043);
#15380=VERTEX_POINT('',#78228);
#15381=VERTEX_POINT('',#78420);
#15382=VERTEX_POINT('',#78421);
#15383=VERTEX_POINT('',#78423);
#15384=VERTEX_POINT('',#78775);
#15385=VERTEX_POINT('',#78776);
#15386=VERTEX_POINT('',#79141);
#15387=VERTEX_POINT('',#79142);
#15388=VERTEX_POINT('',#79320);
#15389=VERTEX_POINT('',#79500);
#15390=VERTEX_POINT('',#79501);
#15391=VERTEX_POINT('',#79503);
#15392=VERTEX_POINT('',#79692);
#15393=VERTEX_POINT('',#79884);
#15394=VERTEX_POINT('',#79885);
#15395=VERTEX_POINT('',#80254);
#15396=VERTEX_POINT('',#80255);
#15397=VERTEX_POINT('',#80257);
#15398=VERTEX_POINT('',#80388);
#15399=VERTEX_POINT('',#80487);
#15400=VERTEX_POINT('',#80488);
#15401=VERTEX_POINT('',#80833);
#15402=VERTEX_POINT('',#80834);
#15403=VERTEX_POINT('',#81167);
#15404=VERTEX_POINT('',#81168);
#15405=VERTEX_POINT('',#81170);
#15406=VERTEX_POINT('',#81504);
#15407=VERTEX_POINT('',#81505);
#15408=VERTEX_POINT('',#81842);
#15409=VERTEX_POINT('',#81843);
#15410=VERTEX_POINT('',#82192);
#15411=VERTEX_POINT('',#82193);
#15412=VERTEX_POINT('',#82363);
#15413=VERTEX_POINT('',#82541);
#15414=VERTEX_POINT('',#82542);
#15415=VERTEX_POINT('',#82869);
#15416=VERTEX_POINT('',#83026);
#15417=VERTEX_POINT('',#83151);
#15418=VERTEX_POINT('',#83214);
#15419=VERTEX_POINT('',#83257);
#15420=VERTEX_POINT('',#83258);
#15421=VERTEX_POINT('',#83599);
#15422=VERTEX_POINT('',#83690);
#15423=VERTEX_POINT('',#83692);
#15424=VERTEX_POINT('',#84019);
#15425=VERTEX_POINT('',#84020);
#15426=VERTEX_POINT('',#84024);
#15427=VERTEX_POINT('',#84026);
#15428=VERTEX_POINT('',#84030);
#15429=VERTEX_POINT('',#84034);
#15430=VERTEX_POINT('',#84036);
#15431=VERTEX_POINT('',#84040);
#15432=VERTEX_POINT('',#84044);
#15433=VERTEX_POINT('',#84046);
#15434=VERTEX_POINT('',#84050);
#15435=VERTEX_POINT('',#84054);
#15436=VERTEX_POINT('',#84056);
#15437=VERTEX_POINT('',#84060);
#15438=VERTEX_POINT('',#84064);
#15439=VERTEX_POINT('',#84066);
#15440=VERTEX_POINT('',#84070);
#15441=VERTEX_POINT('',#84074);
#15442=VERTEX_POINT('',#84079);
#15443=VERTEX_POINT('',#84083);
#15444=VERTEX_POINT('',#84085);
#15445=VERTEX_POINT('',#84089);
#15446=VERTEX_POINT('',#84091);
#15447=VERTEX_POINT('',#84095);
#15448=VERTEX_POINT('',#84097);
#15449=VERTEX_POINT('',#84101);
#15450=VERTEX_POINT('',#84103);
#15451=VERTEX_POINT('',#84107);
#15452=VERTEX_POINT('',#84109);
#15453=VERTEX_POINT('',#84113);
#15454=VERTEX_POINT('',#84115);
#15455=VERTEX_POINT('',#84120);
#15456=VERTEX_POINT('',#84122);
#15457=VERTEX_POINT('',#84127);
#15458=VERTEX_POINT('',#84132);
#15459=VERTEX_POINT('',#84145);
#15460=VERTEX_POINT('',#84146);
#15461=VERTEX_POINT('',#84162);
#15462=VERTEX_POINT('',#84170);
#15463=VERTEX_POINT('',#84175);
#19524=EDGE_CURVE('',#15369,#15370,#9266,.T.);
#19525=EDGE_CURVE('',#15369,#15371,#1376,.F.);
#19526=EDGE_CURVE('',#15371,#15372,#12954,.T.);
#19527=EDGE_CURVE('',#15372,#15370,#1377,.T.);
#19528=EDGE_CURVE('',#15373,#15374,#9267,.T.);
#19529=EDGE_CURVE('',#15373,#15369,#1378,.F.);
#19530=EDGE_CURVE('',#15370,#15374,#1379,.T.);
#19531=EDGE_CURVE('',#15375,#15376,#9268,.T.);
#19532=EDGE_CURVE('',#15375,#15373,#1380,.T.);
#19533=EDGE_CURVE('',#15374,#15376,#1381,.T.);
#19534=EDGE_CURVE('',#15377,#15378,#9269,.T.);
#19535=EDGE_CURVE('',#15377,#15379,#1382,.T.);
#19536=EDGE_CURVE('',#15379,#15375,#1383,.T.);
#19537=EDGE_CURVE('',#15376,#15380,#1384,.T.);
#19538=EDGE_CURVE('',#15380,#15378,#1385,.T.);
#19539=EDGE_CURVE('',#15381,#15382,#9270,.T.);
#19540=EDGE_CURVE('',#15381,#15383,#1386,.T.);
#19541=EDGE_CURVE('',#15383,#15377,#1387,.T.);
#19542=EDGE_CURVE('',#15378,#15382,#1388,.T.);
#19543=EDGE_CURVE('',#15384,#15385,#9271,.T.);
#19544=EDGE_CURVE('',#15384,#15381,#1389,.T.);
#19545=EDGE_CURVE('',#15382,#15385,#1390,.T.);
#19546=EDGE_CURVE('',#15386,#15387,#9272,.T.);
#19547=EDGE_CURVE('',#15386,#15384,#1391,.T.);
#19548=EDGE_CURVE('',#15385,#15388,#1392,.T.);
#19549=EDGE_CURVE('',#15388,#15387,#1393,.T.);
#19550=EDGE_CURVE('',#15389,#15390,#9273,.T.);
#19551=EDGE_CURVE('',#15389,#15391,#1394,.T.);
#19552=EDGE_CURVE('',#15391,#15386,#1395,.T.);
#19553=EDGE_CURVE('',#15387,#15392,#1396,.T.);
#19554=EDGE_CURVE('',#15392,#15390,#1397,.T.);
#19555=EDGE_CURVE('',#15393,#15394,#9274,.T.);
#19556=EDGE_CURVE('',#15393,#15389,#1398,.T.);
#19557=EDGE_CURVE('',#15390,#15394,#1399,.T.);
#19558=EDGE_CURVE('',#15395,#15396,#9275,.T.);
#19559=EDGE_CURVE('',#15397,#15395,#1400,.F.);
#19560=EDGE_CURVE('',#15398,#15397,#12955,.T.);
#19561=EDGE_CURVE('',#15398,#15396,#1401,.T.);
#19562=EDGE_CURVE('',#15399,#15400,#9276,.T.);
#19563=EDGE_CURVE('',#15395,#15399,#1402,.F.);
#19564=EDGE_CURVE('',#15396,#15400,#1403,.T.);
#19565=EDGE_CURVE('',#15401,#15402,#9277,.T.);
#19566=EDGE_CURVE('',#15399,#15401,#1404,.F.);
#19567=EDGE_CURVE('',#15400,#15402,#1405,.T.);
#19568=EDGE_CURVE('',#15403,#15404,#9278,.T.);
#19569=EDGE_CURVE('',#15405,#15403,#1406,.F.);
#19570=EDGE_CURVE('',#15401,#15405,#1407,.F.);
#19571=EDGE_CURVE('',#15402,#15404,#1408,.T.);
#19572=EDGE_CURVE('',#15406,#15407,#9279,.T.);
#19573=EDGE_CURVE('',#15403,#15406,#1409,.F.);
#19574=EDGE_CURVE('',#15404,#15407,#1410,.T.);
#19575=EDGE_CURVE('',#15408,#15409,#9280,.T.);
#19576=EDGE_CURVE('',#15406,#15408,#1411,.F.);
#19577=EDGE_CURVE('',#15407,#15409,#1412,.T.);
#19578=EDGE_CURVE('',#15410,#15411,#9281,.T.);
#19579=EDGE_CURVE('',#15408,#15410,#1413,.F.);
#19580=EDGE_CURVE('',#15409,#15412,#1414,.T.);
#19581=EDGE_CURVE('',#15412,#15411,#1415,.T.);
#19582=EDGE_CURVE('',#15413,#15414,#9282,.T.);
#19583=EDGE_CURVE('',#15410,#15413,#1416,.F.);
#19584=EDGE_CURVE('',#15411,#15414,#1417,.T.);
#19585=EDGE_CURVE('',#15414,#15415,#1418,.T.);
#19586=EDGE_CURVE('',#15416,#15415,#12956,.T.);
#19587=EDGE_CURVE('',#15413,#15416,#1419,.F.);
#19588=EDGE_CURVE('',#15394,#15417,#1420,.T.);
#19589=EDGE_CURVE('',#15418,#15417,#12957,.F.);
#19590=EDGE_CURVE('',#15418,#15393,#1421,.T.);
#19591=EDGE_CURVE('',#15419,#15420,#12958,.F.);
#19592=EDGE_CURVE('',#15419,#15416,#1422,.T.);
#19593=EDGE_CURVE('',#15415,#15418,#1423,.T.);
#19594=EDGE_CURVE('',#15420,#15418,#12959,.F.);
#19595=EDGE_CURVE('',#15417,#15419,#1424,.T.);
#19596=EDGE_CURVE('',#15421,#15372,#1425,.T.);
#19597=EDGE_CURVE('',#15421,#15397,#1426,.T.);
#19598=EDGE_CURVE('',#15372,#15422,#12960,.T.);
#19599=EDGE_CURVE('',#15422,#15423,#12961,.T.);
#19600=EDGE_CURVE('',#15423,#15398,#1427,.T.);
#19601=EDGE_CURVE('',#15423,#15371,#1428,.T.);
#19602=EDGE_CURVE('',#15424,#15425,#104,.T.);
#19603=EDGE_CURVE('',#15426,#15424,#12962,.T.);
#19604=EDGE_CURVE('',#15427,#15426,#105,.T.);
#19605=EDGE_CURVE('',#15428,#15427,#106,.T.);
#19606=EDGE_CURVE('',#15429,#15428,#12963,.T.);
#19607=EDGE_CURVE('',#15430,#15429,#107,.T.);
#19608=EDGE_CURVE('',#15431,#15430,#108,.T.);
#19609=EDGE_CURVE('',#15432,#15431,#12964,.T.);
#19610=EDGE_CURVE('',#15433,#15432,#109,.T.);
#19611=EDGE_CURVE('',#15434,#15433,#110,.T.);
#19612=EDGE_CURVE('',#15435,#15434,#12965,.T.);
#19613=EDGE_CURVE('',#15436,#15435,#111,.T.);
#19614=EDGE_CURVE('',#15437,#15436,#112,.T.);
#19615=EDGE_CURVE('',#15438,#15437,#12966,.T.);
#19616=EDGE_CURVE('',#15439,#15438,#113,.T.);
#19617=EDGE_CURVE('',#15440,#15439,#114,.T.);
#19618=EDGE_CURVE('',#15441,#15440,#12967,.T.);
#19619=EDGE_CURVE('',#15425,#15441,#115,.T.);
#19620=EDGE_CURVE('',#15425,#15442,#9283,.T.);
#19621=EDGE_CURVE('',#15442,#15442,#12968,.T.);
#19622=EDGE_CURVE('',#15438,#15443,#9284,.T.);
#19623=EDGE_CURVE('',#15444,#15437,#9285,.T.);
#19624=EDGE_CURVE('',#15443,#15444,#12969,.T.);
#19625=EDGE_CURVE('',#15445,#15434,#9286,.T.);
#19626=EDGE_CURVE('',#15446,#15445,#12970,.T.);
#19627=EDGE_CURVE('',#15435,#15446,#9287,.T.);
#19628=EDGE_CURVE('',#15441,#15447,#9288,.T.);
#19629=EDGE_CURVE('',#15448,#15440,#9289,.T.);
#19630=EDGE_CURVE('',#15447,#15448,#12971,.T.);
#19631=EDGE_CURVE('',#15449,#15431,#9290,.T.);
#19632=EDGE_CURVE('',#15450,#15449,#12972,.T.);
#19633=EDGE_CURVE('',#15432,#15450,#9291,.T.);
#19634=EDGE_CURVE('',#15426,#15451,#9292,.T.);
#19635=EDGE_CURVE('',#15452,#15424,#9293,.T.);
#19636=EDGE_CURVE('',#15451,#15452,#12973,.T.);
#19637=EDGE_CURVE('',#15453,#15428,#9294,.T.);
#19638=EDGE_CURVE('',#15454,#15453,#12974,.T.);
#19639=EDGE_CURVE('',#15429,#15454,#9295,.T.);
#19640=EDGE_CURVE('',#15452,#15451,#9296,.T.);
#19641=EDGE_CURVE('',#15425,#15455,#9297,.T.);
#19642=EDGE_CURVE('',#15455,#15456,#9298,.T.);
#19643=EDGE_CURVE('',#15427,#15456,#9299,.T.);
#19644=EDGE_CURVE('',#15448,#15447,#9300,.T.);
#19645=EDGE_CURVE('',#15439,#15457,#9301,.T.);
#19646=EDGE_CURVE('',#15457,#15455,#9302,.T.);
#19647=EDGE_CURVE('',#15444,#15443,#9303,.T.);
#19648=EDGE_CURVE('',#15436,#15458,#9304,.T.);
#19649=EDGE_CURVE('',#15458,#15457,#9305,.T.);
#19650=EDGE_CURVE('',#15445,#15446,#9306,.T.);
#19651=EDGE_CURVE('',#15449,#15450,#9307,.T.);
#19652=EDGE_CURVE('',#15453,#15454,#9308,.T.);
#19653=EDGE_CURVE('',#15459,#15460,#9309,.T.);
#19654=EDGE_CURVE('',#15460,#15459,#12975,.T.);
#19655=EDGE_CURVE('',#15460,#15458,#9310,.T.);
#19656=EDGE_CURVE('',#15458,#15460,#12976,.T.);
#19657=EDGE_CURVE('',#15457,#15458,#12977,.T.);
#19658=EDGE_CURVE('',#15455,#15457,#12978,.T.);
#19659=EDGE_CURVE('',#15456,#15455,#12979,.T.);
#19660=EDGE_CURVE('',#15456,#15459,#9311,.T.);
#19661=EDGE_CURVE('',#15459,#15456,#12980,.T.);
#19662=EDGE_CURVE('',#15461,#15455,#9312,.T.);
#19663=EDGE_CURVE('',#15430,#15459,#9313,.T.);
#19664=EDGE_CURVE('',#15433,#15460,#9314,.T.);
#19665=EDGE_CURVE('',#15462,#15462,#12981,.T.);
#19666=EDGE_CURVE('',#15422,#15462,#9315,.T.);
#19667=EDGE_CURVE('',#15420,#15463,#9316,.T.);
#19668=EDGE_CURVE('',#15463,#15463,#12982,.T.);
#27346=ORIENTED_EDGE('',*,*,#19524,.F.);
#27347=ORIENTED_EDGE('',*,*,#19525,.T.);
#27348=ORIENTED_EDGE('',*,*,#19526,.T.);
#27349=ORIENTED_EDGE('',*,*,#19527,.T.);
#27350=ORIENTED_EDGE('',*,*,#19528,.F.);
#27351=ORIENTED_EDGE('',*,*,#19529,.T.);
#27352=ORIENTED_EDGE('',*,*,#19524,.T.);
#27353=ORIENTED_EDGE('',*,*,#19530,.T.);
#27354=ORIENTED_EDGE('',*,*,#19531,.F.);
#27355=ORIENTED_EDGE('',*,*,#19532,.T.);
#27356=ORIENTED_EDGE('',*,*,#19528,.T.);
#27357=ORIENTED_EDGE('',*,*,#19533,.T.);
#27358=ORIENTED_EDGE('',*,*,#19534,.F.);
#27359=ORIENTED_EDGE('',*,*,#19535,.T.);
#27360=ORIENTED_EDGE('',*,*,#19536,.T.);
#27361=ORIENTED_EDGE('',*,*,#19531,.T.);
#27362=ORIENTED_EDGE('',*,*,#19537,.T.);
#27363=ORIENTED_EDGE('',*,*,#19538,.T.);
#27364=ORIENTED_EDGE('',*,*,#19539,.F.);
#27365=ORIENTED_EDGE('',*,*,#19540,.T.);
#27366=ORIENTED_EDGE('',*,*,#19541,.T.);
#27367=ORIENTED_EDGE('',*,*,#19534,.T.);
#27368=ORIENTED_EDGE('',*,*,#19542,.T.);
#27369=ORIENTED_EDGE('',*,*,#19543,.F.);
#27370=ORIENTED_EDGE('',*,*,#19544,.T.);
#27371=ORIENTED_EDGE('',*,*,#19539,.T.);
#27372=ORIENTED_EDGE('',*,*,#19545,.T.);
#27373=ORIENTED_EDGE('',*,*,#19546,.F.);
#27374=ORIENTED_EDGE('',*,*,#19547,.T.);
#27375=ORIENTED_EDGE('',*,*,#19543,.T.);
#27376=ORIENTED_EDGE('',*,*,#19548,.T.);
#27377=ORIENTED_EDGE('',*,*,#19549,.T.);
#27378=ORIENTED_EDGE('',*,*,#19550,.F.);
#27379=ORIENTED_EDGE('',*,*,#19551,.T.);
#27380=ORIENTED_EDGE('',*,*,#19552,.T.);
#27381=ORIENTED_EDGE('',*,*,#19546,.T.);
#27382=ORIENTED_EDGE('',*,*,#19553,.T.);
#27383=ORIENTED_EDGE('',*,*,#19554,.T.);
#27384=ORIENTED_EDGE('',*,*,#19555,.F.);
#27385=ORIENTED_EDGE('',*,*,#19556,.T.);
#27386=ORIENTED_EDGE('',*,*,#19550,.T.);
#27387=ORIENTED_EDGE('',*,*,#19557,.T.);
#27388=ORIENTED_EDGE('',*,*,#19558,.F.);
#27389=ORIENTED_EDGE('',*,*,#19559,.F.);
#27390=ORIENTED_EDGE('',*,*,#19560,.F.);
#27391=ORIENTED_EDGE('',*,*,#19561,.T.);
#27392=ORIENTED_EDGE('',*,*,#19562,.F.);
#27393=ORIENTED_EDGE('',*,*,#19563,.F.);
#27394=ORIENTED_EDGE('',*,*,#19558,.T.);
#27395=ORIENTED_EDGE('',*,*,#19564,.T.);
#27396=ORIENTED_EDGE('',*,*,#19565,.F.);
#27397=ORIENTED_EDGE('',*,*,#19566,.F.);
#27398=ORIENTED_EDGE('',*,*,#19562,.T.);
#27399=ORIENTED_EDGE('',*,*,#19567,.T.);
#27400=ORIENTED_EDGE('',*,*,#19568,.F.);
#27401=ORIENTED_EDGE('',*,*,#19569,.F.);
#27402=ORIENTED_EDGE('',*,*,#19570,.F.);
#27403=ORIENTED_EDGE('',*,*,#19565,.T.);
#27404=ORIENTED_EDGE('',*,*,#19571,.T.);
#27405=ORIENTED_EDGE('',*,*,#19572,.F.);
#27406=ORIENTED_EDGE('',*,*,#19573,.F.);
#27407=ORIENTED_EDGE('',*,*,#19568,.T.);
#27408=ORIENTED_EDGE('',*,*,#19574,.T.);
#27409=ORIENTED_EDGE('',*,*,#19575,.F.);
#27410=ORIENTED_EDGE('',*,*,#19576,.F.);
#27411=ORIENTED_EDGE('',*,*,#19572,.T.);
#27412=ORIENTED_EDGE('',*,*,#19577,.T.);
#27413=ORIENTED_EDGE('',*,*,#19578,.F.);
#27414=ORIENTED_EDGE('',*,*,#19579,.F.);
#27415=ORIENTED_EDGE('',*,*,#19575,.T.);
#27416=ORIENTED_EDGE('',*,*,#19580,.T.);
#27417=ORIENTED_EDGE('',*,*,#19581,.T.);
#27418=ORIENTED_EDGE('',*,*,#19582,.F.);
#27419=ORIENTED_EDGE('',*,*,#19583,.F.);
#27420=ORIENTED_EDGE('',*,*,#19578,.T.);
#27421=ORIENTED_EDGE('',*,*,#19584,.T.);
#27422=ORIENTED_EDGE('',*,*,#19582,.T.);
#27423=ORIENTED_EDGE('',*,*,#19585,.T.);
#27424=ORIENTED_EDGE('',*,*,#19586,.F.);
#27425=ORIENTED_EDGE('',*,*,#19587,.F.);
#27426=ORIENTED_EDGE('',*,*,#19555,.T.);
#27427=ORIENTED_EDGE('',*,*,#19588,.T.);
#27428=ORIENTED_EDGE('',*,*,#19589,.F.);
#27429=ORIENTED_EDGE('',*,*,#19590,.T.);
#27430=ORIENTED_EDGE('',*,*,#19591,.F.);
#27431=ORIENTED_EDGE('',*,*,#19592,.T.);
#27432=ORIENTED_EDGE('',*,*,#19586,.T.);
#27433=ORIENTED_EDGE('',*,*,#19593,.T.);
#27434=ORIENTED_EDGE('',*,*,#19594,.F.);
#27435=ORIENTED_EDGE('',*,*,#19592,.F.);
#27436=ORIENTED_EDGE('',*,*,#19595,.F.);
#27437=ORIENTED_EDGE('',*,*,#19588,.F.);
#27438=ORIENTED_EDGE('',*,*,#19557,.F.);
#27439=ORIENTED_EDGE('',*,*,#19554,.F.);
#27440=ORIENTED_EDGE('',*,*,#19553,.F.);
#27441=ORIENTED_EDGE('',*,*,#19549,.F.);
#27442=ORIENTED_EDGE('',*,*,#19548,.F.);
#27443=ORIENTED_EDGE('',*,*,#19545,.F.);
#27444=ORIENTED_EDGE('',*,*,#19542,.F.);
#27445=ORIENTED_EDGE('',*,*,#19538,.F.);
#27446=ORIENTED_EDGE('',*,*,#19537,.F.);
#27447=ORIENTED_EDGE('',*,*,#19533,.F.);
#27448=ORIENTED_EDGE('',*,*,#19530,.F.);
#27449=ORIENTED_EDGE('',*,*,#19527,.F.);
#27450=ORIENTED_EDGE('',*,*,#19596,.F.);
#27451=ORIENTED_EDGE('',*,*,#19597,.T.);
#27452=ORIENTED_EDGE('',*,*,#19559,.T.);
#27453=ORIENTED_EDGE('',*,*,#19563,.T.);
#27454=ORIENTED_EDGE('',*,*,#19566,.T.);
#27455=ORIENTED_EDGE('',*,*,#19570,.T.);
#27456=ORIENTED_EDGE('',*,*,#19569,.T.);
#27457=ORIENTED_EDGE('',*,*,#19573,.T.);
#27458=ORIENTED_EDGE('',*,*,#19576,.T.);
#27459=ORIENTED_EDGE('',*,*,#19579,.T.);
#27460=ORIENTED_EDGE('',*,*,#19583,.T.);
#27461=ORIENTED_EDGE('',*,*,#19587,.T.);
#27462=ORIENTED_EDGE('',*,*,#19598,.T.);
#27463=ORIENTED_EDGE('',*,*,#19599,.T.);
#27464=ORIENTED_EDGE('',*,*,#19600,.T.);
#27465=ORIENTED_EDGE('',*,*,#19560,.T.);
#27466=ORIENTED_EDGE('',*,*,#19597,.F.);
#27467=ORIENTED_EDGE('',*,*,#19596,.T.);
#27468=ORIENTED_EDGE('',*,*,#19593,.F.);
#27469=ORIENTED_EDGE('',*,*,#19585,.F.);
#27470=ORIENTED_EDGE('',*,*,#19584,.F.);
#27471=ORIENTED_EDGE('',*,*,#19581,.F.);
#27472=ORIENTED_EDGE('',*,*,#19580,.F.);
#27473=ORIENTED_EDGE('',*,*,#19577,.F.);
#27474=ORIENTED_EDGE('',*,*,#19574,.F.);
#27475=ORIENTED_EDGE('',*,*,#19571,.F.);
#27476=ORIENTED_EDGE('',*,*,#19567,.F.);
#27477=ORIENTED_EDGE('',*,*,#19564,.F.);
#27478=ORIENTED_EDGE('',*,*,#19561,.F.);
#27479=ORIENTED_EDGE('',*,*,#19600,.F.);
#27480=ORIENTED_EDGE('',*,*,#19601,.T.);
#27481=ORIENTED_EDGE('',*,*,#19525,.F.);
#27482=ORIENTED_EDGE('',*,*,#19529,.F.);
#27483=ORIENTED_EDGE('',*,*,#19532,.F.);
#27484=ORIENTED_EDGE('',*,*,#19536,.F.);
#27485=ORIENTED_EDGE('',*,*,#19535,.F.);
#27486=ORIENTED_EDGE('',*,*,#19541,.F.);
#27487=ORIENTED_EDGE('',*,*,#19540,.F.);
#27488=ORIENTED_EDGE('',*,*,#19544,.F.);
#27489=ORIENTED_EDGE('',*,*,#19547,.F.);
#27490=ORIENTED_EDGE('',*,*,#19552,.F.);
#27491=ORIENTED_EDGE('',*,*,#19551,.F.);
#27492=ORIENTED_EDGE('',*,*,#19556,.F.);
#27493=ORIENTED_EDGE('',*,*,#19590,.F.);
#27494=ORIENTED_EDGE('',*,*,#19602,.F.);
#27495=ORIENTED_EDGE('',*,*,#19603,.F.);
#27496=ORIENTED_EDGE('',*,*,#19604,.F.);
#27497=ORIENTED_EDGE('',*,*,#19605,.F.);
#27498=ORIENTED_EDGE('',*,*,#19606,.F.);
#27499=ORIENTED_EDGE('',*,*,#19607,.F.);
#27500=ORIENTED_EDGE('',*,*,#19608,.F.);
#27501=ORIENTED_EDGE('',*,*,#19609,.F.);
#27502=ORIENTED_EDGE('',*,*,#19610,.F.);
#27503=ORIENTED_EDGE('',*,*,#19611,.F.);
#27504=ORIENTED_EDGE('',*,*,#19612,.F.);
#27505=ORIENTED_EDGE('',*,*,#19613,.F.);
#27506=ORIENTED_EDGE('',*,*,#19614,.F.);
#27507=ORIENTED_EDGE('',*,*,#19615,.F.);
#27508=ORIENTED_EDGE('',*,*,#19616,.F.);
#27509=ORIENTED_EDGE('',*,*,#19617,.F.);
#27510=ORIENTED_EDGE('',*,*,#19618,.F.);
#27511=ORIENTED_EDGE('',*,*,#19619,.F.);
#27512=ORIENTED_EDGE('',*,*,#19620,.T.);
#27513=ORIENTED_EDGE('',*,*,#19621,.F.);
#27514=ORIENTED_EDGE('',*,*,#19620,.F.);
#27515=ORIENTED_EDGE('',*,*,#19622,.F.);
#27516=ORIENTED_EDGE('',*,*,#19615,.T.);
#27517=ORIENTED_EDGE('',*,*,#19623,.F.);
#27518=ORIENTED_EDGE('',*,*,#19624,.F.);
#27519=ORIENTED_EDGE('',*,*,#19625,.F.);
#27520=ORIENTED_EDGE('',*,*,#19626,.F.);
#27521=ORIENTED_EDGE('',*,*,#19627,.F.);
#27522=ORIENTED_EDGE('',*,*,#19612,.T.);
#27523=ORIENTED_EDGE('',*,*,#19628,.F.);
#27524=ORIENTED_EDGE('',*,*,#19618,.T.);
#27525=ORIENTED_EDGE('',*,*,#19629,.F.);
#27526=ORIENTED_EDGE('',*,*,#19630,.F.);
#27527=ORIENTED_EDGE('',*,*,#19631,.F.);
#27528=ORIENTED_EDGE('',*,*,#19632,.F.);
#27529=ORIENTED_EDGE('',*,*,#19633,.F.);
#27530=ORIENTED_EDGE('',*,*,#19609,.T.);
#27531=ORIENTED_EDGE('',*,*,#19634,.F.);
#27532=ORIENTED_EDGE('',*,*,#19603,.T.);
#27533=ORIENTED_EDGE('',*,*,#19635,.F.);
#27534=ORIENTED_EDGE('',*,*,#19636,.F.);
#27535=ORIENTED_EDGE('',*,*,#19637,.F.);
#27536=ORIENTED_EDGE('',*,*,#19638,.F.);
#27537=ORIENTED_EDGE('',*,*,#19639,.F.);
#27538=ORIENTED_EDGE('',*,*,#19606,.T.);
#27539=ORIENTED_EDGE('',*,*,#19604,.T.);
#27540=ORIENTED_EDGE('',*,*,#19634,.T.);
#27541=ORIENTED_EDGE('',*,*,#19640,.F.);
#27542=ORIENTED_EDGE('',*,*,#19635,.T.);
#27543=ORIENTED_EDGE('',*,*,#19602,.T.);
#27544=ORIENTED_EDGE('',*,*,#19641,.T.);
#27545=ORIENTED_EDGE('',*,*,#19642,.T.);
#27546=ORIENTED_EDGE('',*,*,#19643,.F.);
#27547=ORIENTED_EDGE('',*,*,#19619,.T.);
#27548=ORIENTED_EDGE('',*,*,#19628,.T.);
#27549=ORIENTED_EDGE('',*,*,#19644,.F.);
#27550=ORIENTED_EDGE('',*,*,#19629,.T.);
#27551=ORIENTED_EDGE('',*,*,#19617,.T.);
#27552=ORIENTED_EDGE('',*,*,#19645,.T.);
#27553=ORIENTED_EDGE('',*,*,#19646,.T.);
#27554=ORIENTED_EDGE('',*,*,#19641,.F.);
#27555=ORIENTED_EDGE('',*,*,#19616,.T.);
#27556=ORIENTED_EDGE('',*,*,#19622,.T.);
#27557=ORIENTED_EDGE('',*,*,#19647,.F.);
#27558=ORIENTED_EDGE('',*,*,#19623,.T.);
#27559=ORIENTED_EDGE('',*,*,#19614,.T.);
#27560=ORIENTED_EDGE('',*,*,#19648,.T.);
#27561=ORIENTED_EDGE('',*,*,#19649,.T.);
#27562=ORIENTED_EDGE('',*,*,#19645,.F.);
#27563=ORIENTED_EDGE('',*,*,#19624,.T.);
#27564=ORIENTED_EDGE('',*,*,#19647,.T.);
#27565=ORIENTED_EDGE('',*,*,#19630,.T.);
#27566=ORIENTED_EDGE('',*,*,#19644,.T.);
#27567=ORIENTED_EDGE('',*,*,#19626,.T.);
#27568=ORIENTED_EDGE('',*,*,#19650,.T.);
#27569=ORIENTED_EDGE('',*,*,#19636,.T.);
#27570=ORIENTED_EDGE('',*,*,#19640,.T.);
#27571=ORIENTED_EDGE('',*,*,#19632,.T.);
#27572=ORIENTED_EDGE('',*,*,#19651,.T.);
#27573=ORIENTED_EDGE('',*,*,#19638,.T.);
#27574=ORIENTED_EDGE('',*,*,#19652,.T.);
#27575=ORIENTED_EDGE('',*,*,#19653,.F.);
#27576=ORIENTED_EDGE('',*,*,#19654,.F.);
#27577=ORIENTED_EDGE('',*,*,#19655,.F.);
#27578=ORIENTED_EDGE('',*,*,#19656,.F.);
#27579=ORIENTED_EDGE('',*,*,#19649,.F.);
#27580=ORIENTED_EDGE('',*,*,#19657,.F.);
#27581=ORIENTED_EDGE('',*,*,#19646,.F.);
#27582=ORIENTED_EDGE('',*,*,#19658,.F.);
#27583=ORIENTED_EDGE('',*,*,#19642,.F.);
#27584=ORIENTED_EDGE('',*,*,#19659,.F.);
#27585=ORIENTED_EDGE('',*,*,#19660,.F.);
#27586=ORIENTED_EDGE('',*,*,#19661,.F.);
#27587=ORIENTED_EDGE('',*,*,#19662,.T.);
#27588=ORIENTED_EDGE('',*,*,#19658,.T.);
#27589=ORIENTED_EDGE('',*,*,#19657,.T.);
#27590=ORIENTED_EDGE('',*,*,#19656,.T.);
#27591=ORIENTED_EDGE('',*,*,#19654,.T.);
#27592=ORIENTED_EDGE('',*,*,#19661,.T.);
#27593=ORIENTED_EDGE('',*,*,#19659,.T.);
#27594=ORIENTED_EDGE('',*,*,#19662,.F.);
#27595=ORIENTED_EDGE('',*,*,#19608,.T.);
#27596=ORIENTED_EDGE('',*,*,#19663,.T.);
#27597=ORIENTED_EDGE('',*,*,#19653,.T.);
#27598=ORIENTED_EDGE('',*,*,#19664,.F.);
#27599=ORIENTED_EDGE('',*,*,#19610,.T.);
#27600=ORIENTED_EDGE('',*,*,#19633,.T.);
#27601=ORIENTED_EDGE('',*,*,#19651,.F.);
#27602=ORIENTED_EDGE('',*,*,#19631,.T.);
#27603=ORIENTED_EDGE('',*,*,#19605,.T.);
#27604=ORIENTED_EDGE('',*,*,#19643,.T.);
#27605=ORIENTED_EDGE('',*,*,#19660,.T.);
#27606=ORIENTED_EDGE('',*,*,#19663,.F.);
#27607=ORIENTED_EDGE('',*,*,#19607,.T.);
#27608=ORIENTED_EDGE('',*,*,#19639,.T.);
#27609=ORIENTED_EDGE('',*,*,#19652,.F.);
#27610=ORIENTED_EDGE('',*,*,#19637,.T.);
#27611=ORIENTED_EDGE('',*,*,#19611,.T.);
#27612=ORIENTED_EDGE('',*,*,#19664,.T.);
#27613=ORIENTED_EDGE('',*,*,#19655,.T.);
#27614=ORIENTED_EDGE('',*,*,#19648,.F.);
#27615=ORIENTED_EDGE('',*,*,#19613,.T.);
#27616=ORIENTED_EDGE('',*,*,#19627,.T.);
#27617=ORIENTED_EDGE('',*,*,#19650,.F.);
#27618=ORIENTED_EDGE('',*,*,#19625,.T.);
#27619=ORIENTED_EDGE('',*,*,#19665,.F.);
#27620=ORIENTED_EDGE('',*,*,#19598,.F.);
#27621=ORIENTED_EDGE('',*,*,#19526,.F.);
#27622=ORIENTED_EDGE('',*,*,#19601,.F.);
#27623=ORIENTED_EDGE('',*,*,#19599,.F.);
#27624=ORIENTED_EDGE('',*,*,#19666,.T.);
#27625=ORIENTED_EDGE('',*,*,#19665,.T.);
#27626=ORIENTED_EDGE('',*,*,#19666,.F.);
#27627=ORIENTED_EDGE('',*,*,#19591,.T.);
#27628=ORIENTED_EDGE('',*,*,#19667,.T.);
#27629=ORIENTED_EDGE('',*,*,#19668,.F.);
#27630=ORIENTED_EDGE('',*,*,#19667,.F.);
#27631=ORIENTED_EDGE('',*,*,#19594,.T.);
#27632=ORIENTED_EDGE('',*,*,#19589,.T.);
#27633=ORIENTED_EDGE('',*,*,#19595,.T.);
#27634=ORIENTED_EDGE('',*,*,#19668,.T.);
#27635=ORIENTED_EDGE('',*,*,#19621,.T.);
#30294=CONICAL_SURFACE('',#33442,0.916025403784424,0.785398163397437);
#30295=CONICAL_SURFACE('',#33483,0.433012701892235,1.02974425867666);
#30296=CONICAL_SURFACE('',#33489,1.25,0.785398163397456);
#30297=CONICAL_SURFACE('',#33490,1.35,0.785398163397469);
#31571=ADVANCED_FACE('',(#4596),#1856,.T.);
#31572=ADVANCED_FACE('',(#4597),#1857,.T.);
#31573=ADVANCED_FACE('',(#4598),#1858,.T.);
#31574=ADVANCED_FACE('',(#4599),#1859,.T.);
#31575=ADVANCED_FACE('',(#4600),#1860,.T.);
#31576=ADVANCED_FACE('',(#4601),#1861,.T.);
#31577=ADVANCED_FACE('',(#4602),#1862,.T.);
#31578=ADVANCED_FACE('',(#4603),#1863,.T.);
#31579=ADVANCED_FACE('',(#4604),#1864,.T.);
#31580=ADVANCED_FACE('',(#4605),#1865,.T.);
#31581=ADVANCED_FACE('',(#4606),#1866,.T.);
#31582=ADVANCED_FACE('',(#4607),#1867,.T.);
#31583=ADVANCED_FACE('',(#4608),#1868,.T.);
#31584=ADVANCED_FACE('',(#4609),#1869,.T.);
#31585=ADVANCED_FACE('',(#4610),#1870,.T.);
#31586=ADVANCED_FACE('',(#4611),#1871,.T.);
#31587=ADVANCED_FACE('',(#4612),#1872,.T.);
#31588=ADVANCED_FACE('',(#4613),#1873,.T.);
#31589=ADVANCED_FACE('',(#4614),#1874,.T.);
#31590=ADVANCED_FACE('',(#4615),#3042,.F.);
#31591=ADVANCED_FACE('',(#4616),#609,.F.);
#31592=ADVANCED_FACE('',(#4617),#3043,.T.);
#31593=ADVANCED_FACE('',(#4618),#610,.F.);
#31594=ADVANCED_FACE('',(#4619),#30294,.F.);
#31595=ADVANCED_FACE('',(#4620),#1875,.T.);
#31596=ADVANCED_FACE('',(#4621),#1876,.T.);
#31597=ADVANCED_FACE('',(#4622),#1877,.T.);
#31598=ADVANCED_FACE('',(#4623),#1878,.T.);
#31599=ADVANCED_FACE('',(#4624),#1879,.T.);
#31600=ADVANCED_FACE('',(#4625),#1880,.T.);
#31601=ADVANCED_FACE('',(#4626),#3044,.F.);
#31602=ADVANCED_FACE('',(#4627),#3045,.F.);
#31603=ADVANCED_FACE('',(#4628),#3046,.F.);
#31604=ADVANCED_FACE('',(#4629),#3047,.T.);
#31605=ADVANCED_FACE('',(#4630),#3048,.T.);
#31606=ADVANCED_FACE('',(#4631),#3049,.T.);
#31607=ADVANCED_FACE('',(#4632),#3050,.T.);
#31608=ADVANCED_FACE('',(#4633),#3051,.T.);
#31609=ADVANCED_FACE('',(#4634),#3052,.T.);
#31610=ADVANCED_FACE('',(#4635),#3053,.F.);
#31611=ADVANCED_FACE('',(#4636),#3054,.F.);
#31612=ADVANCED_FACE('',(#4637),#3055,.F.);
#31613=ADVANCED_FACE('',(#4638),#3056,.F.);
#31614=ADVANCED_FACE('',(#4639),#3057,.F.);
#31615=ADVANCED_FACE('',(#4640),#3058,.F.);
#31616=ADVANCED_FACE('',(#4641),#30295,.F.);
#31617=ADVANCED_FACE('',(#4642),#3059,.F.);
#31618=ADVANCED_FACE('',(#4643),#3060,.F.);
#31619=ADVANCED_FACE('',(#4644),#3061,.F.);
#31620=ADVANCED_FACE('',(#4645),#3062,.T.);
#31621=ADVANCED_FACE('',(#4646),#30296,.T.);
#31622=ADVANCED_FACE('',(#4647),#30297,.T.);
#31623=ADVANCED_FACE('',(#4648,#2214),#3063,.T.);
#32083=CLOSED_SHELL('',(#31571,#31572,#31573,#31574,#31575,#31576,#31577,
#31578,#31579,#31580,#31581,#31582,#31583,#31584,#31585,#31586,#31587,#31588,
#31589,#31590,#31591,#31592,#31593,#31594,#31595,#31596,#31597,#31598,#31599,
#31600,#31601,#31602,#31603,#31604,#31605,#31606,#31607,#31608,#31609,#31610,
#31611,#31612,#31613,#31614,#31615,#31616,#31617,#31618,#31619,#31620,#31621,
#31622,#31623));
#33412=AXIS2_PLACEMENT_3D('',#77153,#38780,#38781);
#33413=AXIS2_PLACEMENT_3D('',#77154,#38782,#38783);
#33414=AXIS2_PLACEMENT_3D('',#77218,#38785,#38786);
#33415=AXIS2_PLACEMENT_3D('',#77250,#38787,#38788);
#33416=AXIS2_PLACEMENT_3D('',#77640,#38790,#38791);
#33417=AXIS2_PLACEMENT_3D('',#78039,#38793,#38794);
#33418=AXIS2_PLACEMENT_3D('',#78419,#38796,#38797);
#33419=AXIS2_PLACEMENT_3D('',#78774,#38799,#38800);
#33420=AXIS2_PLACEMENT_3D('',#79140,#38802,#38803);
#33421=AXIS2_PLACEMENT_3D('',#79499,#38805,#38806);
#33422=AXIS2_PLACEMENT_3D('',#79883,#38808,#38809);
#33423=AXIS2_PLACEMENT_3D('',#80253,#38811,#38812);
#33424=AXIS2_PLACEMENT_3D('',#80389,#38814,#38815);
#33425=AXIS2_PLACEMENT_3D('',#80486,#38816,#38817);
#33426=AXIS2_PLACEMENT_3D('',#80832,#38819,#38820);
#33427=AXIS2_PLACEMENT_3D('',#81166,#38822,#38823);
#33428=AXIS2_PLACEMENT_3D('',#81503,#38825,#38826);
#33429=AXIS2_PLACEMENT_3D('',#81841,#38828,#38829);
#33430=AXIS2_PLACEMENT_3D('',#82191,#38831,#38832);
#33431=AXIS2_PLACEMENT_3D('',#82540,#38834,#38835);
#33432=AXIS2_PLACEMENT_3D('',#82868,#38837,#38838);
#33433=AXIS2_PLACEMENT_3D('',#83027,#38839,#38840);
#33434=AXIS2_PLACEMENT_3D('',#83150,#38841,#38842);
#33435=AXIS2_PLACEMENT_3D('',#83215,#38843,#38844);
#33436=AXIS2_PLACEMENT_3D('',#83256,#38845,#38846);
#33437=AXIS2_PLACEMENT_3D('',#83259,#38847,#38848);
#33438=AXIS2_PLACEMENT_3D('',#83356,#38849,#38850);
#33439=AXIS2_PLACEMENT_3D('',#83689,#38851,#38852);
#33440=AXIS2_PLACEMENT_3D('',#83691,#38853,#38854);
#33441=AXIS2_PLACEMENT_3D('',#83693,#38855,#38856);
#33442=AXIS2_PLACEMENT_3D('',#84018,#38857,#38858);
#33443=AXIS2_PLACEMENT_3D('',#84025,#38859,#38860);
#33444=AXIS2_PLACEMENT_3D('',#84035,#38861,#38862);
#33445=AXIS2_PLACEMENT_3D('',#84045,#38863,#38864);
#33446=AXIS2_PLACEMENT_3D('',#84055,#38865,#38866);
#33447=AXIS2_PLACEMENT_3D('',#84065,#38867,#38868);
#33448=AXIS2_PLACEMENT_3D('',#84075,#38869,#38870);
#33449=AXIS2_PLACEMENT_3D('',#84081,#38872,#38873);
#33450=AXIS2_PLACEMENT_3D('',#84082,#38874,#38875);
#33451=AXIS2_PLACEMENT_3D('',#84087,#38878,#38879);
#33452=AXIS2_PLACEMENT_3D('',#84088,#38880,#38881);
#33453=AXIS2_PLACEMENT_3D('',#84092,#38883,#38884);
#33454=AXIS2_PLACEMENT_3D('',#84094,#38886,#38887);
#33455=AXIS2_PLACEMENT_3D('',#84099,#38890,#38891);
#33456=AXIS2_PLACEMENT_3D('',#84100,#38892,#38893);
#33457=AXIS2_PLACEMENT_3D('',#84104,#38895,#38896);
#33458=AXIS2_PLACEMENT_3D('',#84106,#38898,#38899);
#33459=AXIS2_PLACEMENT_3D('',#84111,#38902,#38903);
#33460=AXIS2_PLACEMENT_3D('',#84112,#38904,#38905);
#33461=AXIS2_PLACEMENT_3D('',#84116,#38907,#38908);
#33462=AXIS2_PLACEMENT_3D('',#84118,#38910,#38911);
#33463=AXIS2_PLACEMENT_3D('',#84125,#38916,#38917);
#33464=AXIS2_PLACEMENT_3D('',#84130,#38921,#38922);
#33465=AXIS2_PLACEMENT_3D('',#84135,#38926,#38927);
#33466=AXIS2_PLACEMENT_3D('',#84136,#38928,#38929);
#33467=AXIS2_PLACEMENT_3D('',#84137,#38930,#38931);
#33468=AXIS2_PLACEMENT_3D('',#84139,#38933,#38934);
#33469=AXIS2_PLACEMENT_3D('',#84140,#38935,#38936);
#33470=AXIS2_PLACEMENT_3D('',#84142,#38938,#38939);
#33471=AXIS2_PLACEMENT_3D('',#84144,#38941,#38942);
#33472=AXIS2_PLACEMENT_3D('',#84148,#38944,#38945);
#33473=AXIS2_PLACEMENT_3D('',#84149,#38946,#38947);
#33474=AXIS2_PLACEMENT_3D('',#84151,#38949,#38950);
#33475=AXIS2_PLACEMENT_3D('',#84152,#38951,#38952);
#33476=AXIS2_PLACEMENT_3D('',#84153,#38953,#38954);
#33477=AXIS2_PLACEMENT_3D('',#84154,#38955,#38956);
#33478=AXIS2_PLACEMENT_3D('',#84155,#38957,#38958);
#33479=AXIS2_PLACEMENT_3D('',#84156,#38959,#38960);
#33480=AXIS2_PLACEMENT_3D('',#84157,#38961,#38962);
#33481=AXIS2_PLACEMENT_3D('',#84158,#38963,#38964);
#33482=AXIS2_PLACEMENT_3D('',#84160,#38966,#38967);
#33483=AXIS2_PLACEMENT_3D('',#84161,#38968,#38969);
#33484=AXIS2_PLACEMENT_3D('',#84164,#38971,#38972);
#33485=AXIS2_PLACEMENT_3D('',#84167,#38975,#38976);
#33486=AXIS2_PLACEMENT_3D('',#84168,#38977,#38978);
#33487=AXIS2_PLACEMENT_3D('',#84169,#38979,#38980);
#33488=AXIS2_PLACEMENT_3D('',#84171,#38981,#38982);
#33489=AXIS2_PLACEMENT_3D('',#84172,#38983,#38984);
#33490=AXIS2_PLACEMENT_3D('',#84174,#38986,#38987);
#33491=AXIS2_PLACEMENT_3D('',#84177,#38989,#38990);
#33492=AXIS2_PLACEMENT_3D('',#84178,#38991,#38992);
#38780=DIRECTION('axis',(0.,0.,1.));
#38781=DIRECTION('refdir',(1.,0.,0.));
#38782=DIRECTION('center_axis',(1.,0.,0.));
#38783=DIRECTION('ref_axis',(0.,1.,0.));
#38784=DIRECTION('',(-1.,0.,0.));
#38785=DIRECTION('center_axis',(1.,0.,0.));
#38786=DIRECTION('ref_axis',(0.,1.,0.));
#38787=DIRECTION('center_axis',(1.,0.,0.));
#38788=DIRECTION('ref_axis',(0.,1.,0.));
#38789=DIRECTION('',(-1.,0.,0.));
#38790=DIRECTION('center_axis',(1.,0.,0.));
#38791=DIRECTION('ref_axis',(0.,1.,0.));
#38792=DIRECTION('',(-1.,0.,0.));
#38793=DIRECTION('center_axis',(1.,0.,0.));
#38794=DIRECTION('ref_axis',(0.,1.,0.));
#38795=DIRECTION('',(-1.,0.,0.));
#38796=DIRECTION('center_axis',(1.,0.,0.));
#38797=DIRECTION('ref_axis',(0.,1.,0.));
#38798=DIRECTION('',(-1.,0.,0.));
#38799=DIRECTION('center_axis',(1.,0.,0.));
#38800=DIRECTION('ref_axis',(0.,1.,0.));
#38801=DIRECTION('',(-1.,0.,0.));
#38802=DIRECTION('center_axis',(1.,0.,0.));
#38803=DIRECTION('ref_axis',(0.,1.,0.));
#38804=DIRECTION('',(-1.,0.,0.));
#38805=DIRECTION('center_axis',(1.,0.,0.));
#38806=DIRECTION('ref_axis',(0.,1.,0.));
#38807=DIRECTION('',(-1.,0.,0.));
#38808=DIRECTION('center_axis',(1.,0.,0.));
#38809=DIRECTION('ref_axis',(0.,1.,0.));
#38810=DIRECTION('',(-1.,0.,0.));
#38811=DIRECTION('center_axis',(1.,0.,0.));
#38812=DIRECTION('ref_axis',(0.,0.945745520993383,-0.32490830940583));
#38813=DIRECTION('',(-1.,0.,0.));
#38814=DIRECTION('center_axis',(-1.,0.,0.));
#38815=DIRECTION('ref_axis',(0.,1.,3.95919057815806E-14));
#38816=DIRECTION('center_axis',(1.,0.,0.));
#38817=DIRECTION('ref_axis',(0.,0.945745520993383,-0.32490830940583));
#38818=DIRECTION('',(-1.,0.,0.));
#38819=DIRECTION('center_axis',(1.,0.,0.));
#38820=DIRECTION('ref_axis',(0.,0.945745520993383,-0.32490830940583));
#38821=DIRECTION('',(-1.,0.,0.));
#38822=DIRECTION('center_axis',(1.,0.,0.));
#38823=DIRECTION('ref_axis',(0.,0.945745520993383,-0.32490830940583));
#38824=DIRECTION('',(-1.,0.,0.));
#38825=DIRECTION('center_axis',(1.,0.,0.));
#38826=DIRECTION('ref_axis',(0.,0.945745520993383,-0.32490830940583));
#38827=DIRECTION('',(-1.,0.,0.));
#38828=DIRECTION('center_axis',(1.,0.,0.));
#38829=DIRECTION('ref_axis',(0.,0.945745520993383,-0.32490830940583));
#38830=DIRECTION('',(-1.,0.,0.));
#38831=DIRECTION('center_axis',(1.,0.,0.));
#38832=DIRECTION('ref_axis',(0.,0.945745520993383,-0.32490830940583));
#38833=DIRECTION('',(-1.,0.,0.));
#38834=DIRECTION('center_axis',(1.,0.,0.));
#38835=DIRECTION('ref_axis',(0.,0.945745520993383,-0.32490830940583));
#38836=DIRECTION('',(-1.,0.,0.));
#38837=DIRECTION('center_axis',(1.,0.,0.));
#38838=DIRECTION('ref_axis',(0.,0.945745520993383,-0.32490830940583));
#38839=DIRECTION('center_axis',(1.,0.,0.));
#38840=DIRECTION('ref_axis',(0.,1.,3.95919057815806E-14));
#38841=DIRECTION('center_axis',(1.,0.,0.));
#38842=DIRECTION('ref_axis',(0.,-0.404759137094124,-0.914423337923317));
#38843=DIRECTION('center_axis',(-1.,0.,0.));
#38844=DIRECTION('ref_axis',(0.,1.,0.));
#38845=DIRECTION('center_axis',(1.,0.,0.));
#38846=DIRECTION('ref_axis',(0.,0.,-1.));
#38847=DIRECTION('center_axis',(-1.,0.,0.));
#38848=DIRECTION('ref_axis',(0.,1.,0.));
#38849=DIRECTION('center_axis',(-1.,0.,0.));
#38850=DIRECTION('ref_axis',(0.,1.,0.));
#38851=DIRECTION('center_axis',(1.,0.,0.));
#38852=DIRECTION('ref_axis',(0.,0.,-1.));
#38853=DIRECTION('center_axis',(1.,0.,0.));
#38854=DIRECTION('ref_axis',(0.,1.,0.));
#38855=DIRECTION('center_axis',(1.,0.,0.));
#38856=DIRECTION('ref_axis',(0.,1.,0.));
#38857=DIRECTION('center_axis',(1.,0.,0.));
#38858=DIRECTION('ref_axis',(0.,1.,0.));
#38859=DIRECTION('center_axis',(1.,0.,0.));
#38860=DIRECTION('ref_axis',(0.,0.,-1.));
#38861=DIRECTION('center_axis',(1.,0.,0.));
#38862=DIRECTION('ref_axis',(0.,0.,-1.));
#38863=DIRECTION('center_axis',(1.,0.,0.));
#38864=DIRECTION('ref_axis',(0.,0.,-1.));
#38865=DIRECTION('center_axis',(1.,0.,0.));
#38866=DIRECTION('ref_axis',(0.,0.,-1.));
#38867=DIRECTION('center_axis',(1.,0.,0.));
#38868=DIRECTION('ref_axis',(0.,0.,-1.));
#38869=DIRECTION('center_axis',(1.,0.,0.));
#38870=DIRECTION('ref_axis',(0.,0.,-1.));
#38871=DIRECTION('',(0.707106781186556,-0.707106781186539,-8.65956056235483E-17));
#38872=DIRECTION('center_axis',(-1.,0.,0.));
#38873=DIRECTION('ref_axis',(0.,1.,0.));
#38874=DIRECTION('center_axis',(1.,0.,0.));
#38875=DIRECTION('ref_axis',(0.,1.,0.));
#38876=DIRECTION('',(1.,0.,0.));
#38877=DIRECTION('',(-1.,0.,0.));
#38878=DIRECTION('center_axis',(1.,0.,0.));
#38879=DIRECTION('ref_axis',(0.,1.,0.));
#38880=DIRECTION('center_axis',(1.,0.,0.));
#38881=DIRECTION('ref_axis',(0.,1.,0.));
#38882=DIRECTION('',(-1.,0.,0.));
#38883=DIRECTION('center_axis',(1.,0.,0.));
#38884=DIRECTION('ref_axis',(0.,1.,0.));
#38885=DIRECTION('',(1.,0.,0.));
#38886=DIRECTION('center_axis',(1.,0.,0.));
#38887=DIRECTION('ref_axis',(0.,1.,0.));
#38888=DIRECTION('',(1.,0.,0.));
#38889=DIRECTION('',(-1.,0.,0.));
#38890=DIRECTION('center_axis',(1.,0.,0.));
#38891=DIRECTION('ref_axis',(0.,1.,0.));
#38892=DIRECTION('center_axis',(1.,0.,0.));
#38893=DIRECTION('ref_axis',(0.,1.,0.));
#38894=DIRECTION('',(-1.,0.,0.));
#38895=DIRECTION('center_axis',(1.,0.,0.));
#38896=DIRECTION('ref_axis',(0.,1.,0.));
#38897=DIRECTION('',(1.,0.,0.));
#38898=DIRECTION('center_axis',(1.,0.,0.));
#38899=DIRECTION('ref_axis',(0.,1.,0.));
#38900=DIRECTION('',(1.,0.,0.));
#38901=DIRECTION('',(-1.,0.,0.));
#38902=DIRECTION('center_axis',(1.,0.,0.));
#38903=DIRECTION('ref_axis',(0.,1.,0.));
#38904=DIRECTION('center_axis',(1.,0.,0.));
#38905=DIRECTION('ref_axis',(0.,1.,0.));
#38906=DIRECTION('',(-1.,0.,0.));
#38907=DIRECTION('center_axis',(1.,0.,0.));
#38908=DIRECTION('ref_axis',(0.,1.,0.));
#38909=DIRECTION('',(1.,0.,0.));
#38910=DIRECTION('center_axis',(0.,-0.866025403784431,0.500000000000014));
#38911=DIRECTION('ref_axis',(0.,0.500000000000014,0.866025403784431));
#38912=DIRECTION('',(0.,0.500000000000014,0.866025403784431));
#38913=DIRECTION('',(-1.,0.,0.));
#38914=DIRECTION('',(0.,0.500000000000014,0.866025403784431));
#38915=DIRECTION('',(-1.,0.,0.));
#38916=DIRECTION('center_axis',(0.,-0.866025403784431,-0.500000000000014));
#38917=DIRECTION('ref_axis',(0.,-0.500000000000014,0.866025403784431));
#38918=DIRECTION('',(0.,-0.500000000000014,0.866025403784431));
#38919=DIRECTION('',(-1.,0.,0.));
#38920=DIRECTION('',(0.,-0.500000000000014,0.866025403784431));
#38921=DIRECTION('center_axis',(0.,0.,-1.));
#38922=DIRECTION('ref_axis',(0.,-1.,0.));
#38923=DIRECTION('',(0.,-1.,0.));
#38924=DIRECTION('',(-1.,0.,0.));
#38925=DIRECTION('',(0.,-1.,0.));
#38926=DIRECTION('center_axis',(1.,0.,0.));
#38927=DIRECTION('ref_axis',(0.,0.,-1.));
#38928=DIRECTION('center_axis',(1.,0.,0.));
#38929=DIRECTION('ref_axis',(0.,0.,-1.));
#38930=DIRECTION('center_axis',(1.,0.,0.));
#38931=DIRECTION('ref_axis',(0.,0.,-1.));
#38932=DIRECTION('',(0.,-0.500000000000029,-0.866025403784422));
#38933=DIRECTION('center_axis',(1.,0.,0.));
#38934=DIRECTION('ref_axis',(0.,0.,-1.));
#38935=DIRECTION('center_axis',(1.,0.,0.));
#38936=DIRECTION('ref_axis',(0.,0.,-1.));
#38937=DIRECTION('',(0.,0.500000000000029,-0.866025403784422));
#38938=DIRECTION('center_axis',(1.,0.,0.));
#38939=DIRECTION('ref_axis',(0.,0.,-1.));
#38940=DIRECTION('',(0.,1.,0.));
#38941=DIRECTION('center_axis',(1.,0.,0.));
#38942=DIRECTION('ref_axis',(0.,0.,-1.));
#38943=DIRECTION('',(0.,0.500000000000029,-0.866025403784422));
#38944=DIRECTION('center_axis',(1.,0.,0.));
#38945=DIRECTION('ref_axis',(0.,0.,-1.));
#38946=DIRECTION('center_axis',(1.,0.,0.));
#38947=DIRECTION('ref_axis',(0.,0.,-1.));
#38948=DIRECTION('',(0.,-0.500000000000029,-0.866025403784422));
#38949=DIRECTION('center_axis',(1.,0.,0.));
#38950=DIRECTION('ref_axis',(0.,0.,-1.));
#38951=DIRECTION('center_axis',(1.,0.,0.));
#38952=DIRECTION('ref_axis',(0.,0.,-1.));
#38953=DIRECTION('center_axis',(1.,0.,0.));
#38954=DIRECTION('ref_axis',(0.,0.,-1.));
#38955=DIRECTION('center_axis',(1.,0.,0.));
#38956=DIRECTION('ref_axis',(0.,0.,-1.));
#38957=DIRECTION('center_axis',(1.,0.,0.));
#38958=DIRECTION('ref_axis',(0.,0.,-1.));
#38959=DIRECTION('center_axis',(1.,0.,0.));
#38960=DIRECTION('ref_axis',(0.,0.,-1.));
#38961=DIRECTION('center_axis',(1.,0.,0.));
#38962=DIRECTION('ref_axis',(0.,0.,-1.));
#38963=DIRECTION('center_axis',(1.,0.,0.));
#38964=DIRECTION('ref_axis',(0.,0.,-1.));
#38965=DIRECTION('',(0.,1.,0.));
#38966=DIRECTION('center_axis',(1.,0.,0.));
#38967=DIRECTION('ref_axis',(0.,0.,-1.));
#38968=DIRECTION('center_axis',(1.,0.,0.));
#38969=DIRECTION('ref_axis',(0.,1.,0.));
#38970=DIRECTION('',(0.515038074910049,-0.857167300702115,-1.04972719113862E-16));
#38971=DIRECTION('center_axis',(0.,0.866025403784422,0.500000000000029));
#38972=DIRECTION('ref_axis',(0.,0.500000000000029,-0.866025403784422));
#38973=DIRECTION('',(-1.,0.,0.));
#38974=DIRECTION('',(-1.,0.,0.));
#38975=DIRECTION('center_axis',(0.,0.,1.));
#38976=DIRECTION('ref_axis',(0.,1.,0.));
#38977=DIRECTION('center_axis',(0.,0.866025403784422,-0.500000000000029));
#38978=DIRECTION('ref_axis',(0.,-0.500000000000029,-0.866025403784422));
#38979=DIRECTION('center_axis',(-1.,0.,0.));
#38980=DIRECTION('ref_axis',(0.,0.,1.));
#38981=DIRECTION('center_axis',(1.,0.,0.));
#38982=DIRECTION('ref_axis',(0.,0.,-1.));
#38983=DIRECTION('center_axis',(1.,0.,0.));
#38984=DIRECTION('ref_axis',(0.,1.,0.));
#38985=DIRECTION('',(-0.707106781186542,0.707106781186553,8.659560562355E-17));
#38986=DIRECTION('center_axis',(-1.,0.,0.));
#38987=DIRECTION('ref_axis',(0.,1.,0.));
#38988=DIRECTION('',(0.707106781186533,0.707106781186562,-8.65956056235511E-17));
#38989=DIRECTION('center_axis',(1.,0.,0.));
#38990=DIRECTION('ref_axis',(0.,0.,-1.));
#38991=DIRECTION('center_axis',(1.,0.,0.));
#38992=DIRECTION('ref_axis',(0.,0.,-1.));
#77153=CARTESIAN_POINT('',(0.,0.,0.));
#77154=CARTESIAN_POINT('Origin',(4.2,139.,13.3));
#77155=CARTESIAN_POINT('',(2.2251969548064,137.5365,13.2999999724982));
#77156=CARTESIAN_POINT('',(2.15284495415709,137.536500503216,13.3012136364406));
#77157=CARTESIAN_POINT('',(4.2,137.5365,13.3));
#77158=CARTESIAN_POINT('',(2.0641830960939,139.63445579128,14.6190127185149));
#77159=CARTESIAN_POINT('Ctrl Pts',(2.06484487113285,139.634380960677,14.6188605107176));
#77160=CARTESIAN_POINT('Ctrl Pts',(2.07154330550746,139.516436019972,14.6755928369821));
#77161=CARTESIAN_POINT('Ctrl Pts',(2.07762498273557,139.391404855929,14.7162526547379));
#77162=CARTESIAN_POINT('Ctrl Pts',(2.08649714863426,139.216238221626,14.7482044865399));
#77163=CARTESIAN_POINT('Ctrl Pts',(2.08889178538834,139.169476945985,14.7544181785645));
#77164=CARTESIAN_POINT('Ctrl Pts',(2.09231151530127,139.104262707784,14.7598960496728));
#77165=CARTESIAN_POINT('Ctrl Pts',(2.0932777214869,139.085999063756,14.7610856612976));
#77166=CARTESIAN_POINT('Ctrl Pts',(2.09497000815552,139.054327780598,14.7625527123752));
#77167=CARTESIAN_POINT('Ctrl Pts',(2.09569109521671,139.040929560602,14.7629889606482));
#77168=CARTESIAN_POINT('Ctrl Pts',(2.09719470100381,139.013204014515,14.7635105533602));
#77169=CARTESIAN_POINT('Ctrl Pts',(2.09797795278032,138.998877684261,14.7635696792124));
#77170=CARTESIAN_POINT('Ctrl Pts',(2.10004847387981,138.961322163813,14.7631732683632));
#77171=CARTESIAN_POINT('Ctrl Pts',(2.10134607908924,138.938101320443,14.7623749368849));
#77172=CARTESIAN_POINT('Ctrl Pts',(2.10859075663927,138.810212841032,14.7549267336709));
#77173=CARTESIAN_POINT('Ctrl Pts',(2.11486128108125,138.706487368182,14.7375936245252));
#77174=CARTESIAN_POINT('Ctrl Pts',(2.12411026253069,138.558087782332,14.6960558892612));
#77175=CARTESIAN_POINT('Ctrl Pts',(2.12705998570955,138.511352950434,14.6803922987276));
#77176=CARTESIAN_POINT('Ctrl Pts',(2.13161267157336,138.438928683095,14.6519784229804));
#77177=CARTESIAN_POINT('Ctrl Pts',(2.13325897783698,138.412670772443,14.6407800921261));
#77178=CARTESIAN_POINT('Ctrl Pts',(2.13547313520369,138.377006577717,14.6243212348215));
#77179=CARTESIAN_POINT('Ctrl Pts',(2.13607302496145,138.367306999997,14.6197147868878));
#77180=CARTESIAN_POINT('Ctrl Pts',(2.13708688600052,138.35083225505,14.6116673391423));
#77181=CARTESIAN_POINT('Ctrl Pts',(2.13750388562067,138.34403167401,14.6082796086849));
#77182=CARTESIAN_POINT('Ctrl Pts',(2.13839379691369,138.329459608557,14.6008782900398));
#77183=CARTESIAN_POINT('Ctrl Pts',(2.13886569620043,138.32169726621,14.5968477748556));
#77184=CARTESIAN_POINT('Ctrl Pts',(2.14022664500463,138.299229529139,14.5849247132341));
#77185=CARTESIAN_POINT('Ctrl Pts',(2.141105259426,138.284622015765,14.576849700171));
#77186=CARTESIAN_POINT('Ctrl Pts',(2.14568093691103,138.208274242917,14.5329231190416));
#77187=CARTESIAN_POINT('Ctrl Pts',(2.14917413717831,138.149075567429,14.4928363322984));
#77188=CARTESIAN_POINT('Ctrl Pts',(2.15615714477518,138.036536945863,14.4039717549171));
#77189=CARTESIAN_POINT('Ctrl Pts',(2.15963902309474,137.983408114186,14.355251232627));
#77190=CARTESIAN_POINT('Ctrl Pts',(2.16542259001683,137.904256023087,14.2711189460665));
#77191=CARTESIAN_POINT('Ctrl Pts',(2.16764235849417,137.875861400932,14.2381038600084));
#77192=CARTESIAN_POINT('Ctrl Pts',(2.17085156010389,137.837997571907,14.189887014097));
#77193=CARTESIAN_POINT('Ctrl Pts',(2.17179187459467,137.827269832423,14.1757011239281));
#77194=CARTESIAN_POINT('Ctrl Pts',(2.17345236454698,137.808982294968,14.1505796158621));
#77195=CARTESIAN_POINT('Ctrl Pts',(2.17416803256024,137.801307917839,14.1397297975067));
#77196=CARTESIAN_POINT('Ctrl Pts',(2.17567344767817,137.78560227226,14.1168715144026));
#77197=CARTESIAN_POINT('Ctrl Pts',(2.17646413874395,137.77759894815,14.1048456744472));
#77198=CARTESIAN_POINT('Ctrl Pts',(2.1785851962511,137.756786226949,14.0725456746905));
#77199=CARTESIAN_POINT('Ctrl Pts',(2.17992696594011,137.744295305875,14.0520724240382));
#77200=CARTESIAN_POINT('Ctrl Pts',(2.18788516733776,137.674136401513,13.9304544687656));
#77201=CARTESIAN_POINT('Ctrl Pts',(2.19491253895104,137.628208659697,13.8230369797022));
#77202=CARTESIAN_POINT('Ctrl Pts',(2.20453657899678,137.583225008379,13.6694411294335));
#77203=CARTESIAN_POINT('Ctrl Pts',(2.20714717172512,137.572834993177,13.6270145557349));
#77204=CARTESIAN_POINT('Ctrl Pts',(2.21124977622621,137.559208651109,13.5581771932772));
#77205=CARTESIAN_POINT('Ctrl Pts',(2.21277752855814,137.554767735982,13.5320324223786));
#77206=CARTESIAN_POINT('Ctrl Pts',(2.21485710674279,137.549579562116,13.4955008800206));
#77207=CARTESIAN_POINT('Ctrl Pts',(2.21543707823911,137.548229115306,13.4852062414051));
#77208=CARTESIAN_POINT('Ctrl Pts',(2.21642385112219,137.546096418386,13.4674882740937));
#77209=CARTESIAN_POINT('Ctrl Pts',(2.21683344472635,137.545261207564,13.4600718632937));
#77210=CARTESIAN_POINT('Ctrl Pts',(2.21771407477505,137.543574175518,13.4439859076296));
#77211=CARTESIAN_POINT('Ctrl Pts',(2.21818400497777,137.542742965998,13.4353147014655));
#77212=CARTESIAN_POINT('Ctrl Pts',(2.21952396927374,137.540575546037,13.4103604037126));
#77213=CARTESIAN_POINT('Ctrl Pts',(2.22038400700859,137.539434464801,13.3940612374598));
#77214=CARTESIAN_POINT('Ctrl Pts',(2.22258002585803,137.537188697747,13.3518461985471));
#77215=CARTESIAN_POINT('Ctrl Pts',(2.22389800731999,137.536499999513,13.3259217714187));
#77216=CARTESIAN_POINT('Ctrl Pts',(2.22519695480639,137.5365,13.2999999724982));
#77217=CARTESIAN_POINT('',(2.0635,138.365992905425,14.6190402776368));
#77218=CARTESIAN_POINT('Origin',(2.0635,139.,13.3));
#77219=CARTESIAN_POINT('Ctrl Pts',(2.0635,138.365992905425,14.6190402776369));
#77220=CARTESIAN_POINT('Ctrl Pts',(2.0665728961224,138.315057965225,14.5945579976066));
#77221=CARTESIAN_POINT('Ctrl Pts',(2.0696457922448,138.265498495672,14.5671001288649));
#77222=CARTESIAN_POINT('Ctrl Pts',(2.0727186883672,138.217668754599,14.5368468265996));
#77223=CARTESIAN_POINT('Ctrl Pts',(2.07578984658353,138.169866064098,14.5066106343814));
#77224=CARTESIAN_POINT('Ctrl Pts',(2.07886100479987,138.123791580139,14.4735824089652));
#77225=CARTESIAN_POINT('Ctrl Pts',(2.08193216301621,138.079773340259,14.4379873218545));
#77226=CARTESIAN_POINT('Ctrl Pts',(2.08500244800625,138.035767616141,14.4024023555399));
#77227=CARTESIAN_POINT('Ctrl Pts',(2.08807273299629,137.993817360905,14.3642522881152));
#77228=CARTESIAN_POINT('Ctrl Pts',(2.09114301798633,137.95421850133,14.3238033536967));
#77229=CARTESIAN_POINT('Ctrl Pts',(2.09421341287704,137.914618224317,14.2833529714109));
#77230=CARTESIAN_POINT('Ctrl Pts',(2.09728380776776,137.877369856597,14.2406039136272));
#77231=CARTESIAN_POINT('Ctrl Pts',(2.10035420265847,137.842731963572,14.1958587733915));
#77232=CARTESIAN_POINT('Ctrl Pts',(2.10342569040786,137.808081741735,14.1510977068281));
#77233=CARTESIAN_POINT('Ctrl Pts',(2.10649717815726,137.776044142247,14.1043395398346));
#77234=CARTESIAN_POINT('Ctrl Pts',(2.10956866590665,137.74683581807,14.0559178415192));
#77235=CARTESIAN_POINT('Ctrl Pts',(2.1126447961947,137.717583345654,14.0074229540446));
#77236=CARTESIAN_POINT('Ctrl Pts',(2.11572092648275,137.691168941285,13.9572599420295));
#77237=CARTESIAN_POINT('Ctrl Pts',(2.1187970567708,137.66776399032,13.9057883000785));
#77238=CARTESIAN_POINT('Ctrl Pts',(2.12187565596135,137.644340254539,13.854275346982));
#77239=CARTESIAN_POINT('Ctrl Pts',(2.12495425515191,137.623930962426,13.8014521348082));
#77240=CARTESIAN_POINT('Ctrl Pts',(2.12803285434246,137.606658688541,13.7476965934434));
#77241=CARTESIAN_POINT('Ctrl Pts',(2.13111793264504,137.589350064032,13.6938279200492));
#77242=CARTESIAN_POINT('Ctrl Pts',(2.13420301094762,137.575191770299,13.6390234789101));
#77243=CARTESIAN_POINT('Ctrl Pts',(2.13728808925019,137.5642558315,13.5836739900301));
#77244=CARTESIAN_POINT('Ctrl Pts',(2.13910859425859,137.557802532945,13.551012251223));
#77245=CARTESIAN_POINT('Ctrl Pts',(2.14092909926698,137.552470335605,13.5181608773554));
#77246=CARTESIAN_POINT('Ctrl Pts',(2.14274960427537,137.548265548371,13.4852007882095));
#77247=CARTESIAN_POINT('Ctrl Pts',(2.14611472090261,137.540493199836,13.4242756363922));
#77248=CARTESIAN_POINT('Ctrl Pts',(2.14947983752985,137.536551593288,13.3628221147701));
#77249=CARTESIAN_POINT('Ctrl Pts',(2.15284495415709,137.536500503216,13.3012136364406));
#77250=CARTESIAN_POINT('Origin',(4.2,139.,13.3));
#77251=CARTESIAN_POINT('',(2.72330048309449,137.536992130936,13.300479477908));
#77252=CARTESIAN_POINT('',(2.65378340881734,137.537042726446,13.3005506582616));
#77253=CARTESIAN_POINT('',(4.2,137.5365,13.3));
#77254=CARTESIAN_POINT('Ctrl Pts',(2.22519695480639,137.5365,13.2999999724982));
#77255=CARTESIAN_POINT('Ctrl Pts',(2.22748597883763,137.536500000858,13.2543202038524));
#77256=CARTESIAN_POINT('Ctrl Pts',(2.22971638608312,137.538638685949,13.2086486214609));
#77257=CARTESIAN_POINT('Ctrl Pts',(2.23545370680436,137.549673160254,13.0911733936797));
#77258=CARTESIAN_POINT('Ctrl Pts',(2.23894358657392,137.56175428192,13.0198120653719));
#77259=CARTESIAN_POINT('Ctrl Pts',(2.24473778427457,137.589490539063,12.907323702418));
#77260=CARTESIAN_POINT('Ctrl Pts',(2.24695836509237,137.601808176735,12.865499360933));
#77261=CARTESIAN_POINT('Ctrl Pts',(2.25016330812179,137.621720741502,12.8075660116011));
#77262=CARTESIAN_POINT('Ctrl Pts',(2.25109779072504,137.627771127863,12.7909490853336));
#77263=CARTESIAN_POINT('Ctrl Pts',(2.25274516472884,137.638846575935,12.7621647322052));
#77264=CARTESIAN_POINT('Ctrl Pts',(2.25345351216668,137.643737526163,12.7499477247201));
#77265=CARTESIAN_POINT('Ctrl Pts',(2.25494028833314,137.654264288147,12.7246474670605));
#77266=CARTESIAN_POINT('Ctrl Pts',(2.25571959888999,137.659927685746,12.711577264534));
#77267=CARTESIAN_POINT('Ctrl Pts',(2.25780079451095,137.675428976039,12.6771877600644));
#77268=CARTESIAN_POINT('Ctrl Pts',(2.25911363643615,137.68559037694,12.6560196150069));
#77269=CARTESIAN_POINT('Ctrl Pts',(2.26708123642232,137.749500719644,12.5307023464671));
#77270=CARTESIAN_POINT('Ctrl Pts',(2.27415966659373,137.815086893494,12.4330859538698));
#77271=CARTESIAN_POINT('Ctrl Pts',(2.28385895071946,137.920311904295,12.3110407886912));
#77272=CARTESIAN_POINT('Ctrl Pts',(2.28649165609938,137.950520369593,12.2790398775774));
#77273=CARTESIAN_POINT('Ctrl Pts',(2.29062106322069,138.001237787505,12.2299468122273));
#77274=CARTESIAN_POINT('Ctrl Pts',(2.29215454654415,138.020852036895,12.211970028329));
#77275=CARTESIAN_POINT('Ctrl Pts',(2.29423675454051,138.048753122294,12.1877642157909));
#77276=CARTESIAN_POINT('Ctrl Pts',(2.29481417212436,138.056631474004,12.1810742210004));
#77277=CARTESIAN_POINT('Ctrl Pts',(2.29579641297636,138.07029174004,12.1697212936527));
#77278=CARTESIAN_POINT('Ctrl Pts',(2.29620401253249,138.076039314993,12.1650180339266));
#77279=CARTESIAN_POINT('Ctrl Pts',(2.29708235201722,138.088600276358,12.1548980203329));
#77280=CARTESIAN_POINT('Ctrl Pts',(2.29755196526253,138.095426486923,12.1494980368316));
#77281=CARTESIAN_POINT('Ctrl Pts',(2.29888510429663,138.115104798427,12.1342146113771));
#77282=CARTESIAN_POINT('Ctrl Pts',(2.2997388719371,138.12807384151,12.1244831321404));
#77283=CARTESIAN_POINT('Ctrl Pts',(2.3039489445032,138.193667498271,12.076947107172));
#77284=CARTESIAN_POINT('Ctrl Pts',(2.30713589812369,138.248604495764,12.0424481197653));
#77285=CARTESIAN_POINT('Ctrl Pts',(2.31327779702413,138.359536887051,11.9826593606305));
#77286=CARTESIAN_POINT('Ctrl Pts',(2.31623035240831,138.415191331578,11.9570264076628));
#77287=CARTESIAN_POINT('Ctrl Pts',(2.3221087692099,138.526330276767,11.9140611365669));
#77288=CARTESIAN_POINT('Ctrl Pts',(2.32502237779676,138.581562981292,11.8963978043222));
#77289=CARTESIAN_POINT('Ctrl Pts',(2.32904944521308,138.656459309778,11.8772606827653));
#77290=CARTESIAN_POINT('Ctrl Pts',(2.33006939111661,138.675317164604,11.8728390488385));
#77291=CARTESIAN_POINT('Ctrl Pts',(2.33182061866858,138.707461216137,11.8659722361271));
#77292=CARTESIAN_POINT('Ctrl Pts',(2.33254569395921,138.720703866693,11.8633343392351));
#77293=CARTESIAN_POINT('Ctrl Pts',(2.3340259433531,138.747591822371,11.8583641405755));
#77294=CARTESIAN_POINT('Ctrl Pts',(2.33478133960006,138.761237481902,11.8560414546064));
#77295=CARTESIAN_POINT('Ctrl Pts',(2.33670725600901,138.79582469885,11.8506578873227));
#77296=CARTESIAN_POINT('Ctrl Pts',(2.33788578600493,138.81680299418,11.8478571336295));
#77297=CARTESIAN_POINT('Ctrl Pts',(2.34371292345557,138.919586945369,11.8363973788373));
#77298=CARTESIAN_POINT('Ctrl Pts',(2.3485574759316,139.001952206167,11.8341924141317));
#77299=CARTESIAN_POINT('Ctrl Pts',(2.35776999673555,139.155291462259,11.8430140649857));
#77300=CARTESIAN_POINT('Ctrl Pts',(2.36210085406627,139.226131638434,11.8523162681797));
#77301=CARTESIAN_POINT('Ctrl Pts',(2.36839126025368,139.330413340426,11.8738537033917));
#77302=CARTESIAN_POINT('Ctrl Pts',(2.37043534614109,139.364550994105,11.882195656608));
#77303=CARTESIAN_POINT('Ctrl Pts',(2.37306907709964,139.409344510914,11.8948666630384));
#77304=CARTESIAN_POINT('Ctrl Pts',(2.37370902267679,139.420295105406,11.8981031905725));
#77305=CARTESIAN_POINT('Ctrl Pts',(2.37476487930829,139.438497302472,11.903715442248));
#77306=CARTESIAN_POINT('Ctrl Pts',(2.37518463184687,139.445770127091,11.9060202821745));
#77307=CARTESIAN_POINT('Ctrl Pts',(2.37605246938255,139.460891057036,11.9109427237289));
#77308=CARTESIAN_POINT('Ctrl Pts',(2.37650000128357,139.468735521553,11.9135701601655));
#77309=CARTESIAN_POINT('Ctrl Pts',(2.37772541824389,139.490326547998,11.9210060911159));
#77310=CARTESIAN_POINT('Ctrl Pts',(2.3784956971696,139.504024589974,11.9259535783716));
#77311=CARTESIAN_POINT('Ctrl Pts',(2.38434251093767,139.60869592036,11.9655349895755));
#77312=CARTESIAN_POINT('Ctrl Pts',(2.38900748988419,139.696093046544,12.0089669629706));
#77313=CARTESIAN_POINT('Ctrl Pts',(2.39760626119889,139.845744994916,12.1029839665974));
#77314=CARTESIAN_POINT('Ctrl Pts',(2.40150115951419,139.909403070161,12.1506016419536));
#77315=CARTESIAN_POINT('Ctrl Pts',(2.40684657404106,139.987187405098,12.2193105111532));
#77316=CARTESIAN_POINT('Ctrl Pts',(2.40812101239358,140.005083667629,12.2359344589578));
#77317=CARTESIAN_POINT('Ctrl Pts',(2.4101812790993,140.03291814835,12.2631190121901));
#77318=CARTESIAN_POINT('Ctrl Pts',(2.4109548070105,140.043130219096,12.2733932546015));
#77319=CARTESIAN_POINT('Ctrl Pts',(2.41244528595526,140.06234281667,12.2933054923245));
#77320=CARTESIAN_POINT('Ctrl Pts',(2.41316101199145,140.071368915085,12.3029168922141));
#77321=CARTESIAN_POINT('Ctrl Pts',(2.41483577592686,140.092021011334,12.3255124068903));
#77322=CARTESIAN_POINT('Ctrl Pts',(2.41579886511404,140.103547215887,12.3385846560322));
#77323=CARTESIAN_POINT('Ctrl Pts',(2.41907814192734,140.14161005561,12.3833394642116));
#77324=CARTESIAN_POINT('Ctrl Pts',(2.42143774752584,140.167035759087,12.4159371473718));
#77325=CARTESIAN_POINT('Ctrl Pts',(2.42766446925053,140.229219391161,12.5030262103607));
#77326=CARTESIAN_POINT('Ctrl Pts',(2.43159587364131,140.263746584658,12.5589933090611));
#77327=CARTESIAN_POINT('Ctrl Pts',(2.44049739430663,140.33271927143,12.6897241365367));
#77328=CARTESIAN_POINT('Ctrl Pts',(2.4454679399433,140.364862743131,12.7654640632126));
#77329=CARTESIAN_POINT('Ctrl Pts',(2.45109231771666,140.395450064994,12.8586329154602));
#77330=CARTESIAN_POINT('Ctrl Pts',(2.45199516489703,140.400169710514,12.8738420352965));
#77331=CARTESIAN_POINT('Ctrl Pts',(2.45336820299642,140.407067033628,12.8974216555631));
#77332=CARTESIAN_POINT('Ctrl Pts',(2.45384745113161,140.40942020479,12.9057391034271));
#77333=CARTESIAN_POINT('Ctrl Pts',(2.45473312315506,140.413670089769,12.9212851135362));
#77334=CARTESIAN_POINT('Ctrl Pts',(2.45514049794269,140.415585249132,12.9285077499075));
#77335=CARTESIAN_POINT('Ctrl Pts',(2.45611397160794,140.420063501894,12.9459342246824));
#77336=CARTESIAN_POINT('Ctrl Pts',(2.45667704562606,140.422572019983,12.9561515107088));
#77337=CARTESIAN_POINT('Ctrl Pts',(2.45870326266731,140.431285559853,12.993370809746));
#77338=CARTESIAN_POINT('Ctrl Pts',(2.46013392939336,140.436834013943,13.0205218929193));
#77339=CARTESIAN_POINT('Ctrl Pts',(2.46391819628186,140.449690327572,13.0940148453703));
#77340=CARTESIAN_POINT('Ctrl Pts',(2.46622290348314,140.455547010517,13.1405782999316));
#77341=CARTESIAN_POINT('Ctrl Pts',(2.47406375811669,140.467924889942,13.3009016006718));
#77342=CARTESIAN_POINT('Ctrl Pts',(2.479520579716,140.463406430134,13.4150838475486));
#77343=CARTESIAN_POINT('Ctrl Pts',(2.48657384780218,140.44219234876,13.5498421181231));
#77344=CARTESIAN_POINT('Ctrl Pts',(2.48775310321166,140.438175405704,13.5720133927024));
#77345=CARTESIAN_POINT('Ctrl Pts',(2.48969622194985,140.430816082615,13.6078900142765));
#77346=CARTESIAN_POINT('Ctrl Pts',(2.49045021101467,140.427784483891,13.6216556727881));
#77347=CARTESIAN_POINT('Ctrl Pts',(2.49192856304666,140.421504766341,13.6483296896206));
#77348=CARTESIAN_POINT('Ctrl Pts',(2.4926521625319,140.418278439744,13.661241781066));
#77349=CARTESIAN_POINT('Ctrl Pts',(2.49438700710972,140.410186030904,13.6918472905395));
#77350=CARTESIAN_POINT('Ctrl Pts',(2.49540324434179,140.405162478517,13.7094964061111));
#77351=CARTESIAN_POINT('Ctrl Pts',(2.49914145775699,140.3856708096,13.7733879170323));
#77352=CARTESIAN_POINT('Ctrl Pts',(2.5019255108253,140.369241751737,13.8189951850368));
#77353=CARTESIAN_POINT('Ctrl Pts',(2.50997773036562,140.316356776344,13.945703482937));
#77354=CARTESIAN_POINT('Ctrl Pts',(2.51537525337801,140.27473480582,14.024415152914));
#77355=CARTESIAN_POINT('Ctrl Pts',(2.52399775337936,140.196231888673,14.1449160293077));
#77356=CARTESIAN_POINT('Ctrl Pts',(2.52725565082794,140.163653140279,14.1892503616524));
#77357=CARTESIAN_POINT('Ctrl Pts',(2.53112444036924,140.120359529895,14.2416987678188));
#77358=CARTESIAN_POINT('Ctrl Pts',(2.53185814070649,140.111930261071,14.2516370969016));
#77359=CARTESIAN_POINT('Ctrl Pts',(2.53302452797269,140.098152677373,14.2674481868343));
#77360=CARTESIAN_POINT('Ctrl Pts',(2.53346280805793,140.092887508867,14.2733921080965));
#77361=CARTESIAN_POINT('Ctrl Pts',(2.53432576684646,140.082337840558,14.2851082601725));
#77362=CARTESIAN_POINT('Ctrl Pts',(2.53475052174912,140.077054923951,14.2908815171046));
#77363=CARTESIAN_POINT('Ctrl Pts',(2.53584371726522,140.063232632713,14.3057455798949));
#77364=CARTESIAN_POINT('Ctrl Pts',(2.53650706107763,140.054622723902,14.3147702861604));
#77365=CARTESIAN_POINT('Ctrl Pts',(2.53969122706636,140.01228302441,14.3580287634261));
#77366=CARTESIAN_POINT('Ctrl Pts',(2.54211057309605,139.976993619402,14.3906997831747));
#77367=CARTESIAN_POINT('Ctrl Pts',(2.54746373958457,139.893965405756,14.4602978588967));
#77368=CARTESIAN_POINT('Ctrl Pts',(2.55036831553376,139.845424159169,14.4961285860499));
#77369=CARTESIAN_POINT('Ctrl Pts',(2.55716828842193,139.728267435862,14.571903765268));
#77370=CARTESIAN_POINT('Ctrl Pts',(2.56108155800638,139.658343009659,14.6094638059892));
#77371=CARTESIAN_POINT('Ctrl Pts',(2.56627800431265,139.566583289732,14.6495377101254));
#77372=CARTESIAN_POINT('Ctrl Pts',(2.5673747304241,139.547262904707,14.6574873519514));
#77373=CARTESIAN_POINT('Ctrl Pts',(2.56921771023866,139.514929433858,14.6699889563101));
#77374=CARTESIAN_POINT('Ctrl Pts',(2.5699560558399,139.502010069577,14.6747755942725));
#77375=CARTESIAN_POINT('Ctrl Pts',(2.57143120423961,139.476280225902,14.6838974857424));
#77376=CARTESIAN_POINT('Ctrl Pts',(2.57216771077682,139.463473410209,14.6882389871584));
#77377=CARTESIAN_POINT('Ctrl Pts',(2.57398306513389,139.432014746243,14.6984196248955));
#77378=CARTESIAN_POINT('Ctrl Pts',(2.57506814285162,139.413302941079,14.7040636791332));
#77379=CARTESIAN_POINT('Ctrl Pts',(2.57953817834046,139.336618770665,14.7255282611144));
#77380=CARTESIAN_POINT('Ctrl Pts',(2.58302264742412,139.27781679373,14.7381444641175));
#77381=CARTESIAN_POINT('Ctrl Pts',(2.59009978778521,139.15970191813,14.7559714410965));
#77382=CARTESIAN_POINT('Ctrl Pts',(2.5936839870074,139.100509770264,14.7612511146981));
#77383=CARTESIAN_POINT('Ctrl Pts',(2.60110886981884,138.977218876787,14.7647202482106));
#77384=CARTESIAN_POINT('Ctrl Pts',(2.60494005927591,138.913220346021,14.7623251564652));
#77385=CARTESIAN_POINT('Ctrl Pts',(2.60953934019143,138.833500429977,14.7540878445661));
#77386=CARTESIAN_POINT('Ctrl Pts',(2.61045635642689,138.817448698174,14.7521599885751));
#77387=CARTESIAN_POINT('Ctrl Pts',(2.61184622426581,138.79281680752,14.748786727065));
#77388=CARTESIAN_POINT('Ctrl Pts',(2.61232845875939,138.784212517125,14.747530181319));
#77389=CARTESIAN_POINT('Ctrl Pts',(2.61321669327177,138.768244032571,14.7450526398145));
#77390=CARTESIAN_POINT('Ctrl Pts',(2.61362370017114,138.760877554038,14.7438519376105));
#77391=CARTESIAN_POINT('Ctrl Pts',(2.61459236001744,138.743233843288,14.7408373563039));
#77392=CARTESIAN_POINT('Ctrl Pts',(2.61515107908305,138.732966345954,14.7389698352756));
#77393=CARTESIAN_POINT('Ctrl Pts',(2.61713938730934,138.696149582923,14.7318657110777));
#77394=CARTESIAN_POINT('Ctrl Pts',(2.61853810773955,138.669725479143,14.7260025953688));
#77395=CARTESIAN_POINT('Ctrl Pts',(2.62220547837201,138.599681121623,14.7084091027784));
#77396=CARTESIAN_POINT('Ctrl Pts',(2.6244288972829,138.556414814728,14.6953866860314));
#77397=CARTESIAN_POINT('Ctrl Pts',(2.63237037328822,138.402966457918,14.6413409779586));
#77398=CARTESIAN_POINT('Ctrl Pts',(2.6379887583654,138.297230528857,14.5890920157521));
#77399=CARTESIAN_POINT('Ctrl Pts',(2.64521164228452,138.180458135184,14.5127110224938));
#77400=CARTESIAN_POINT('Ctrl Pts',(2.64636500163808,138.162309689367,14.5002465450273));
#77401=CARTESIAN_POINT('Ctrl Pts',(2.64827679819217,138.133093147334,14.4791949350024));
#77402=CARTESIAN_POINT('Ctrl Pts',(2.64902600158494,138.121854683969,14.4708496792317));
#77403=CARTESIAN_POINT('Ctrl Pts',(2.65050324866083,138.100117631428,14.4542195549148));
#77404=CARTESIAN_POINT('Ctrl Pts',(2.6512306706349,138.089609467871,14.4459494406902));
#77405=CARTESIAN_POINT('Ctrl Pts',(2.65298892542883,138.064685122948,14.425774329069));
#77406=CARTESIAN_POINT('Ctrl Pts',(2.6540250975836,138.050381128817,14.4137350282089));
#77407=CARTESIAN_POINT('Ctrl Pts',(2.65795219338977,137.997616345733,14.3675686866497));
#77408=CARTESIAN_POINT('Ctrl Pts',(2.66091385203213,137.960735266399,14.3316994883801));
#77409=CARTESIAN_POINT('Ctrl Pts',(2.66994083637004,137.856492796377,14.2190447339856));
#77410=CARTESIAN_POINT('Ctrl Pts',(2.6761834058447,137.795199824031,14.1370819223044));
#77411=CARTESIAN_POINT('Ctrl Pts',(2.68460271814688,137.722590502865,14.015287168761));
#77412=CARTESIAN_POINT('Ctrl Pts',(2.68692730425134,137.703642274769,13.9803439403179));
#77413=CARTESIAN_POINT('Ctrl Pts',(2.68986908455229,137.680797122219,13.9337847011799));
#77414=CARTESIAN_POINT('Ctrl Pts',(2.69055017515359,137.675591118539,13.9228325735292));
#77415=CARTESIAN_POINT('Ctrl Pts',(2.69161145163983,137.667600250298,13.9054684069714));
#77416=CARTESIAN_POINT('Ctrl Pts',(2.69199684122509,137.664724277442,13.8990991852561));
#77417=CARTESIAN_POINT('Ctrl Pts',(2.69280690817822,137.658731287118,13.8855693585572));
#77418=CARTESIAN_POINT('Ctrl Pts',(2.69323084901377,137.655625743929,13.8784039226315));
#77419=CARTESIAN_POINT('Ctrl Pts',(2.69431925404384,137.647739328723,13.8598008509167));
#77420=CARTESIAN_POINT('Ctrl Pts',(2.69497870638576,137.643046049485,13.8483264650811));
#77421=CARTESIAN_POINT('Ctrl Pts',(2.69809933896348,137.621293000266,13.793152918644));
#77422=CARTESIAN_POINT('Ctrl Pts',(2.70046390778229,137.606193741402,13.7487066123177));
#77423=CARTESIAN_POINT('Ctrl Pts',(2.70952833111271,137.555655267457,13.572558774906));
#77424=CARTESIAN_POINT('Ctrl Pts',(2.71592526133157,137.536552809664,13.436905793067));
#77425=CARTESIAN_POINT('Ctrl Pts',(2.72296469855451,137.536500109331,13.300565695148));
#77426=CARTESIAN_POINT('Ctrl Pts',(2.1523578980801,137.536219494403,13.3011848097323));
#77427=CARTESIAN_POINT('Ctrl Pts',(2.15550554832557,137.536293154548,13.2472840551289));
#77428=CARTESIAN_POINT('Ctrl Pts',(2.15869901612957,137.539374600405,13.1932720094472));
#77429=CARTESIAN_POINT('Ctrl Pts',(2.1618777162065,137.545442632201,13.1395110595447));
#77430=CARTESIAN_POINT('Ctrl Pts',(2.16505245649291,137.551503104888,13.0858170810754));
#77431=CARTESIAN_POINT('Ctrl Pts',(2.16821217235941,137.56054245299,13.0323735512194));
#77432=CARTESIAN_POINT('Ctrl Pts',(2.17131609025905,137.572501951759,12.9795326602491));
#77433=CARTESIAN_POINT('Ctrl Pts',(2.1744174825726,137.584451719361,12.9267347646876));
#77434=CARTESIAN_POINT('Ctrl Pts',(2.17746166119412,137.599319909126,12.8745368755472));
#77435=CARTESIAN_POINT('Ctrl Pts',(2.18039406670322,137.617070160124,12.8233094345982));
#77436=CARTESIAN_POINT('Ctrl Pts',(2.18316172764799,137.633823189777,12.7749599866193));
#77437=CARTESIAN_POINT('Ctrl Pts',(2.18592960702013,137.652981000612,12.7274166011582));
#77438=CARTESIAN_POINT('Ctrl Pts',(2.18862949130611,137.674558624412,12.6809911398357));
#77439=CARTESIAN_POINT('Ctrl Pts',(2.18878910882343,137.675834296395,12.6782464604008));
#77440=CARTESIAN_POINT('Ctrl Pts',(2.18894848868499,137.677118421965,12.6755057029054));
#77441=CARTESIAN_POINT('Ctrl Pts',(2.18910761679543,137.678411002512,12.6727689372519));
#77442=CARTESIAN_POINT('Ctrl Pts',(2.19196056412663,137.701585187226,12.6237025074072));
#77443=CARTESIAN_POINT('Ctrl Pts',(2.19472252007874,137.727492198735,12.575928224394));
#77444=CARTESIAN_POINT('Ctrl Pts',(2.1974438794689,137.755931673586,12.5297545626452));
#77445=CARTESIAN_POINT('Ctrl Pts',(2.20016620731441,137.784381269248,12.4835644689875));
#77446=CARTESIAN_POINT('Ctrl Pts',(2.20284819104804,137.815365953895,12.4389751052157));
#77447=CARTESIAN_POINT('Ctrl Pts',(2.20553720782205,137.848684385416,12.3962928570608));
#77448=CARTESIAN_POINT('Ctrl Pts',(2.20823134953414,137.882066317804,12.3535292617455));
#77449=CARTESIAN_POINT('Ctrl Pts',(2.2109330428732,137.917791187923,12.3126805278709));
#77450=CARTESIAN_POINT('Ctrl Pts',(2.21370375737088,137.955614718014,12.2740340050254));
#77451=CARTESIAN_POINT('Ctrl Pts',(2.21602203639286,137.987261968722,12.2416981496855));
#77452=CARTESIAN_POINT('Ctrl Pts',(2.21838912584427,138.020377776731,12.2109039054139));
#77453=CARTESIAN_POINT('Ctrl Pts',(2.22084375255782,138.054794553718,12.1818038527325));
#77454=CARTESIAN_POINT('Ctrl Pts',(2.2208448905864,138.054810510228,12.1817903611937));
#77455=CARTESIAN_POINT('Ctrl Pts',(2.2208460286338,138.054826467018,12.1817768700183));
#77456=CARTESIAN_POINT('Ctrl Pts',(2.22084716670001,138.054842424087,12.1817633792064));
#77457=CARTESIAN_POINT('Ctrl Pts',(2.22357929346152,138.093150157043,12.1493763284752));
#77458=CARTESIAN_POINT('Ctrl Pts',(2.22642812310337,138.133235441837,12.1189543861747));
#77459=CARTESIAN_POINT('Ctrl Pts',(2.22933369529822,138.174856196594,12.0906687998612));
#77460=CARTESIAN_POINT('Ctrl Pts',(2.22961559730069,138.178894290753,12.0879244992939));
#77461=CARTESIAN_POINT('Ctrl Pts',(2.22989803342686,138.182946797967,12.0852003090169));
#77462=CARTESIAN_POINT('Ctrl Pts',(2.23018094891673,138.187013471129,12.0824963851001));
#77463=CARTESIAN_POINT('Ctrl Pts',(2.23337406614028,138.232911856263,12.0519786285997));
#77464=CARTESIAN_POINT('Ctrl Pts',(2.23662760472992,138.280620606839,12.024041912797));
#77465=CARTESIAN_POINT('Ctrl Pts',(2.23987572411306,138.329805024634,11.9988660921796));
#77466=CARTESIAN_POINT('Ctrl Pts',(2.2431205475994,138.378939534544,11.9737158177004));
#77467=CARTESIAN_POINT('Ctrl Pts',(2.24635961740638,138.429546607901,11.9513204831712));
#77468=CARTESIAN_POINT('Ctrl Pts',(2.24954747105379,138.481282391603,11.9318213807645));
#77469=CARTESIAN_POINT('Ctrl Pts',(2.25273335069003,138.532986139011,11.9123343527659));
#77470=CARTESIAN_POINT('Ctrl Pts',(2.25586793486043,138.585817172414,11.8957398310716));
#77471=CARTESIAN_POINT('Ctrl Pts',(2.25892958794811,138.63942303065,11.8821445272637));
#77472=CARTESIAN_POINT('Ctrl Pts',(2.26199055592287,138.693016893385,11.8685522657072));
#77473=CARTESIAN_POINT('Ctrl Pts',(2.26497862342163,138.747385219049,11.8579579099369));
#77474=CARTESIAN_POINT('Ctrl Pts',(2.26789695879374,138.802166817994,11.8504345673539));
#77475=CARTESIAN_POINT('Ctrl Pts',(2.27081790052231,138.856997342219,11.8429045056964));
#77476=CARTESIAN_POINT('Ctrl Pts',(2.27366910740785,138.912241854974,11.8384511263189));
#77477=CARTESIAN_POINT('Ctrl Pts',(2.27647771075072,138.967529489259,11.8371125396387));
#77478=CARTESIAN_POINT('Ctrl Pts',(2.27928753489876,139.022841155215,11.83577337112));
#77479=CARTESIAN_POINT('Ctrl Pts',(2.28205500254431,139.078195919884,11.8375520422158));
#77480=CARTESIAN_POINT('Ctrl Pts',(2.2848282455957,139.133214302515,11.8424476371093));
#77481=CARTESIAN_POINT('Ctrl Pts',(2.28760671021388,139.188336275835,11.8473524496138));
#77482=CARTESIAN_POINT('Ctrl Pts',(2.29039147921724,139.243120415904,11.8553864709964));
#77483=CARTESIAN_POINT('Ctrl Pts',(2.29324613297757,139.297178632503,11.8665029888428));
#77484=CARTESIAN_POINT('Ctrl Pts',(2.2955148416726,139.340140881634,11.875337734775));
#77485=CARTESIAN_POINT('Ctrl Pts',(2.29782816447982,139.382644379702,11.8861186741655));
#77486=CARTESIAN_POINT('Ctrl Pts',(2.30022080660466,139.424493347728,11.8987979320856));
#77487=CARTESIAN_POINT('Ctrl Pts',(2.30022183019628,139.424511251055,11.8988033563746));
#77488=CARTESIAN_POINT('Ctrl Pts',(2.30022285380242,139.424529154262,11.8988087810107));
#77489=CARTESIAN_POINT('Ctrl Pts',(2.30022387742307,139.424547057349,11.8988142059941));
#77490=CARTESIAN_POINT('Ctrl Pts',(2.30298533681397,139.472844880835,11.9134493847729));
#77491=CARTESIAN_POINT('Ctrl Pts',(2.30585969637305,139.520448031779,11.9306718051708));
#77492=CARTESIAN_POINT('Ctrl Pts',(2.3087869074351,139.56707767681,11.9503691296638));
#77493=CARTESIAN_POINT('Ctrl Pts',(2.30905673505877,139.571375954606,11.9521848109207));
#77494=CARTESIAN_POINT('Ctrl Pts',(2.30932701176075,139.575665940011,11.9540214911148));
#77495=CARTESIAN_POINT('Ctrl Pts',(2.30959769050828,139.579947402644,11.9558790635485));
#77496=CARTESIAN_POINT('Ctrl Pts',(2.31279923135007,139.630587793168,11.9778501051142));
#77497=CARTESIAN_POINT('Ctrl Pts',(2.31605639029282,139.680039512358,12.0027484103807));
#77498=CARTESIAN_POINT('Ctrl Pts',(2.31930454869308,139.727969586401,12.0303902103241));
#77499=CARTESIAN_POINT('Ctrl Pts',(2.32254956202045,139.775853251508,12.0580052457243));
#77500=CARTESIAN_POINT('Ctrl Pts',(2.3257852564346,139.822218447312,12.0883581874517));
#77501=CARTESIAN_POINT('Ctrl Pts',(2.3289675118827,139.866759328631,12.1212366597246));
#77502=CARTESIAN_POINT('Ctrl Pts',(2.33214793458404,139.911274557654,12.1540961963981));
#77503=CARTESIAN_POINT('Ctrl Pts',(2.33527484322847,139.953967669826,12.1894782608107));
#77504=CARTESIAN_POINT('Ctrl Pts',(2.33832795525588,139.994557015017,12.227144403972));
#77505=CARTESIAN_POINT('Ctrl Pts',(2.34138050668152,140.035138907334,12.2648036310075));
#77506=CARTESIAN_POINT('Ctrl Pts',(2.34435929156306,140.073617767386,12.3047461053593));
#77507=CARTESIAN_POINT('Ctrl Pts',(2.34726876744892,140.109735338471,12.3467076749523));
#77508=CARTESIAN_POINT('Ctrl Pts',(2.35018098300326,140.145886919177,12.3887087570877));
#77509=CARTESIAN_POINT('Ctrl Pts',(2.35302388710834,140.179672592426,12.4327328225378));
#77510=CARTESIAN_POINT('Ctrl Pts',(2.35582576337124,140.210858209603,12.4784883848673));
#77511=CARTESIAN_POINT('Ctrl Pts',(2.35862893969711,140.242058296822,12.5242651776534));
#77512=CARTESIAN_POINT('Ctrl Pts',(2.36139134364931,140.270655589927,12.5717752126333));
#77513=CARTESIAN_POINT('Ctrl Pts',(2.36416200661037,140.296444117614,12.6206983103048));
#77514=CARTESIAN_POINT('Ctrl Pts',(2.36693796007643,140.322281887789,12.6697148252908));
#77515=CARTESIAN_POINT('Ctrl Pts',(2.36972272487537,140.345299592945,12.7201499427997));
#77516=CARTESIAN_POINT('Ctrl Pts',(2.37258035955952,140.365325280923,12.7716510616305));
#77517=CARTESIAN_POINT('Ctrl Pts',(2.37481409186371,140.380978795489,12.8119080313098));
#77518=CARTESIAN_POINT('Ctrl Pts',(2.37709280050146,140.394804689715,12.852815702604));
#77519=CARTESIAN_POINT('Ctrl Pts',(2.37944946662814,140.406739886195,12.8941922688946));
#77520=CARTESIAN_POINT('Ctrl Pts',(2.37945051133745,140.406745177063,12.8942106111127));
#77521=CARTESIAN_POINT('Ctrl Pts',(2.37945155606208,140.406750467561,12.8942289534231));
#77522=CARTESIAN_POINT('Ctrl Pts',(2.37945260080203,140.406755757687,12.894247295826));
#77523=CARTESIAN_POINT('Ctrl Pts',(2.38220585907322,140.4206971066,12.9425859971643));
#77524=CARTESIAN_POINT('Ctrl Pts',(2.38507288664342,140.432105939502,12.9917488432394));
#77525=CARTESIAN_POINT('Ctrl Pts',(2.38799344305808,140.440924128759,13.0414426716851));
#77526=CARTESIAN_POINT('Ctrl Pts',(2.38826395906563,140.441740911937,13.0460455535206));
#77527=CARTESIAN_POINT('Ctrl Pts',(2.38853493431624,140.442535483363,13.050652956791));
#77528=CARTESIAN_POINT('Ctrl Pts',(2.38880632093915,140.443307806116,13.0552646279701));
#77529=CARTESIAN_POINT('Ctrl Pts',(2.39200187028919,140.45240182646,13.1095665780098));
#77530=CARTESIAN_POINT('Ctrl Pts',(2.39525383070685,140.458409324209,13.1644657791954));
#77531=CARTESIAN_POINT('Ctrl Pts',(2.39849724748783,140.461302303971,13.219584694723));
#77532=CARTESIAN_POINT('Ctrl Pts',(2.40173739340044,140.464192366268,13.2746480248204));
#77533=CARTESIAN_POINT('Ctrl Pts',(2.40496867820619,140.463974544526,13.3299306654181));
#77534=CARTESIAN_POINT('Ctrl Pts',(2.40814662138283,140.460659602981,13.3850621023334));
#77535=CARTESIAN_POINT('Ctrl Pts',(2.41132262401351,140.457346685637,13.440159874365));
#77536=CARTESIAN_POINT('Ctrl Pts',(2.41444521352809,140.450940560639,13.495106652687));
#77537=CARTESIAN_POINT('Ctrl Pts',(2.41749370942239,140.441487057421,13.5495379157152));
#77538=CARTESIAN_POINT('Ctrl Pts',(2.42054155654786,140.43203556606,13.6039575948973));
#77539=CARTESIAN_POINT('Ctrl Pts',(2.4235153433608,140.419537968165,13.6578619456573));
#77540=CARTESIAN_POINT('Ctrl Pts',(2.42641909641369,140.40407440464,13.7108920333125));
#77541=CARTESIAN_POINT('Ctrl Pts',(2.42932552104518,140.388596613966,13.7639709109456));
#77542=CARTESIAN_POINT('Ctrl Pts',(2.43216190823954,140.370147239321,13.8161738155769));
#77543=CARTESIAN_POINT('Ctrl Pts',(2.43495610334391,140.348842442441,13.8671471737924));
#77544=CARTESIAN_POINT('Ctrl Pts',(2.43775154983969,140.327528104124,13.9181433606294));
#77545=CARTESIAN_POINT('Ctrl Pts',(2.44050505464395,140.303355499708,13.9679087012849));
#77546=CARTESIAN_POINT('Ctrl Pts',(2.44326526369745,140.276480081452,14.0160976886114));
#77547=CARTESIAN_POINT('Ctrl Pts',(2.44603076905287,140.249553094518,14.0643791411901));
#77548=CARTESIAN_POINT('Ctrl Pts',(2.44880351661884,140.219912496511,14.1110777927002));
#77549=CARTESIAN_POINT('Ctrl Pts',(2.45164733848727,140.187759233284,14.155859031342));
#77550=CARTESIAN_POINT('Ctrl Pts',(2.45393344763572,140.161911668768,14.1918580509974));
#77551=CARTESIAN_POINT('Ctrl Pts',(2.45626596845874,140.134441103001,14.2266180351326));
#77552=CARTESIAN_POINT('Ctrl Pts',(2.45868078854869,140.105475601412,14.2599747072367));
#77553=CARTESIAN_POINT('Ctrl Pts',(2.45868184863585,140.105462885783,14.2599893505552));
#77554=CARTESIAN_POINT('Ctrl Pts',(2.45868290873886,140.105450169866,14.2600039936037));
#77555=CARTESIAN_POINT('Ctrl Pts',(2.45868396885773,140.105437453661,14.2600186363824));
#77556=CARTESIAN_POINT('Ctrl Pts',(2.46143468376256,140.072442422951,14.2980125919953));
#77557=CARTESIAN_POINT('Ctrl Pts',(2.46429959910621,140.037378642723,14.3343270654957));
#77558=CARTESIAN_POINT('Ctrl Pts',(2.46721859668257,140.0004607922,14.3687541847263));
#77559=CARTESIAN_POINT('Ctrl Pts',(2.46749158409374,139.99700819994,14.371973841443));
#77560=CARTESIAN_POINT('Ctrl Pts',(2.46776504451716,139.993539428748,14.3751769845194));
#77561=CARTESIAN_POINT('Ctrl Pts',(2.46803892877915,139.9900546772,14.378363440494));
#77562=CARTESIAN_POINT('Ctrl Pts',(2.4712356635498,139.949381195785,14.4155552620871));
#77563=CARTESIAN_POINT('Ctrl Pts',(2.47448950913879,139.906525063113,14.4504752560248));
#77564=CARTESIAN_POINT('Ctrl Pts',(2.4777354034318,139.861788895216,14.4828945695633));
#77565=CARTESIAN_POINT('Ctrl Pts',(2.48097805793362,139.817097379371,14.5152815247449));
#77566=CARTESIAN_POINT('Ctrl Pts',(2.48421243948382,139.770529740384,14.5451731131655));
#77567=CARTESIAN_POINT('Ctrl Pts',(2.48739394460498,139.722403678361,14.5723769424731));
#77568=CARTESIAN_POINT('Ctrl Pts',(2.49057353314209,139.674306608165,14.599564383806));
#77569=CARTESIAN_POINT('Ctrl Pts',(2.49370017089743,139.624653040574,14.6240674304793));
#77570=CARTESIAN_POINT('Ctrl Pts',(2.4967530713209,139.573774622569,14.6457264304736));
#77571=CARTESIAN_POINT('Ctrl Pts',(2.49980534061447,139.522906722723,14.6673809528759));
#77572=CARTESIAN_POINT('Ctrl Pts',(2.50278390429222,139.470814490295,14.6861925675373));
#77573=CARTESIAN_POINT('Ctrl Pts',(2.50569271488533,139.417843475775,14.7020334705389));
#77574=CARTESIAN_POINT('Ctrl Pts',(2.50860420241418,139.364823712807,14.7178889516912));
#77575=CARTESIAN_POINT('Ctrl Pts',(2.51144593371271,139.310923545508,14.7307680641669));
#77576=CARTESIAN_POINT('Ctrl Pts',(2.5142457157691,139.256503576921,14.7405761469619));
#77577=CARTESIAN_POINT('Ctrl Pts',(2.51704675672904,139.202059138753,14.7503886398967));
#77578=CARTESIAN_POINT('Ctrl Pts',(2.51980609950029,139.147094440689,14.7571269926452));
#77579=CARTESIAN_POINT('Ctrl Pts',(2.52257238304002,139.091984679983,14.7607339012244));
#77580=CARTESIAN_POINT('Ctrl Pts',(2.52534394446532,139.036769773508,14.764347691546));
#77581=CARTESIAN_POINT('Ctrl Pts',(2.52812298668982,138.981409352939,14.7648175137342));
#77582=CARTESIAN_POINT('Ctrl Pts',(2.53097335002254,138.926294221959,14.7621301847635));
#77583=CARTESIAN_POINT('Ctrl Pts',(2.53324011254487,138.882463699763,14.7599930759515));
#77584=CARTESIAN_POINT('Ctrl Pts',(2.53555245154774,138.838788669781,14.7558599980584));
#77585=CARTESIAN_POINT('Ctrl Pts',(2.53794511405316,138.795470381661,14.7497484762756));
#77586=CARTESIAN_POINT('Ctrl Pts',(2.53794616090957,138.795451428705,14.7497458023148));
#77587=CARTESIAN_POINT('Ctrl Pts',(2.53794720778136,138.795432475817,14.7497431279756));
#77588=CARTESIAN_POINT('Ctrl Pts',(2.53794825466852,138.795413522996,14.7497404532578));
#77589=CARTESIAN_POINT('Ctrl Pts',(2.54070220430138,138.745556084026,14.7427043197617));
#77590=CARTESIAN_POINT('Ctrl Pts',(2.5435699260012,138.695983868955,14.7330159221944));
#77591=CARTESIAN_POINT('Ctrl Pts',(2.54649128200699,138.646988471565,14.7207425410881));
#77592=CARTESIAN_POINT('Ctrl Pts',(2.54676281372437,138.642434488972,14.7196017652829));
#77593=CARTESIAN_POINT('Ctrl Pts',(2.54703480879779,138.637885514961,14.7184386845662));
#77594=CARTESIAN_POINT('Ctrl Pts',(2.54730721893744,138.633341798781,14.7172533700387));
#77595=CARTESIAN_POINT('Ctrl Pts',(2.55050471805701,138.58000851059,14.7033403704606));
#77596=CARTESIAN_POINT('Ctrl Pts',(2.55375877581914,138.527395326826,14.6863601882844));
#77597=CARTESIAN_POINT('Ctrl Pts',(2.55700446481932,138.475858827517,14.6664423511454));
#77598=CARTESIAN_POINT('Ctrl Pts',(2.56024692677543,138.424373568654,14.646544317425));
#77599=CARTESIAN_POINT('Ctrl Pts',(2.56348070031214,138.37396267069,14.623714777597));
#77600=CARTESIAN_POINT('Ctrl Pts',(2.5666613306184,138.324960354391,14.5981157372378));
#77601=CARTESIAN_POINT('Ctrl Pts',(2.56984005670062,138.275987375481,14.5725320228685));
#77602=CARTESIAN_POINT('Ctrl Pts',(2.57296556587356,138.228421212674,14.5441822324541));
#77603=CARTESIAN_POINT('Ctrl Pts',(2.57601722018781,138.182576216969,14.5132578854509));
#77604=CARTESIAN_POINT('Ctrl Pts',(2.57906825454379,138.136740534896,14.4823398208777));
#77605=CARTESIAN_POINT('Ctrl Pts',(2.58204546584293,138.092625358433,14.4488482348586));
#77606=CARTESIAN_POINT('Ctrl Pts',(2.58495294617121,138.050525882716,14.413003646619));
#77607=CARTESIAN_POINT('Ctrl Pts',(2.58786311642032,138.008387457722,14.3771258959521));
#77608=CARTESIAN_POINT('Ctrl Pts',(2.59070355255766,137.968268619983,14.3388906818389));
#77609=CARTESIAN_POINT('Ctrl Pts',(2.5935021841686,137.930444939341,14.2985491993314));
#77610=CARTESIAN_POINT('Ctrl Pts',(2.59630208209884,137.892604144315,14.2581894631898));
#77611=CARTESIAN_POINT('Ctrl Pts',(2.59906042738604,137.857060881683,14.2157213699025));
#77612=CARTESIAN_POINT('Ctrl Pts',(2.60182595290597,137.824067298388,14.1714287029391));
#77613=CARTESIAN_POINT('Ctrl Pts',(2.60459676467958,137.791010648436,14.1270513713172));
#77614=CARTESIAN_POINT('Ctrl Pts',(2.60737529898325,137.760513964324,14.0808422637597));
#77615=CARTESIAN_POINT('Ctrl Pts',(2.6102254451594,137.732800829309,14.0331222855858));
#77616=CARTESIAN_POINT('Ctrl Pts',(2.61249014724905,137.71078020619,13.9952043937973));
#77617=CARTESIAN_POINT('Ctrl Pts',(2.61480053283759,137.690516653433,13.9563332651505));
#77618=CARTESIAN_POINT('Ctrl Pts',(2.61719125755502,137.67210465407,13.9166869331431));
#77619=CARTESIAN_POINT('Ctrl Pts',(2.61719230777412,137.672096565881,13.9166695169452));
#77620=CARTESIAN_POINT('Ctrl Pts',(2.61719335800871,137.672088478049,13.9166521005974));
#77621=CARTESIAN_POINT('Ctrl Pts',(2.61719440825882,137.672080390573,13.9166346840999));
#77622=CARTESIAN_POINT('Ctrl Pts',(2.62005550770341,137.650048427832,13.8691885269283));
#77623=CARTESIAN_POINT('Ctrl Pts',(2.62303773388409,137.630602442131,13.8204822350955));
#77624=CARTESIAN_POINT('Ctrl Pts',(2.62607496753421,137.61383739867,13.7708069211651));
#77625=CARTESIAN_POINT('Ctrl Pts',(2.62650186804912,137.611480976178,13.7638247724277));
#77626=CARTESIAN_POINT('Ctrl Pts',(2.62692985528643,137.609177515152,13.756823563917));
#77627=CARTESIAN_POINT('Ctrl Pts',(2.62735874564581,137.606927273515,13.7498041862546));
#77628=CARTESIAN_POINT('Ctrl Pts',(2.63065497843165,137.589633062772,13.6958568258598));
#77629=CARTESIAN_POINT('Ctrl Pts',(2.63400382996392,137.575481918602,13.6408301187835));
#77630=CARTESIAN_POINT('Ctrl Pts',(2.63733875522186,137.564555143265,13.5850899660694));
#77631=CARTESIAN_POINT('Ctrl Pts',(2.63751513242926,137.563977249018,13.5821419862152));
#77632=CARTESIAN_POINT('Ctrl Pts',(2.63769147068306,137.563408376539,13.5791920225578));
#77633=CARTESIAN_POINT('Ctrl Pts',(2.63786776013896,137.562848538649,13.5762401332085));
#77634=CARTESIAN_POINT('Ctrl Pts',(2.64136237790394,137.551750770921,13.5177242968082));
#77635=CARTESIAN_POINT('Ctrl Pts',(2.64483743486126,137.544201557004,13.4584462153631));
#77636=CARTESIAN_POINT('Ctrl Pts',(2.64824438977004,137.54026214309,13.3988283257318));
#77637=CARTESIAN_POINT('Ctrl Pts',(2.65011196726024,137.538102689575,13.3661478143456));
#77638=CARTESIAN_POINT('Ctrl Pts',(2.65195961351415,137.537027408895,13.3333652157989));
#77639=CARTESIAN_POINT('Ctrl Pts',(2.65378340881734,137.537042726446,13.3005506582616));
#77640=CARTESIAN_POINT('Origin',(4.2,139.,13.3));
#77641=CARTESIAN_POINT('',(3.22385647472349,137.536631187551,13.2999996886484));
#77642=CARTESIAN_POINT('',(3.1529262221125,137.5365,13.3000000000405));
#77643=CARTESIAN_POINT('',(4.2,137.5365,13.3));
#77644=CARTESIAN_POINT('Ctrl Pts',(3.22385647472349,137.536631187551,13.2999996886484));
#77645=CARTESIAN_POINT('Ctrl Pts',(3.22068411944641,137.536760431405,13.354271285598));
#77646=CARTESIAN_POINT('Ctrl Pts',(3.21753929924093,137.539896871394,13.4085937059785));
#77647=CARTESIAN_POINT('Ctrl Pts',(3.21445595208442,137.546016699963,13.4626125813809));
#77648=CARTESIAN_POINT('Ctrl Pts',(3.21134941699173,137.552182551956,13.5170376991468));
#77649=CARTESIAN_POINT('Ctrl Pts',(3.2083053657435,137.561376771111,13.5711546984878));
#77650=CARTESIAN_POINT('Ctrl Pts',(3.20533500370354,137.573539915795,13.6246062603118));
#77651=CARTESIAN_POINT('Ctrl Pts',(3.20236504498896,137.585701408928,13.6780505643094));
#77652=CARTESIAN_POINT('Ctrl Pts',(3.19946871180647,137.600831087743,13.730829527396));
#77653=CARTESIAN_POINT('Ctrl Pts',(3.19663342159315,137.618834381317,13.7825917897771));
#77654=CARTESIAN_POINT('Ctrl Pts',(3.19379538095205,137.636855139331,13.8344042651358));
#77655=CARTESIAN_POINT('Ctrl Pts',(3.19101832874183,137.657755277935,13.8851979101551));
#77656=CARTESIAN_POINT('Ctrl Pts',(3.18826740825234,137.681402812034,13.9346279494016));
#77657=CARTESIAN_POINT('Ctrl Pts',(3.18551498551653,137.705063259781,13.9840849818293));
#77658=CARTESIAN_POINT('Ctrl Pts',(3.18278837109439,137.731474407983,14.0321766444765));
#77659=CARTESIAN_POINT('Ctrl Pts',(3.18003428613028,137.760463205269,14.0785683654693));
#77660=CARTESIAN_POINT('Ctrl Pts',(3.17743948609428,137.787775409948,14.1222769804435));
#77661=CARTESIAN_POINT('Ctrl Pts',(3.17481977800385,137.817376122555,14.1644767214396));
#77662=CARTESIAN_POINT('Ctrl Pts',(3.17212111534149,137.849081944602,14.2048998818061));
#77663=CARTESIAN_POINT('Ctrl Pts',(3.17195027196522,137.851089134964,14.207458937924));
#77664=CARTESIAN_POINT('Ctrl Pts',(3.17177911215989,137.853104763532,14.2100108912797));
#77665=CARTESIAN_POINT('Ctrl Pts',(3.171607622213,137.855128784553,14.2125556809621));
#77666=CARTESIAN_POINT('Ctrl Pts',(3.17028440112709,137.870746185698,14.2321913472384));
#77667=CARTESIAN_POINT('Ctrl Pts',(3.16894142083759,137.886862460427,14.251399619855));
#77668=CARTESIAN_POINT('Ctrl Pts',(3.16757219701131,137.903452644182,14.2701512175302));
#77669=CARTESIAN_POINT('Ctrl Pts',(3.16757114655029,137.90346537208,14.2701656036532));
#77670=CARTESIAN_POINT('Ctrl Pts',(3.16757009607383,137.903478100257,14.2701799895075));
#77671=CARTESIAN_POINT('Ctrl Pts',(3.16756904558192,137.903490828713,14.2701943750933));
#77672=CARTESIAN_POINT('Ctrl Pts',(3.16481615624691,137.936846659555,14.3078928334693));
#77673=CARTESIAN_POINT('Ctrl Pts',(3.16194936692662,137.972256761486,14.3438918429709));
#77674=CARTESIAN_POINT('Ctrl Pts',(3.15902882320879,138.00950437876,14.377985337582));
#77675=CARTESIAN_POINT('Ctrl Pts',(3.15875699094376,138.012971234644,14.3811586206273));
#77676=CARTESIAN_POINT('Ctrl Pts',(3.15848469299766,138.016453972372,14.3843153897995));
#77677=CARTESIAN_POINT('Ctrl Pts',(3.15821197786757,138.019952394499,14.3874554757464));
#77678=CARTESIAN_POINT('Ctrl Pts',(3.15501496723241,138.060964027196,14.4242663712924));
#77679=CARTESIAN_POINT('Ctrl Pts',(3.15176125240872,138.104136728251,14.4587859943268));
#77680=CARTESIAN_POINT('Ctrl Pts',(3.14851580474113,138.149165919676,14.4907883258101));
#77681=CARTESIAN_POINT('Ctrl Pts',(3.14527359382322,138.194150202591,14.5227587407299));
#77682=CARTESIAN_POINT('Ctrl Pts',(3.14203997002484,138.240987117066,14.552217206911));
#77683=CARTESIAN_POINT('Ctrl Pts',(3.13885943606447,138.2893573173,14.5789742687615));
#77684=CARTESIAN_POINT('Ctrl Pts',(3.13568081490621,138.337698427254,14.6057152386712));
#77685=CARTESIAN_POINT('Ctrl Pts',(3.13255535717331,138.387570931696,14.6297581791116));
#77686=CARTESIAN_POINT('Ctrl Pts',(3.12950375096041,138.438641819003,14.6509464862624));
#77687=CARTESIAN_POINT('Ctrl Pts',(3.126452771915,138.489702210198,14.6721304387827));
#77688=CARTESIAN_POINT('Ctrl Pts',(3.1234756124121,138.541960479639,14.6904608938436));
#77689=CARTESIAN_POINT('Ctrl Pts',(3.1205682308823,138.595069988531,14.7058132196658));
#77690=CARTESIAN_POINT('Ctrl Pts',(3.11765816577949,138.648228518594,14.7211797160009));
#77691=CARTESIAN_POINT('Ctrl Pts',(3.11481788186344,138.702239862291,14.7335623955975));
#77692=CARTESIAN_POINT('Ctrl Pts',(3.11201949749925,138.756742619446,14.7428699123261));
#77693=CARTESIAN_POINT('Ctrl Pts',(3.10921985102585,138.811269958082,14.7521816268706));
#77694=CARTESIAN_POINT('Ctrl Pts',(3.10646185266845,138.866289141069,14.7584150555775));
#77695=CARTESIAN_POINT('Ctrl Pts',(3.10369680928727,138.921424509622,14.7615163550724));
#77696=CARTESIAN_POINT('Ctrl Pts',(3.10092648080941,138.976665263774,14.764623582383));
#77697=CARTESIAN_POINT('Ctrl Pts',(3.09814856626772,139.032022539742,14.7645861327575));
#77698=CARTESIAN_POINT('Ctrl Pts',(3.09529919866355,139.087105474071,14.7613944447161));
#77699=CARTESIAN_POINT('Ctrl Pts',(3.09303102401316,139.130952998388,14.7588537736223));
#77700=CARTESIAN_POINT('Ctrl Pts',(3.09071710096498,139.17462632544,14.7543150943676));
#77701=CARTESIAN_POINT('Ctrl Pts',(3.08832258410537,139.217923813411,14.7477978745243));
#77702=CARTESIAN_POINT('Ctrl Pts',(3.08832153365373,139.217942807605,14.7477950154823));
#77703=CARTESIAN_POINT('Ctrl Pts',(3.08832048318658,139.217961801727,14.7477921560598));
#77704=CARTESIAN_POINT('Ctrl Pts',(3.08831943270391,139.217980795777,14.7477892962568));
#77705=CARTESIAN_POINT('Ctrl Pts',(3.08556654185288,139.267756530636,14.7402949075103));
#77706=CARTESIAN_POINT('Ctrl Pts',(3.0826997512446,139.317223062877,14.7301523923613));
#77707=CARTESIAN_POINT('Ctrl Pts',(3.07977920653119,139.366089589428,14.7174316092589));
#77708=CARTESIAN_POINT('Ctrl Pts',(3.07950737589646,139.37063785704,14.7162476182968));
#77709=CARTESIAN_POINT('Ctrl Pts',(3.07923507958909,139.375180901625,14.7150413192777));
#77710=CARTESIAN_POINT('Ctrl Pts',(3.0789623661053,139.379718473696,14.7138127858175));
#77711=CARTESIAN_POINT('Ctrl Pts',(3.0757653562098,139.432912260124,14.6994107343506));
#77712=CARTESIAN_POINT('Ctrl Pts',(3.07251164249836,139.485358235846,14.6819491181184));
#77713=CARTESIAN_POINT('Ctrl Pts',(3.06926619619694,139.53670109826,14.661560649424));
#77714=CARTESIAN_POINT('Ctrl Pts',(3.06602398663132,139.587992755612,14.6411925144774));
#77715=CARTESIAN_POINT('Ctrl Pts',(3.0627903644374,139.638183685255,14.6179036707393));
#77716=CARTESIAN_POINT('Ctrl Pts',(3.05960983216241,139.68694123977,14.5918591061032));
#77717=CARTESIAN_POINT('Ctrl Pts',(3.05643121267842,139.735669471203,14.5658302048229));
#77718=CARTESIAN_POINT('Ctrl Pts',(3.05330575669995,139.782966131404,14.537049004985));
#77719=CARTESIAN_POINT('Ctrl Pts',(3.05025415211496,139.828518712385,14.5057098269839));
#77720=CARTESIAN_POINT('Ctrl Pts',(3.04720317468954,139.874061931492,14.474377089747));
#77721=CARTESIAN_POINT('Ctrl Pts',(3.04422601667987,139.917861750206,14.4404874154542));
#77722=CARTESIAN_POINT('Ctrl Pts',(3.04131863629093,139.95962508268,14.4042639462185));
#77723=CARTESIAN_POINT('Ctrl Pts',(3.03840857232731,140.00142696361,14.3680070419409));
#77724=CARTESIAN_POINT('Ctrl Pts',(3.03556828919654,140.041188441112,14.3294119289375));
#77725=CARTESIAN_POINT('Ctrl Pts',(3.03276990503546,140.078636337172,14.2887322372334));
#77726=CARTESIAN_POINT('Ctrl Pts',(3.02997025876238,140.116101122779,14.2480341983959));
#77727=CARTESIAN_POINT('Ctrl Pts',(3.02721226002056,140.151249940328,14.2052495210673));
#77728=CARTESIAN_POINT('Ctrl Pts',(3.02444721546737,140.183833332194,14.1606641943811));
#77729=CARTESIAN_POINT('Ctrl Pts',(3.02167688582266,140.216479003784,14.1159936475375));
#77730=CARTESIAN_POINT('Ctrl Pts',(3.0188989693198,140.246548902012,14.0695153461368));
#77731=CARTESIAN_POINT('Ctrl Pts',(3.01604959882231,140.27382246456,14.0215521186743));
#77732=CARTESIAN_POINT('Ctrl Pts',(3.01378142952579,140.295532894015,13.9833722049044));
#77733=CARTESIAN_POINT('Ctrl Pts',(3.0114675115503,140.315471807703,13.9442520438436));
#77734=CARTESIAN_POINT('Ctrl Pts',(3.00907299981926,140.333545898687,13.9043714450552));
#77735=CARTESIAN_POINT('Ctrl Pts',(3.00907194934552,140.333553827802,13.9043539494123));
#77736=CARTESIAN_POINT('Ctrl Pts',(3.00907089885626,140.333561756558,13.9043364536229));
#77737=CARTESIAN_POINT('Ctrl Pts',(3.00906984835148,140.333569684956,13.9043189576868));
#77738=CARTESIAN_POINT('Ctrl Pts',(3.00631696071253,140.354346352467,13.8584701931279));
#77739=CARTESIAN_POINT('Ctrl Pts',(3.00345017312882,140.372732489355,13.811440968349));
#77740=CARTESIAN_POINT('Ctrl Pts',(3.00052963124722,140.388628595016,13.7635133215497));
#77741=CARTESIAN_POINT('Ctrl Pts',(3.00025780009716,140.390108134382,13.7590524276891));
#77742=CARTESIAN_POINT('Ctrl Pts',(2.99998550327013,140.391566111854,13.754583786826));
#77743=CARTESIAN_POINT('Ctrl Pts',(2.99971278926276,140.39300245355,13.7501076483702));
#77744=CARTESIAN_POINT('Ctrl Pts',(2.99651578162392,140.409840588926,13.697634183683));
#77745=CARTESIAN_POINT('Ctrl Pts',(2.99326206992987,140.423704400013,13.6441246280831));
#77746=CARTESIAN_POINT('Ctrl Pts',(2.99001662553576,140.434512062875,13.5899493279236));
#77747=CARTESIAN_POINT('Ctrl Pts',(2.98677441787933,140.44530894707,13.5358280577253));
#77748=CARTESIAN_POINT('Ctrl Pts',(2.98354079748535,140.453056136228,13.4810423815984));
#77749=CARTESIAN_POINT('Ctrl Pts',(2.98036026710783,140.457711212427,13.4259611832007));
#77750=CARTESIAN_POINT('Ctrl Pts',(2.97718164951125,140.462363489049,13.3709131108083));
#77751=CARTESIAN_POINT('Ctrl Pts',(2.97405619551912,140.463927505734,13.3155698631984));
#77752=CARTESIAN_POINT('Ctrl Pts',(2.97100459329227,140.462396412643,13.2602993722482));
#77753=CARTESIAN_POINT('Ctrl Pts',(2.96795361820384,140.46086563421,13.2050402400026));
#77754=CARTESIAN_POINT('Ctrl Pts',(2.96497646290531,140.456240988816,13.1498538608409));
#77755=CARTESIAN_POINT('Ctrl Pts',(2.96206908591755,140.448550375984,13.09510753903));
#77756=CARTESIAN_POINT('Ctrl Pts',(2.9591590252783,140.440852664339,13.0403106836803));
#77757=CARTESIAN_POINT('Ctrl Pts',(2.9563187461703,140.430083150869,12.9859547730942));
#77758=CARTESIAN_POINT('Ctrl Pts',(2.95352036704958,140.41630614684,12.932406982302));
#77759=CARTESIAN_POINT('Ctrl Pts',(2.95072072578499,140.402522929014,12.8788350400229));
#77760=CARTESIAN_POINT('Ctrl Pts',(2.94796273307699,140.385729194159,12.8260721004516));
#77761=CARTESIAN_POINT('Ctrl Pts',(2.94519769584247,140.366029308712,12.7744830271846));
#77762=CARTESIAN_POINT('Ctrl Pts',(2.94242737340597,140.346291768121,12.7227953445142));
#77763=CARTESIAN_POINT('Ctrl Pts',(2.93964946540878,140.323636487067,12.6722863488327));
#77764=CARTESIAN_POINT('Ctrl Pts',(2.93680010481051,140.298214460992,12.623316685582));
#77765=CARTESIAN_POINT('Ctrl Pts',(2.9345318977506,140.277977493071,12.5843348396288));
#77766=CARTESIAN_POINT('Ctrl Pts',(2.93221794105132,140.255988081874,12.5463284777213));
#77767=CARTESIAN_POINT('Ctrl Pts',(2.92982338745721,140.232346399278,12.5094736904392));
#77768=CARTESIAN_POINT('Ctrl Pts',(2.92982233699319,140.232336027935,12.5094575226541));
#77769=CARTESIAN_POINT('Ctrl Pts',(2.92982128651367,140.232325656274,12.5094413550901));
#77770=CARTESIAN_POINT('Ctrl Pts',(2.92982023601862,140.232315284295,12.5094251877472));
#77771=CARTESIAN_POINT('Ctrl Pts',(2.92706734763268,140.205134860668,12.4670576479171));
#77772=CARTESIAN_POINT('Ctrl Pts',(2.92420055875117,140.175663861234,12.4260544440134));
#77773=CARTESIAN_POINT('Ctrl Pts',(2.92128001475791,140.144084878576,12.3866524428245));
#77774=CARTESIAN_POINT('Ctrl Pts',(2.92100817781079,140.141145585671,12.3829850028755));
#77775=CARTESIAN_POINT('Ctrl Pts',(2.92073587516046,140.138188065819,12.3793314465479));
#77776=CARTESIAN_POINT('Ctrl Pts',(2.92046315530633,140.135212488172,12.3756919714781));
#77777=CARTESIAN_POINT('Ctrl Pts',(2.91726613944558,140.100330653251,12.3330274593544));
#77778=CARTESIAN_POINT('Ctrl Pts',(2.91401241847817,140.062961948118,12.2922957355906));
#77779=CARTESIAN_POINT('Ctrl Pts',(2.91076696397492,140.023372690231,12.2537668521489));
#77780=CARTESIAN_POINT('Ctrl Pts',(2.90752474626434,139.983822915941,12.2152763947604));
#77781=CARTESIAN_POINT('Ctrl Pts',(2.90429111498613,139.942057221426,12.1789840897379));
#77782=CARTESIAN_POINT('Ctrl Pts',(2.90111057316057,139.898362124081,12.1451261224966));
#77783=CARTESIAN_POINT('Ctrl Pts',(2.89793194418588,139.854693305971,12.1112885182142));
#77784=CARTESIAN_POINT('Ctrl Pts',(2.89480647825229,139.809097471513,12.0798822067063));
#77785=CARTESIAN_POINT('Ctrl Pts',(2.89175486378769,139.761879679908,12.0511130056982));
#77786=CARTESIAN_POINT('Ctrl Pts',(2.88870387654282,139.714671593307,12.0223497178258));
#77787=CARTESIAN_POINT('Ctrl Pts',(2.88572670878814,139.665842222438,11.9962224953458));
#77788=CARTESIAN_POINT('Ctrl Pts',(2.88281931929704,139.615714995229,11.9729076517383));
#77789=CARTESIAN_POINT('Ctrl Pts',(2.87990924633403,139.565541501427,11.9495712889198));
#77790=CARTESIAN_POINT('Ctrl Pts',(2.87706895484425,139.51406772366,11.9290526836133));
#77791=CARTESIAN_POINT('Ctrl Pts',(2.87427056353783,139.461636780811,11.9114975209264));
#77792=CARTESIAN_POINT('Ctrl Pts',(2.87147091017097,139.409182191871,11.8939344409492));
#77793=CARTESIAN_POINT('Ctrl Pts',(2.86871290555125,139.355769533193,11.879337823445));
#77794=CARTESIAN_POINT('Ctrl Pts',(2.86594785687873,139.301761764499,11.8678184808448));
#77795=CARTESIAN_POINT('Ctrl Pts',(2.86317752323033,139.247650768054,11.8562771207486));
#77796=CARTESIAN_POINT('Ctrl Pts',(2.86039960449443,139.192942405235,11.847825383046));
#77797=CARTESIAN_POINT('Ctrl Pts',(2.85755023400243,139.138021450999,11.8425326536085));
#77798=CARTESIAN_POINT('Ctrl Pts',(2.85528208892008,139.094303481496,11.8383195552138));
#77799=CARTESIAN_POINT('Ctrl Pts',(2.85296819755423,139.050451267159,11.836107494406));
#77800=CARTESIAN_POINT('Ctrl Pts',(2.85057371610521,139.00666704191,11.8359081545861));
#77801=CARTESIAN_POINT('Ctrl Pts',(2.8505726657136,139.006647835003,11.8359080671414));
#77802=CARTESIAN_POINT('Ctrl Pts',(2.85057161530649,139.006628628109,11.8359079800836));
#77803=CARTESIAN_POINT('Ctrl Pts',(2.85057056488386,139.006609421227,11.8359078934127));
#77804=CARTESIAN_POINT('Ctrl Pts',(2.84781766447786,138.95627288889,11.8356807503924));
#77805=CARTESIAN_POINT('Ctrl Pts',(2.8449508656128,138.905835826224,11.8381178567553));
#77806=CARTESIAN_POINT('Ctrl Pts',(2.84203031428587,138.855596313128,11.843194772491));
#77807=CARTESIAN_POINT('Ctrl Pts',(2.8417584925555,138.850920418115,11.8436672915005));
#77808=CARTESIAN_POINT('Ctrl Pts',(2.84148620519934,138.846246263447,11.8441626542865));
#77809=CARTESIAN_POINT('Ctrl Pts',(2.8412135007088,138.841574106924,11.8446808263642));
#77810=CARTESIAN_POINT('Ctrl Pts',(2.83801649368961,138.786800835056,11.8507555329688));
#77811=CARTESIAN_POINT('Ctrl Pts',(2.83476278494475,138.732297363719,11.8599683052966));
#77812=CARTESIAN_POINT('Ctrl Pts',(2.83151734501095,138.678435145453,11.8722424839325));
#77813=CARTESIAN_POINT('Ctrl Pts',(2.82827514173831,138.62462664371,11.8845044215908));
#77814=CARTESIAN_POINT('Ctrl Pts',(2.82504152722837,138.571457979768,11.8998213288386));
#77815=CARTESIAN_POINT('Ctrl Pts',(2.8218610030209,138.519283168349,11.9180811785138));
#77816=CARTESIAN_POINT('Ctrl Pts',(2.81868239155011,138.467139734359,11.936330046891));
#77817=CARTESIAN_POINT('Ctrl Pts',(2.81555694396305,138.415988895149,11.957518199297));
#77818=CARTESIAN_POINT('Ctrl Pts',(2.81250534692587,138.366169262362,11.9815015347655));
#77819=CARTESIAN_POINT('Ctrl Pts',(2.80945437701603,138.316359867904,12.0054799414688));
#77820=CARTESIAN_POINT('Ctrl Pts',(2.80647722567327,138.267881168738,12.0322523984068));
#77821=CARTESIAN_POINT('Ctrl Pts',(2.80356984975818,138.221057003936,12.0616433454123));
#77822=CARTESIAN_POINT('Ctrl Pts',(2.80065979029537,138.174189619789,12.0910614206638));
#77823=CARTESIAN_POINT('Ctrl Pts',(2.79781950945779,138.128979964023,12.1231029482391));
#77824=CARTESIAN_POINT('Ctrl Pts',(2.79502112402402,138.085736878694,12.1575591876438));
#77825=CARTESIAN_POINT('Ctrl Pts',(2.79222147647836,138.042474290116,12.1920309673058));
#77826=CARTESIAN_POINT('Ctrl Pts',(2.78946347288055,138.001180314522,12.2289198602271));
#77827=CARTESIAN_POINT('Ctrl Pts',(2.78669841868601,137.962145316382,12.2679815116619));
#77828=CARTESIAN_POINT('Ctrl Pts',(2.78392807947884,137.923035708326,12.3071178239556));
#77829=CARTESIAN_POINT('Ctrl Pts',(2.78115014858955,137.886194213387,12.3484355025929));
#77830=CARTESIAN_POINT('Ctrl Pts',(2.77830075810428,137.851888291559,12.3916493575631));
#77831=CARTESIAN_POINT('Ctrl Pts',(2.77603263486686,137.824580676515,12.4260477136829));
#77832=CARTESIAN_POINT('Ctrl Pts',(2.77371876190569,137.798879365393,12.4616467894858));
#77833=CARTESIAN_POINT('Ctrl Pts',(2.77132429694915,137.7749041258,12.4982832225735));
#77834=CARTESIAN_POINT('Ctrl Pts',(2.7713232463534,137.774893606421,12.4982992971795));
#77835=CARTESIAN_POINT('Ctrl Pts',(2.77132219574214,137.774883087374,12.4983153719853));
#77836=CARTESIAN_POINT('Ctrl Pts',(2.77132114511536,137.774872568658,12.498331446991));
#77837=CARTESIAN_POINT('Ctrl Pts',(2.76853889632218,137.747017116706,12.5409009551319));
#77838=CARTESIAN_POINT('Ctrl Pts',(2.76564074785638,137.721394723939,12.5850279057137));
#77839=CARTESIAN_POINT('Ctrl Pts',(2.76268845048957,137.698146050023,12.6304457161441));
#77840=CARTESIAN_POINT('Ctrl Pts',(2.76238418499472,137.69575002808,12.6351265022738));
#77841=CARTESIAN_POINT('Ctrl Pts',(2.76207934435818,137.693379216241,12.639820953662));
#77842=CARTESIAN_POINT('Ctrl Pts',(2.76177399617581,137.691033766025,12.6445287472006));
#77843=CARTESIAN_POINT('Ctrl Pts',(2.75849865503538,137.665875110983,12.6950272624956));
#77844=CARTESIAN_POINT('Ctrl Pts',(2.75516560230959,137.643634301116,12.747067073688));
#77845=CARTESIAN_POINT('Ctrl Pts',(2.75184352051216,137.624454846283,12.8002776550356));
#77846=CARTESIAN_POINT('Ctrl Pts',(2.74854042393741,137.605384999293,12.8531841455156));
#77847=CARTESIAN_POINT('Ctrl Pts',(2.7452485086563,137.589341192048,12.9072480674698));
#77848=CARTESIAN_POINT('Ctrl Pts',(2.74201324571513,137.576426943074,12.9620999662645));
#77849=CARTESIAN_POINT('Ctrl Pts',(2.73875008977143,137.563401353171,13.0174247738086));
#77850=CARTESIAN_POINT('Ctrl Pts',(2.73554475485694,137.55355942859,13.0735512801728));
#77851=CARTESIAN_POINT('Ctrl Pts',(2.73241746689613,137.546972783191,13.1300943074508));
#77852=CARTESIAN_POINT('Ctrl Pts',(2.7292901789353,137.540386137791,13.1866373347289));
#77853=CARTESIAN_POINT('Ctrl Pts',(2.72624093881871,137.537054835619,13.2435969411206));
#77854=CARTESIAN_POINT('Ctrl Pts',(2.72326232145936,137.537016258812,13.3005808617436));
#77855=CARTESIAN_POINT('Ctrl Pts',(2.65409617475124,137.536500110378,13.3005683984462));
#77856=CARTESIAN_POINT('Ctrl Pts',(2.65466310222895,137.53649618178,13.2904531293485));
#77857=CARTESIAN_POINT('Ctrl Pts',(2.65522685214119,137.536597123654,13.2803379125779));
#77858=CARTESIAN_POINT('Ctrl Pts',(2.65629969032862,137.536991033323,13.2609808948677));
#77859=CARTESIAN_POINT('Ctrl Pts',(2.65680928418378,137.537266724753,13.2517392689034));
#77860=CARTESIAN_POINT('Ctrl Pts',(2.65798864352025,137.538111914222,13.230243698703));
#77861=CARTESIAN_POINT('Ctrl Pts',(2.6586562914533,137.538747942181,13.2179929681791));
#77862=CARTESIAN_POINT('Ctrl Pts',(2.66005823903909,137.540418745327,13.1921024513624));
#77863=CARTESIAN_POINT('Ctrl Pts',(2.6607913037575,137.54149087262,13.1784662076472));
#77864=CARTESIAN_POINT('Ctrl Pts',(2.6625813274488,137.544599966471,13.144943433684));
#77865=CARTESIAN_POINT('Ctrl Pts',(2.66363146053399,137.546853526745,13.1250795199141));
#77866=CARTESIAN_POINT('Ctrl Pts',(2.66834263008991,137.558919300866,13.0352063348586));
#77867=CARTESIAN_POINT('Ctrl Pts',(2.67185817974909,137.573389465835,12.9659146751024));
#77868=CARTESIAN_POINT('Ctrl Pts',(2.67760590621929,137.605673846808,12.852922305549));
#77869=CARTESIAN_POINT('Ctrl Pts',(2.67986873855879,137.620687616564,12.8085518927537));
#77870=CARTESIAN_POINT('Ctrl Pts',(2.68446266394564,137.655140256846,12.7208335179032));
#77871=CARTESIAN_POINT('Ctrl Pts',(2.68679168278632,137.674613117955,12.6775606887324));
#77872=CARTESIAN_POINT('Ctrl Pts',(2.69017044385885,137.704876242449,12.6181966807565));
#77873=CARTESIAN_POINT('Ctrl Pts',(2.69115674512985,137.713937278149,12.6012554597535));
#77874=CARTESIAN_POINT('Ctrl Pts',(2.69293514062228,137.730594946282,12.5715331521187));
#77875=CARTESIAN_POINT('Ctrl Pts',(2.69372056735556,137.738057906698,12.5586800566001));
#77876=CARTESIAN_POINT('Ctrl Pts',(2.69496257456362,137.749989265911,12.5388336372937));
#77877=CARTESIAN_POINT('Ctrl Pts',(2.69541111258585,137.754323777508,12.5317605783388));
#77878=CARTESIAN_POINT('Ctrl Pts',(2.69626906594014,137.762655742181,12.5184203879017));
#77879=CARTESIAN_POINT('Ctrl Pts',(2.69667774087347,137.766641181133,12.5121462589585));
#77880=CARTESIAN_POINT('Ctrl Pts',(2.6976003643726,137.775679471678,12.4981542605646));
#77881=CARTESIAN_POINT('Ctrl Pts',(2.69811590052295,137.780757850923,12.4904532633158));
#77882=CARTESIAN_POINT('Ctrl Pts',(2.69996300968592,137.799066420869,12.4632526940456));
#77883=CARTESIAN_POINT('Ctrl Pts',(2.701316989524,137.812693799748,12.4440260628534));
#77884=CARTESIAN_POINT('Ctrl Pts',(2.70962298922062,137.897919974233,12.3297347111804));
#77885=CARTESIAN_POINT('Ctrl Pts',(2.7169600934264,137.980432191215,12.2433642657711));
#77886=CARTESIAN_POINT('Ctrl Pts',(2.72717272619952,138.114418587096,12.1335888538252));
#77887=CARTESIAN_POINT('Ctrl Pts',(2.73030172564423,138.158219121381,12.1015946579821));
#77888=CARTESIAN_POINT('Ctrl Pts',(2.73440065065334,138.219574040901,12.0618054945042));
#77889=CARTESIAN_POINT('Ctrl Pts',(2.73545010890919,138.235648984453,12.0518181689181));
#77890=CARTESIAN_POINT('Ctrl Pts',(2.73722048368912,138.263386625297,12.0353217114875));
#77891=CARTESIAN_POINT('Ctrl Pts',(2.73794702910959,138.274952672293,12.0286555044602));
#77892=CARTESIAN_POINT('Ctrl Pts',(2.73932551419404,138.297240955656,12.016212534551));
#77893=CARTESIAN_POINT('Ctrl Pts',(2.73997834871232,138.307947208204,12.0104095702686));
#77894=CARTESIAN_POINT('Ctrl Pts',(2.7416862026952,138.33634314525,11.9954739917205));
#77895=CARTESIAN_POINT('Ctrl Pts',(2.74273328579147,138.354149177648,11.9865673627086));
#77896=CARTESIAN_POINT('Ctrl Pts',(2.74680045128104,138.424776792109,11.9530229530751));
#77897=CARTESIAN_POINT('Ctrl Pts',(2.74972684311173,138.478870596431,11.9311852117206));
#77898=CARTESIAN_POINT('Ctrl Pts',(2.75658664971136,138.61082545062,11.8868752966019));
#77899=CARTESIAN_POINT('Ctrl Pts',(2.76045455453737,138.689525383751,11.8675254566008));
#77900=CARTESIAN_POINT('Ctrl Pts',(2.76691916346528,138.818955910378,11.8468752272363));
#77901=CARTESIAN_POINT('Ctrl Pts',(2.76943850204505,138.868861896941,11.8415245925354));
#77902=CARTESIAN_POINT('Ctrl Pts',(2.7727361839293,138.931476252696,11.838051162252));
#77903=CARTESIAN_POINT('Ctrl Pts',(2.77340375145205,138.944021190969,11.8375170906944));
#77904=CARTESIAN_POINT('Ctrl Pts',(2.77450047489231,138.964380308864,11.8369126730385));
#77905=CARTESIAN_POINT('Ctrl Pts',(2.77492441769269,138.972191155141,11.8367433746979));
#77906=CARTESIAN_POINT('Ctrl Pts',(2.77578175847501,138.987857464013,11.836529291057));
#77907=CARTESIAN_POINT('Ctrl Pts',(2.77621517565434,138.995712668179,11.8364851999461));
#77908=CARTESIAN_POINT('Ctrl Pts',(2.77736132189666,139.016329295621,11.8365354583956));
#77909=CARTESIAN_POINT('Ctrl Pts',(2.77807936048492,139.029089544468,11.8367334876793));
#77910=CARTESIAN_POINT('Ctrl Pts',(2.78160655630213,139.091117674292,11.83850775197));
#77911=CARTESIAN_POINT('Ctrl Pts',(2.7845143431464,139.140283790947,11.84240551233));
#77912=CARTESIAN_POINT('Ctrl Pts',(2.79305492842287,139.281956325216,11.8608713552696));
#77913=CARTESIAN_POINT('Ctrl Pts',(2.79875424541355,139.373391602539,11.881842220141));
#77914=CARTESIAN_POINT('Ctrl Pts',(2.80715768816329,139.509211580132,11.9270503022962));
#77915=CARTESIAN_POINT('Ctrl Pts',(2.81000767554148,139.555402444196,11.9450770447013));
#77916=CARTESIAN_POINT('Ctrl Pts',(2.81381268079047,139.617388208491,11.9729720312145));
#77917=CARTESIAN_POINT('Ctrl Pts',(2.81483299250233,139.634039122419,11.9808465347684));
#77918=CARTESIAN_POINT('Ctrl Pts',(2.81656942509919,139.662416505644,11.9949281703905));
#77919=CARTESIAN_POINT('Ctrl Pts',(2.81729065503355,139.674215078387,12.000984160351));
#77920=CARTESIAN_POINT('Ctrl Pts',(2.8187593730443,139.698257269211,12.0137403928848));
#77921=CARTESIAN_POINT('Ctrl Pts',(2.81950618456959,139.710490644127,12.0204570918312));
#77922=CARTESIAN_POINT('Ctrl Pts',(2.82141990454456,139.741841969805,12.0382587321009));
#77923=CARTESIAN_POINT('Ctrl Pts',(2.82257742735777,139.760808595488,12.049603709255));
#77924=CARTESIAN_POINT('Ctrl Pts',(2.82975714474677,139.878225878183,12.1234986280291));
#77925=CARTESIAN_POINT('Ctrl Pts',(2.83533651420647,139.969157301158,12.1971981830322));
#77926=CARTESIAN_POINT('Ctrl Pts',(2.84325672149494,140.082172223105,12.3136835617332));
#77927=CARTESIAN_POINT('Ctrl Pts',(2.84550338950116,140.112412532608,12.3479208178204));
#77928=CARTESIAN_POINT('Ctrl Pts',(2.84920294174542,140.158047288461,12.4047348788046));
#77929=CARTESIAN_POINT('Ctrl Pts',(2.85060947145878,140.174496691428,12.426426586926));
#77930=CARTESIAN_POINT('Ctrl Pts',(2.85260507176628,140.196392294626,12.4570371998088));
#77931=CARTESIAN_POINT('Ctrl Pts',(2.8531628421868,140.202363019898,12.4655756709428));
#77932=CARTESIAN_POINT('Ctrl Pts',(2.85412822195039,140.212430002699,12.4803044313401));
#77933=CARTESIAN_POINT('Ctrl Pts',(2.85453288178863,140.2165711873,12.4864633496416));
#77934=CARTESIAN_POINT('Ctrl Pts',(2.85541341923085,140.225409982253,12.4998271485266));
#77935=CARTESIAN_POINT('Ctrl Pts',(2.85589024979634,140.230090984303,12.5070420064163));
#77936=CARTESIAN_POINT('Ctrl Pts',(2.8572580028558,140.243230298316,12.5276900461691));
#77937=CARTESIAN_POINT('Ctrl Pts',(2.85815794375411,140.251533787627,12.5412198102772));
#77938=CARTESIAN_POINT('Ctrl Pts',(2.86345950924891,140.298599510435,12.6207839209644));
#77939=CARTESIAN_POINT('Ctrl Pts',(2.86807804453755,140.332349071655,12.6896398307197));
#77940=CARTESIAN_POINT('Ctrl Pts',(2.8768767107194,140.386155422329,12.8254120832268));
#77941=CARTESIAN_POINT('Ctrl Pts',(2.88104703903556,140.407124255955,12.8917559498268));
#77942=CARTESIAN_POINT('Ctrl Pts',(2.88758115878448,140.433223739487,13.0008021880647));
#77943=CARTESIAN_POINT('Ctrl Pts',(2.89001846051829,140.441331184998,13.0426781319569));
#77944=CARTESIAN_POINT('Ctrl Pts',(2.89337888469893,140.450177806088,13.1022014841772));
#77945=CARTESIAN_POINT('Ctrl Pts',(2.89434870276218,140.452444387427,13.1195969475888));
#77946=CARTESIAN_POINT('Ctrl Pts',(2.89602712253877,140.455859424193,13.1500737646765));
#77947=CARTESIAN_POINT('Ctrl Pts',(2.89673995344613,140.457145557949,13.1631373766263));
#77948=CARTESIAN_POINT('Ctrl Pts',(2.89821668761868,140.459463330673,13.1904424254939));
#77949=CARTESIAN_POINT('Ctrl Pts',(2.89897950928965,140.46046266441,13.2046852522793));
#77950=CARTESIAN_POINT('Ctrl Pts',(2.90099187817338,140.46256615626,13.2426048687142));
#77951=CARTESIAN_POINT('Ctrl Pts',(2.90223001924217,140.463303874755,13.26629814552));
#77952=CARTESIAN_POINT('Ctrl Pts',(2.9094568083219,140.464261335976,13.4064165844386));
#77953=CARTESIAN_POINT('Ctrl Pts',(2.91501336329876,140.45116397503,13.5225085848602));
#77954=CARTESIAN_POINT('Ctrl Pts',(2.92283902460782,140.414411526104,13.6783984440591));
#77955=CARTESIAN_POINT('Ctrl Pts',(2.92499599039625,140.402471864323,13.7204968826564));
#77956=CARTESIAN_POINT('Ctrl Pts',(2.92856583338239,140.380302880672,13.7871324598516));
#77957=CARTESIAN_POINT('Ctrl Pts',(2.9299362479539,140.371259397808,13.8120366964607));
#77958=CARTESIAN_POINT('Ctrl Pts',(2.9318887634983,140.357762059052,13.8462791356142));
#77959=CARTESIAN_POINT('Ctrl Pts',(2.93244131394557,140.353877195534,13.8558374134105));
#77960=CARTESIAN_POINT('Ctrl Pts',(2.93340077535806,140.347029585564,13.8721874161956));
#77961=CARTESIAN_POINT('Ctrl Pts',(2.93380484041928,140.344115787591,13.8789990427618));
#77962=CARTESIAN_POINT('Ctrl Pts',(2.93468801771395,140.337685040656,13.8937220988875));
#77963=CARTESIAN_POINT('Ctrl Pts',(2.93516814755004,140.33414958617,13.9016245280045));
#77964=CARTESIAN_POINT('Ctrl Pts',(2.93655451516751,140.323821717461,13.9241705520232));
#77965=CARTESIAN_POINT('Ctrl Pts',(2.93747013309247,140.316857042938,13.9387333579756));
#77966=CARTESIAN_POINT('Ctrl Pts',(2.94208421657747,140.280971976747,14.0106847079453));
#77967=CARTESIAN_POINT('Ctrl Pts',(2.9459331378894,140.248536099458,14.066236497296));
#77968=CARTESIAN_POINT('Ctrl Pts',(2.9532518798441,140.180466565949,14.1669576837337));
#77969=CARTESIAN_POINT('Ctrl Pts',(2.95671175038683,140.145612332033,14.2125183613962));
#77970=CARTESIAN_POINT('Ctrl Pts',(2.96377187406115,140.067869740671,14.3026436146242));
#77971=CARTESIAN_POINT('Ctrl Pts',(2.96735488027574,140.024646320557,14.3467766592538));
#77972=CARTESIAN_POINT('Ctrl Pts',(2.97192116683008,139.964184379563,14.4011653561232));
#77973=CARTESIAN_POINT('Ctrl Pts',(2.97301007442118,139.949345356427,14.4139838895466));
#77974=CARTESIAN_POINT('Ctrl Pts',(2.97482649388754,139.923884265713,14.4350998019601));
#77975=CARTESIAN_POINT('Ctrl Pts',(2.97556036080566,139.913397368437,14.4435554036328));
#77976=CARTESIAN_POINT('Ctrl Pts',(2.97702583341629,139.892057794421,14.4602806765246));
#77977=CARTESIAN_POINT('Ctrl Pts',(2.97775721775671,139.881203237585,14.4685457749596));
#77978=CARTESIAN_POINT('Ctrl Pts',(2.97957384348168,139.853741406549,14.4888560345353));
#77979=CARTESIAN_POINT('Ctrl Pts',(2.98065155127362,139.836993233847,14.5007062260942));
#77980=CARTESIAN_POINT('Ctrl Pts',(2.98535763085779,139.761944831812,14.5514731919838));
#77981=CARTESIAN_POINT('Ctrl Pts',(2.98884420383262,139.701139044483,14.5865265017309));
#77982=CARTESIAN_POINT('Ctrl Pts',(2.99725695836799,139.54638388673,14.6614961549644));
#77983=CARTESIAN_POINT('Ctrl Pts',(3.00208917402969,139.45034000052,14.6962082373129));
#77984=CARTESIAN_POINT('Ctrl Pts',(3.00845945604121,139.329623909149,14.7260740875111));
#77985=CARTESIAN_POINT('Ctrl Pts',(3.0096316025172,139.307646032047,14.7309762539674));
#77986=CARTESIAN_POINT('Ctrl Pts',(3.01134622464625,139.27603424709,14.737265380843));
#77987=CARTESIAN_POINT('Ctrl Pts',(3.0118678853092,139.266485109035,14.7390664879663));
#77988=CARTESIAN_POINT('Ctrl Pts',(3.01275555679849,139.250369793641,14.7419401764803));
#77989=CARTESIAN_POINT('Ctrl Pts',(3.01311877650576,139.243813073562,14.7430633005873));
#77990=CARTESIAN_POINT('Ctrl Pts',(3.01396417515042,139.228641984634,14.7455556603524));
#77991=CARTESIAN_POINT('Ctrl Pts',(3.01444806219066,139.220023048526,14.7468925926079));
#77992=CARTESIAN_POINT('Ctrl Pts',(3.01585586906362,139.19511408884,14.7505286584277));
#77993=CARTESIAN_POINT('Ctrl Pts',(3.01678959482598,139.178797036445,14.7526301905503));
#77994=CARTESIAN_POINT('Ctrl Pts',(3.02181008430347,139.091915682594,14.762334001119));
#77995=CARTESIAN_POINT('Ctrl Pts',(3.02607930365139,139.020907767063,14.7650702033945));
#77996=CARTESIAN_POINT('Ctrl Pts',(3.03473190503188,138.877368272342,14.7601621163864));
#77997=CARTESIAN_POINT('Ctrl Pts',(3.03910234764817,138.805029774772,14.7522740813092));
#77998=CARTESIAN_POINT('Ctrl Pts',(3.04589242527088,138.690598122333,14.7310879924214));
#77999=CARTESIAN_POINT('Ctrl Pts',(3.04839359277293,138.647998876187,14.7212100903847));
#78000=CARTESIAN_POINT('Ctrl Pts',(3.05182366753431,138.588868195168,14.7046763825307));
#78001=CARTESIAN_POINT('Ctrl Pts',(3.05280195388958,138.571921231778,14.6996048397633));
#78002=CARTESIAN_POINT('Ctrl Pts',(3.05449005322213,138.542544676056,14.6902301005515));
#78003=CARTESIAN_POINT('Ctrl Pts',(3.05520424054462,138.530073686029,14.6860643495454));
#78004=CARTESIAN_POINT('Ctrl Pts',(3.05667926296593,138.504237892961,14.6770454954315));
#78005=CARTESIAN_POINT('Ctrl Pts',(3.05743908946801,138.490884236955,14.6721645391156));
#78006=CARTESIAN_POINT('Ctrl Pts',(3.05943294751541,138.455745629654,14.6587372663541));
#78007=CARTESIAN_POINT('Ctrl Pts',(3.06065596472053,138.434090504514,14.6498615858537));
#78008=CARTESIAN_POINT('Ctrl Pts',(3.06736980104744,138.314932599652,14.5976510984772));
#78009=CARTESIAN_POINT('Ctrl Pts',(3.07250587343878,138.222184622774,14.5442751730275));
#78010=CARTESIAN_POINT('Ctrl Pts',(3.08016700156831,138.095156833528,14.4513726205349));
#78011=CARTESIAN_POINT('Ctrl Pts',(3.08264732581614,138.055838084481,14.4193559852395));
#78012=CARTESIAN_POINT('Ctrl Pts',(3.08668044558145,137.996739474906,14.365899951849));
#78013=CARTESIAN_POINT('Ctrl Pts',(3.08817605995022,137.975802877911,14.3457984691542));
#78014=CARTESIAN_POINT('Ctrl Pts',(3.09027756541743,137.948013910521,14.3174827290039));
#78015=CARTESIAN_POINT('Ctrl Pts',(3.09084761813261,137.940632407218,14.309795091207));
#78016=CARTESIAN_POINT('Ctrl Pts',(3.09182708370348,137.928231132239,14.2965938632666));
#78017=CARTESIAN_POINT('Ctrl Pts',(3.09223331657872,137.923168228597,14.2911211677208));
#78018=CARTESIAN_POINT('Ctrl Pts',(3.09310845939597,137.912437544027,14.2793426545058));
#78019=CARTESIAN_POINT('Ctrl Pts',(3.09357819541395,137.906782492671,14.2730260042519));
#78020=CARTESIAN_POINT('Ctrl Pts',(3.09490608346451,137.891076360544,14.2551726172246));
#78021=CARTESIAN_POINT('Ctrl Pts',(3.09577249751711,137.881151113502,14.2435271583221));
#78022=CARTESIAN_POINT('Ctrl Pts',(3.10165636424834,137.815741043791,14.1642969007287));
#78023=CARTESIAN_POINT('Ctrl Pts',(3.10696111273656,137.766230359656,14.0920158234387));
#78024=CARTESIAN_POINT('Ctrl Pts',(3.11600860073425,137.692707403977,13.9608893736882));
#78025=CARTESIAN_POINT('Ctrl Pts',(3.11976527131541,137.665511789136,13.9040951885532));
#78026=CARTESIAN_POINT('Ctrl Pts',(3.12575861170288,137.627052130992,13.8083944407724));
#78027=CARTESIAN_POINT('Ctrl Pts',(3.12805351381581,137.613595248694,13.7704604725126));
#78028=CARTESIAN_POINT('Ctrl Pts',(3.13125763417118,137.59664053884,13.7155842872592));
#78029=CARTESIAN_POINT('Ctrl Pts',(3.13220780620945,137.591853244956,13.6990624373537));
#78030=CARTESIAN_POINT('Ctrl Pts',(3.13386404533131,137.583939621216,13.6698328969429));
#78031=CARTESIAN_POINT('Ctrl Pts',(3.13457400445591,137.580690452139,13.6571607353527));
#78032=CARTESIAN_POINT('Ctrl Pts',(3.1360559334785,137.574214301904,13.6304175299124));
#78033=CARTESIAN_POINT('Ctrl Pts',(3.13682663955094,137.571024714405,13.6163388283167));
#78034=CARTESIAN_POINT('Ctrl Pts',(3.13888713540599,137.562988404197,13.5782611420473));
#78035=CARTESIAN_POINT('Ctrl Pts',(3.14016448255719,137.558534624514,13.5541834988602));
#78036=CARTESIAN_POINT('Ctrl Pts',(3.14539148405244,137.542581743376,13.4539380260478));
#78037=CARTESIAN_POINT('Ctrl Pts',(3.14917702522996,137.536500000002,13.3770311563965));
#78038=CARTESIAN_POINT('Ctrl Pts',(3.1529262221125,137.5365,13.3000000000405));
#78039=CARTESIAN_POINT('Origin',(4.2,139.,13.3));
#78040=CARTESIAN_POINT('',(3.72552751600545,137.5365,13.2999999999998));
#78041=CARTESIAN_POINT('',(3.65157748137716,137.5365,13.3000000000035));
#78042=CARTESIAN_POINT('',(4.2,137.5365,13.3));
#78043=CARTESIAN_POINT('',(3.22392529813232,137.53661469332,13.2986845264305));
#78044=CARTESIAN_POINT('Ctrl Pts',(3.72552751600545,137.5365,13.2999999999998));
#78045=CARTESIAN_POINT('Ctrl Pts',(3.72552055759137,137.5365,13.3001317195931));
#78046=CARTESIAN_POINT('Ctrl Pts',(3.72551359830482,137.536500017726,13.3002634393025));
#78047=CARTESIAN_POINT('Ctrl Pts',(3.72491065267735,137.536503098796,13.3116741882147));
#78048=CARTESIAN_POINT('Ctrl Pts',(3.72430858380333,137.53663653343,13.3229524639633));
#78049=CARTESIAN_POINT('Ctrl Pts',(3.72329361321726,137.537076133077,13.3417436126553));
#78050=CARTESIAN_POINT('Ctrl Pts',(3.72288457083917,137.537309867579,13.3492579417754));
#78051=CARTESIAN_POINT('Ctrl Pts',(3.7220183172435,137.537922497249,13.3650392762235));
#78052=CARTESIAN_POINT('Ctrl Pts',(3.72156050455177,137.538313626764,13.3733053269853));
#78053=CARTESIAN_POINT('Ctrl Pts',(3.7202852417732,137.539588415186,13.3961423032577));
#78054=CARTESIAN_POINT('Ctrl Pts',(3.71946034626683,137.540619992297,13.4107036565694));
#78055=CARTESIAN_POINT('Ctrl Pts',(3.71432320836805,137.548314434174,13.5002829870594));
#78056=CARTESIAN_POINT('Ctrl Pts',(3.70979067888011,137.560541757334,13.5747044391791));
#78057=CARTESIAN_POINT('Ctrl Pts',(3.69908558943376,137.602774937851,13.7472999962083));
#78058=CARTESIAN_POINT('Ctrl Pts',(3.69295487081315,137.637483031646,13.8439377666827));
#78059=CARTESIAN_POINT('Ctrl Pts',(3.68579717125114,137.692383641285,13.9576793940163));
#78060=CARTESIAN_POINT('Ctrl Pts',(3.68446083742992,137.703291481434,13.9789328679809));
#78061=CARTESIAN_POINT('Ctrl Pts',(3.68234925070244,137.721588767213,14.012533187052));
#78062=CARTESIAN_POINT('Ctrl Pts',(3.68156261378719,137.72864813472,14.0250539829195));
#78063=CARTESIAN_POINT('Ctrl Pts',(3.68006564595427,137.742547286583,14.0488787691578));
#78064=CARTESIAN_POINT('Ctrl Pts',(3.67935436347111,137.749357901011,14.060198061938));
#78065=CARTESIAN_POINT('Ctrl Pts',(3.67770544614854,137.765625069086,14.0864237681303));
#78066=CARTESIAN_POINT('Ctrl Pts',(3.67677225942952,137.775200003886,14.1012545278744));
#78067=CARTESIAN_POINT('Ctrl Pts',(3.67359972327705,137.808992948077,14.151575141327));
#78068=CARTESIAN_POINT('Ctrl Pts',(3.67140842608218,137.83450470886,14.1861710682816));
#78069=CARTESIAN_POINT('Ctrl Pts',(3.66573573895202,137.905699734204,14.2743133111995));
#78070=CARTESIAN_POINT('Ctrl Pts',(3.66233265239016,137.953784496369,14.3257743966884));
#78071=CARTESIAN_POINT('Ctrl Pts',(3.65527363097964,138.060284532009,14.4244412734167));
#78072=CARTESIAN_POINT('Ctrl Pts',(3.65162457188126,138.119000895709,14.4710131626245));
#78073=CARTESIAN_POINT('Ctrl Pts',(3.64689703122542,138.194366934675,14.5219031118683));
#78074=CARTESIAN_POINT('Ctrl Pts',(3.64604841828823,138.207867439716,14.5306981010816));
#78075=CARTESIAN_POINT('Ctrl Pts',(3.64472167167265,138.22886214242,14.5438866679129));
#78076=CARTESIAN_POINT('Ctrl Pts',(3.64425315092351,138.236255219156,14.5484396421401));
#78077=CARTESIAN_POINT('Ctrl Pts',(3.64337380178454,138.250079308209,14.5567843633872));
#78078=CARTESIAN_POINT('Ctrl Pts',(3.64296404575968,138.256499469596,14.560593087611));
#78079=CARTESIAN_POINT('Ctrl Pts',(3.64197312341593,138.271978611614,14.5696166211277));
#78080=CARTESIAN_POINT('Ctrl Pts',(3.64138909004881,138.281064721753,14.5747837303755));
#78081=CARTESIAN_POINT('Ctrl Pts',(3.63926699591292,138.313981095788,14.5930388544123));
#78082=CARTESIAN_POINT('Ctrl Pts',(3.63769915866345,138.338118497709,14.6055589274622));
#78083=CARTESIAN_POINT('Ctrl Pts',(3.6334457770555,138.403541028122,14.637213004489));
#78084=CARTESIAN_POINT('Ctrl Pts',(3.63072142494503,138.445392932358,14.6551061035238));
#78085=CARTESIAN_POINT('Ctrl Pts',(3.6209558427848,138.597428799279,14.7118821814145));
#78086=CARTESIAN_POINT('Ctrl Pts',(3.61391890020323,138.711367617347,14.7395049836129));
#78087=CARTESIAN_POINT('Ctrl Pts',(3.60607251763857,138.849351620248,14.7558936943484));
#78088=CARTESIAN_POINT('Ctrl Pts',(3.60483865118399,138.871370705246,14.7580041026479));
#78089=CARTESIAN_POINT('Ctrl Pts',(3.60284807813009,138.907410190847,14.7606354313836));
#78090=CARTESIAN_POINT('Ctrl Pts',(3.60208220962205,138.92140459749,14.7614552740624));
#78091=CARTESIAN_POINT('Ctrl Pts',(3.60059865088163,138.948755351319,14.7626635667031));
#78092=CARTESIAN_POINT('Ctrl Pts',(3.59988045837982,138.962109463099,14.7630704175964));
#78093=CARTESIAN_POINT('Ctrl Pts',(3.59817440573133,138.99408991786,14.7636065761001));
#78094=CARTESIAN_POINT('Ctrl Pts',(3.59719198722265,139.012717031029,14.7635632741589));
#78095=CARTESIAN_POINT('Ctrl Pts',(3.59356873524607,139.082118683392,14.7620767930083));
#78096=CARTESIAN_POINT('Ctrl Pts',(3.5909978226926,139.132809921046,14.758346388967));
#78097=CARTESIAN_POINT('Ctrl Pts',(3.58355847560734,139.281477528068,14.7395878839013));
#78098=CARTESIAN_POINT('Ctrl Pts',(3.5788611716942,139.378229244989,14.7172453436941));
#78099=CARTESIAN_POINT('Ctrl Pts',(3.57181336461342,139.512631773826,14.6714537184059));
#78100=CARTESIAN_POINT('Ctrl Pts',(3.56964092242108,139.55265109264,14.6558218319845));
#78101=CARTESIAN_POINT('Ctrl Pts',(3.56672857643548,139.603273016283,14.6334346495559));
#78102=CARTESIAN_POINT('Ctrl Pts',(3.56606837805997,139.614559405581,14.6282706852905));
#78103=CARTESIAN_POINT('Ctrl Pts',(3.56502059078414,139.632143664744,14.6199531125627));
#78104=CARTESIAN_POINT('Ctrl Pts',(3.56463864604462,139.638487009202,14.6168964147185));
#78105=CARTESIAN_POINT('Ctrl Pts',(3.56383025074229,139.65176565834,14.6103792764037));
#78106=CARTESIAN_POINT('Ctrl Pts',(3.56340317861143,139.658695919349,14.606909330829));
#78107=CARTESIAN_POINT('Ctrl Pts',(3.56230071818509,139.676380609222,14.5978783087148));
#78108=CARTESIAN_POINT('Ctrl Pts',(3.56162074833845,139.687094055567,14.5922385893897));
#78109=CARTESIAN_POINT('Ctrl Pts',(3.55850035494803,139.735453641193,14.5660099913516));
#78110=CARTESIAN_POINT('Ctrl Pts',(3.5559844134253,139.77225065949,14.5439058246684));
#78111=CARTESIAN_POINT('Ctrl Pts',(3.54660646222448,139.903650575853,14.4568937409475));
#78112=CARTESIAN_POINT('Ctrl Pts',(3.53958601907467,139.991518692225,14.3825355455001));
#78113=CARTESIAN_POINT('Ctrl Pts',(3.53068345530036,140.096149901422,14.270452755276));
#78114=CARTESIAN_POINT('Ctrl Pts',(3.52848126669326,140.121372687485,14.2411943659893));
#78115=CARTESIAN_POINT('Ctrl Pts',(3.52535840073494,140.156190718643,14.1974158556493));
#78116=CARTESIAN_POINT('Ctrl Pts',(3.52440094497153,140.16672992276,14.1836704813028));
#78117=CARTESIAN_POINT('Ctrl Pts',(3.52273025812501,140.184871028997,14.1591200656308));
#78118=CARTESIAN_POINT('Ctrl Pts',(3.52201311119488,140.192575124548,14.1483933231709));
#78119=CARTESIAN_POINT('Ctrl Pts',(3.520526415383,140.208365060775,14.1257681424408));
#78120=CARTESIAN_POINT('Ctrl Pts',(3.51975798039364,140.216422809703,14.1138517759384));
#78121=CARTESIAN_POINT('Ctrl Pts',(3.51772762967691,140.23742019116,14.0817906784012));
#78122=CARTESIAN_POINT('Ctrl Pts',(3.51647738340998,140.25004364801,14.0614436007363));
#78123=CARTESIAN_POINT('Ctrl Pts',(3.51141730825231,140.299727651289,13.9767922718665));
#78124=CARTESIAN_POINT('Ctrl Pts',(3.50775942042999,140.332372005345,13.9100212336995));
#78125=CARTESIAN_POINT('Ctrl Pts',(3.49997472682672,140.391443554923,13.7615600108478));
#78126=CARTESIAN_POINT('Ctrl Pts',(3.49587678859058,140.416040595909,13.6794467112804));
#78127=CARTESIAN_POINT('Ctrl Pts',(3.4902068559564,140.438571477507,13.5702206049436));
#78128=CARTESIAN_POINT('Ctrl Pts',(3.48886331304834,140.443140912839,13.5446451007436));
#78129=CARTESIAN_POINT('Ctrl Pts',(3.48692857706182,140.448601916939,13.5085558129043));
#78130=CARTESIAN_POINT('Ctrl Pts',(3.48636524076321,140.450064366232,13.4981321823053));
#78131=CARTESIAN_POINT('Ctrl Pts',(3.48539139343094,140.45237283916,13.4802810493853));
#78132=CARTESIAN_POINT('Ctrl Pts',(3.48498391022247,140.453274607272,13.4728613175211));
#78133=CARTESIAN_POINT('Ctrl Pts',(3.48409820474165,140.455096506983,13.4568473815084));
#78134=CARTESIAN_POINT('Ctrl Pts',(3.48361903435778,140.455997365785,13.4482518426327));
#78135=CARTESIAN_POINT('Ctrl Pts',(3.48222001330599,140.458386037709,13.4233331643838));
#78136=CARTESIAN_POINT('Ctrl Pts',(3.48129033998743,140.459675783735,13.4069928279238));
#78137=CARTESIAN_POINT('Ctrl Pts',(3.47674120558153,140.464584533842,13.3278824813832));
#78138=CARTESIAN_POINT('Ctrl Pts',(3.47297848363,140.46443010861,13.2649486292002));
#78139=CARTESIAN_POINT('Ctrl Pts',(3.46229997926127,140.452577551596,13.0879354507405));
#78140=CARTESIAN_POINT('Ctrl Pts',(3.45540526651605,140.431531938995,12.9749198354831));
#78141=CARTESIAN_POINT('Ctrl Pts',(3.44766280692175,140.390852670363,12.8440782624796));
#78142=CARTESIAN_POINT('Ctrl Pts',(3.44641023310681,140.383698498533,12.8228057784297));
#78143=CARTESIAN_POINT('Ctrl Pts',(3.44439755376339,140.371262997021,12.7884647162484));
#78144=CARTESIAN_POINT('Ctrl Pts',(3.4436278935083,140.366277360269,12.7752936556342));
#78145=CARTESIAN_POINT('Ctrl Pts',(3.44214219432967,140.356205260591,12.7498026502038));
#78146=CARTESIAN_POINT('Ctrl Pts',(3.44142556662377,140.351139093871,12.7374762247398));
#78147=CARTESIAN_POINT('Ctrl Pts',(3.43973155704996,140.33867011977,12.7082788466883));
#78148=CARTESIAN_POINT('Ctrl Pts',(3.43875940668276,140.331115650545,12.6914749157925));
#78149=CARTESIAN_POINT('Ctrl Pts',(3.43523725161072,140.302305145296,12.630495311347));
#78150=CARTESIAN_POINT('Ctrl Pts',(3.43275185280457,140.279149989483,12.5872510200952));
#78151=CARTESIAN_POINT('Ctrl Pts',(3.42577804639236,140.206835073795,12.467114623918));
#78152=CARTESIAN_POINT('Ctrl Pts',(3.42143141091406,140.152605363204,12.3935511810349));
#78153=CARTESIAN_POINT('Ctrl Pts',(3.41437840618844,140.05720445989,12.2866573226237));
#78154=CARTESIAN_POINT('Ctrl Pts',(3.41176961318957,140.020479385239,12.2496831208837));
#78155=CARTESIAN_POINT('Ctrl Pts',(3.40835685791258,139.97229919986,12.2060928064908));
#78156=CARTESIAN_POINT('Ctrl Pts',(3.40767158892432,139.96261892614,12.1975647581915));
#78157=CARTESIAN_POINT('Ctrl Pts',(3.40655139896407,139.946818981303,12.1840122171201));
#78158=CARTESIAN_POINT('Ctrl Pts',(3.4061220620133,139.940768873303,12.1789073027083));
#78159=CARTESIAN_POINT('Ctrl Pts',(3.4052595336185,139.928634888969,12.1688363669593));
#78160=CARTESIAN_POINT('Ctrl Pts',(3.40482640688436,139.922551871954,12.1638697439615));
#78161=CARTESIAN_POINT('Ctrl Pts',(3.40368955868837,139.906602285339,12.1510598753505));
#78162=CARTESIAN_POINT('Ctrl Pts',(3.40298072234981,139.896674012335,12.1432948485353));
#78163=CARTESIAN_POINT('Ctrl Pts',(3.39941232385398,139.846701104864,12.1052404110541));
#78164=CARTESIAN_POINT('Ctrl Pts',(3.39644951353024,139.805219322734,12.0768997391778));
#78165=CARTESIAN_POINT('Ctrl Pts',(3.38860893858539,139.693293530767,12.0085959591534));
#78166=CARTESIAN_POINT('Ctrl Pts',(3.38368886121182,139.620838593996,11.9722422164872));
#78167=CARTESIAN_POINT('Ctrl Pts',(3.3754248025165,139.491336941169,11.9201959418631));
#78168=CARTESIAN_POINT('Ctrl Pts',(3.37202471328968,139.435654641086,11.9016161047724));
#78169=CARTESIAN_POINT('Ctrl Pts',(3.36762140413896,139.359927220255,11.8813123488158));
#78170=CARTESIAN_POINT('Ctrl Pts',(3.36652439028684,139.340750200544,11.8765845265348));
#78171=CARTESIAN_POINT('Ctrl Pts',(3.36476950223142,139.309576811633,11.8695653164109));
#78172=CARTESIAN_POINT('Ctrl Pts',(3.36410404781468,139.297637639231,11.8670334844503));
#78173=CARTESIAN_POINT('Ctrl Pts',(3.36271362796051,139.272448653474,11.8620202878826));
#78174=CARTESIAN_POINT('Ctrl Pts',(3.36198977215922,139.259193370751,11.8595720307994));
#78175=CARTESIAN_POINT('Ctrl Pts',(3.36024255922599,139.226867303336,11.8540620782963));
#78176=CARTESIAN_POINT('Ctrl Pts',(3.35922536853238,139.20776584591,11.8511940619226));
#78177=CARTESIAN_POINT('Ctrl Pts',(3.35522176623594,139.131561532493,11.8412904294161));
#78178=CARTESIAN_POINT('Ctrl Pts',(3.35232751344371,139.074120199961,11.837246053713));
#78179=CARTESIAN_POINT('Ctrl Pts',(3.3465261985009,138.956572231158,11.8359138209579));
#78180=CARTESIAN_POINT('Ctrl Pts',(3.3436294520061,138.896573086068,11.8389259736535));
#78181=CARTESIAN_POINT('Ctrl Pts',(3.33748065763914,138.771137308895,11.8529903141975));
#78182=CARTESIAN_POINT('Ctrl Pts',(3.33422941245165,138.705927835779,11.8648222421279));
#78183=CARTESIAN_POINT('Ctrl Pts',(3.32994244169614,138.625927337032,11.8850200725186));
#78184=CARTESIAN_POINT('Ctrl Pts',(3.32908333829389,138.6101736009,11.8892789475666));
#78185=CARTESIAN_POINT('Ctrl Pts',(3.32774357454516,138.586110586489,11.8962179841558));
#78186=CARTESIAN_POINT('Ctrl Pts',(3.32727282225491,138.577748154629,11.8987106772942));
#78187=CARTESIAN_POINT('Ctrl Pts',(3.32639180636825,138.562283055776,11.9034715492023));
#78188=CARTESIAN_POINT('Ctrl Pts',(3.32598266537213,138.555174690518,11.9057194426576));
#78189=CARTESIAN_POINT('Ctrl Pts',(3.32499671494542,138.538214984737,11.9112255361837));
#78190=CARTESIAN_POINT('Ctrl Pts',(3.32441711679906,138.528380690997,11.9145343287338));
#78191=CARTESIAN_POINT('Ctrl Pts',(3.32233104883395,138.493428383037,11.926709440084));
#78192=CARTESIAN_POINT('Ctrl Pts',(3.3207960514629,138.468519415094,11.9361561736659));
#78193=CARTESIAN_POINT('Ctrl Pts',(3.31666321124202,138.403146906964,11.9630115280814));
#78194=CARTESIAN_POINT('Ctrl Pts',(3.31402888426484,138.363188093868,11.9815759298846));
#78195=CARTESIAN_POINT('Ctrl Pts',(3.30428824606432,138.219539229737,12.0563691079987));
#78196=CARTESIAN_POINT('Ctrl Pts',(3.29717324240272,138.121895329679,12.1232767923625));
#78197=CARTESIAN_POINT('Ctrl Pts',(3.28922399737098,138.016320789655,12.2161545562617));
#78198=CARTESIAN_POINT('Ctrl Pts',(3.28795864243356,137.99965654557,12.2315156581374));
#78199=CARTESIAN_POINT('Ctrl Pts',(3.28593086056927,137.97319355856,12.2570712706267));
#78200=CARTESIAN_POINT('Ctrl Pts',(3.28515860727105,137.96317442958,12.267031191698));
#78201=CARTESIAN_POINT('Ctrl Pts',(3.28367135472077,137.944001781126,12.2866505870111));
#78202=CARTESIAN_POINT('Ctrl Pts',(3.28295570885517,137.934832735968,12.2962928779888));
#78203=CARTESIAN_POINT('Ctrl Pts',(3.2812694640749,137.913374323431,12.3194841031224));
#78204=CARTESIAN_POINT('Ctrl Pts',(3.28030396148403,137.901204826964,12.3331411725082));
#78205=CARTESIAN_POINT('Ctrl Pts',(3.27684504717546,137.858092776139,12.3833887823832));
#78206=CARTESIAN_POINT('Ctrl Pts',(3.27441303928814,137.828694673803,12.4212664700008));
#78207=CARTESIAN_POINT('Ctrl Pts',(3.26770454816095,137.751409950639,12.5316306916283));
#78208=CARTESIAN_POINT('Ctrl Pts',(3.26355480582356,137.708040678928,12.6070284516602));
#78209=CARTESIAN_POINT('Ctrl Pts',(3.25648070783177,137.64750350872,12.7379635532396));
#78210=CARTESIAN_POINT('Ctrl Pts',(3.25361929884706,137.626490253744,12.7914712264083));
#78211=CARTESIAN_POINT('Ctrl Pts',(3.2499158729755,137.604604409594,12.8585525973906));
#78212=CARTESIAN_POINT('Ctrl Pts',(3.24921884122643,137.600700039935,12.8710894488228));
#78213=CARTESIAN_POINT('Ctrl Pts',(3.24808413696821,137.594699195873,12.8913126600479));
#78214=CARTESIAN_POINT('Ctrl Pts',(3.24765231510458,137.592495801843,12.8989668118558));
#78215=CARTESIAN_POINT('Ctrl Pts',(3.24678981132717,137.588256064853,12.9141602714618));
#78216=CARTESIAN_POINT('Ctrl Pts',(3.24635926947857,137.586217383655,12.9216986110282));
#78217=CARTESIAN_POINT('Ctrl Pts',(3.24523697857455,137.581099390025,12.9412425278066));
#78218=CARTESIAN_POINT('Ctrl Pts',(3.24454034137454,137.578112133274,12.9532713765573));
#78219=CARTESIAN_POINT('Ctrl Pts',(3.24117591250513,137.564560552932,13.0109628221969));
#78220=CARTESIAN_POINT('Ctrl Pts',(3.23841806440327,137.556041782866,13.0570743846208));
#78221=CARTESIAN_POINT('Ctrl Pts',(3.23172620786661,137.540985892648,13.1681991539778));
#78222=CARTESIAN_POINT('Ctrl Pts',(3.22776565882116,137.536559451577,13.2334009106179));
#78223=CARTESIAN_POINT('Ctrl Pts',(3.22385963331144,137.53650059484,13.2986804940338));
#78224=CARTESIAN_POINT('Ctrl Pts',(3.22393332744186,137.536628644961,13.2986850195007));
#78225=CARTESIAN_POINT('Ctrl Pts',(3.22390770808568,137.536629296413,13.2991232392521));
#78226=CARTESIAN_POINT('Ctrl Pts',(3.22388209050693,137.536630143947,13.2995614623613));
#78227=CARTESIAN_POINT('Ctrl Pts',(3.22385647472349,137.536631187551,13.2999996886484));
#78228=CARTESIAN_POINT('',(3.65155456155019,137.536499869567,13.3004052814541));
#78229=CARTESIAN_POINT('Ctrl Pts',(3.1529262221125,137.5365,13.3000000000405));
#78230=CARTESIAN_POINT('Ctrl Pts',(3.15294755840493,137.5365,13.2995616236816));
#78231=CARTESIAN_POINT('Ctrl Pts',(3.15296889379876,137.536500196966,13.2991232433111));
#78232=CARTESIAN_POINT('Ctrl Pts',(3.15751033426512,137.536584055109,13.2058052336659));
#78233=CARTESIAN_POINT('Ctrl Pts',(3.16195982162168,137.545509033665,13.1131535443846));
#78234=CARTESIAN_POINT('Ctrl Pts',(3.16771026279101,137.56663405572,13.0039751141562));
#78235=CARTESIAN_POINT('Ctrl Pts',(3.16867234969529,137.570456420978,12.9860354171264));
#78236=CARTESIAN_POINT('Ctrl Pts',(3.17013174161221,137.576652671786,12.9594189949979));
#78237=CARTESIAN_POINT('Ctrl Pts',(3.1706158604517,137.578771162034,12.9506840693296));
#78238=CARTESIAN_POINT('Ctrl Pts',(3.17150088843002,137.582753232004,12.9349014023963));
#78239=CARTESIAN_POINT('Ctrl Pts',(3.17190027439989,137.584589207954,12.9278472484509));
#78240=CARTESIAN_POINT('Ctrl Pts',(3.1728420867,137.589009672106,12.9113690287514));
#78241=CARTESIAN_POINT('Ctrl Pts',(3.17338677568636,137.591635926829,12.9019568317226));
#78242=CARTESIAN_POINT('Ctrl Pts',(3.17522105621282,137.600718501482,12.8706215717162));
#78243=CARTESIAN_POINT('Ctrl Pts',(3.17653130032495,137.607593797145,12.8488244244251));
#78244=CARTESIAN_POINT('Ctrl Pts',(3.17989083960996,137.626263723224,12.794132787799));
#78245=CARTESIAN_POINT('Ctrl Pts',(3.18196326855966,137.638731205648,12.7614834938888));
#78246=CARTESIAN_POINT('Ctrl Pts',(3.18854188070924,137.681603102232,12.6602438283886));
#78247=CARTESIAN_POINT('Ctrl Pts',(3.19309763093147,137.71611998596,12.5935220360881));
#78248=CARTESIAN_POINT('Ctrl Pts',(3.20125385796455,137.788412655287,12.4767289300527));
#78249=CARTESIAN_POINT('Ctrl Pts',(3.20487897271493,137.824582211789,12.4258640488924));
#78250=CARTESIAN_POINT('Ctrl Pts',(3.20951444539336,137.87656148433,12.3618517018039));
#78251=CARTESIAN_POINT('Ctrl Pts',(3.21063194066752,137.889553518242,12.3465090479064));
#78252=CARTESIAN_POINT('Ctrl Pts',(3.21240752262372,137.910937850465,12.3222858613872));
#78253=CARTESIAN_POINT('Ctrl Pts',(3.21307362791868,137.919132088415,12.3132346414778));
#78254=CARTESIAN_POINT('Ctrl Pts',(3.21445632491872,137.936498631168,12.2945277686582));
#78255=CARTESIAN_POINT('Ctrl Pts',(3.21517195098565,137.94569142272,12.2848926118549));
#78256=CARTESIAN_POINT('Ctrl Pts',(3.21688159878464,137.968138656341,12.2619991267902));
#78257=CARTESIAN_POINT('Ctrl Pts',(3.21787000150962,137.981518981748,12.248867228555));
#78258=CARTESIAN_POINT('Ctrl Pts',(3.22158792416261,138.033328705337,12.1999378372203));
#78259=CARTESIAN_POINT('Ctrl Pts',(3.22424204467757,138.073424029924,12.1659595159793));
#78260=CARTESIAN_POINT('Ctrl Pts',(3.23221073876424,138.201485255124,12.0687718558));
#78261=CARTESIAN_POINT('Ctrl Pts',(3.23731520016404,138.294694732578,12.0131082029346));
#78262=CARTESIAN_POINT('Ctrl Pts',(3.2444334374589,138.423674767298,11.9543387272715));
#78263=CARTESIAN_POINT('Ctrl Pts',(3.24614808605334,138.454632837018,11.9414973703536));
#78264=CARTESIAN_POINT('Ctrl Pts',(3.24852371530324,138.496767966907,11.9256921801478));
#78265=CARTESIAN_POINT('Ctrl Pts',(3.24913699095929,138.507580743555,11.9217809600122));
#78266=CARTESIAN_POINT('Ctrl Pts',(3.25016344770839,138.525542382742,11.9155221858991));
#78267=CARTESIAN_POINT('Ctrl Pts',(3.25057250969724,138.532665520309,11.9131015427845));
#78268=CARTESIAN_POINT('Ctrl Pts',(3.25142967204679,138.547509735395,11.9081844040243));
#78269=CARTESIAN_POINT('Ctrl Pts',(3.25187823324844,138.555233390326,11.9056970382251));
#78270=CARTESIAN_POINT('Ctrl Pts',(3.25310913027287,138.576321240534,11.8990988412559));
#78271=CARTESIAN_POINT('Ctrl Pts',(3.25389818135018,138.589724001539,11.895115192073));
#78272=CARTESIAN_POINT('Ctrl Pts',(3.25881460932111,138.672681873001,11.8717462657293));
#78273=CARTESIAN_POINT('Ctrl Pts',(3.26314868270188,138.743530769368,11.857340036066));
#78274=CARTESIAN_POINT('Ctrl Pts',(3.27398278108366,138.921962374414,11.8346205421573));
#78275=CARTESIAN_POINT('Ctrl Pts',(3.28044530560699,139.029969325974,11.8328479289741));
#78276=CARTESIAN_POINT('Ctrl Pts',(3.28786047488858,139.160385303115,11.845128538219));
#78277=CARTESIAN_POINT('Ctrl Pts',(3.28916206025021,139.183512669676,11.8478644679518));
#78278=CARTESIAN_POINT('Ctrl Pts',(3.2912294450728,139.22061727807,11.8531545619147));
#78279=CARTESIAN_POINT('Ctrl Pts',(3.29200590715503,139.234639116481,11.8553622564576));
#78280=CARTESIAN_POINT('Ctrl Pts',(3.29348968891621,139.261591534641,11.8600086132795));
#78281=CARTESIAN_POINT('Ctrl Pts',(3.29419784328166,139.274525642452,11.8624183459632));
#78282=CARTESIAN_POINT('Ctrl Pts',(3.29584839371893,139.304825110353,11.868487239466));
#78283=CARTESIAN_POINT('Ctrl Pts',(3.29678619325137,139.322160066447,11.8722885237703));
#78284=CARTESIAN_POINT('Ctrl Pts',(3.3000236405971,139.382352909126,11.8866400574855));
#78285=CARTESIAN_POINT('Ctrl Pts',(3.30227214938022,139.424800710582,11.8988130468265));
#78286=CARTESIAN_POINT('Ctrl Pts',(3.30817797019884,139.536752369269,11.9364744913971));
#78287=CARTESIAN_POINT('Ctrl Pts',(3.31174719840716,139.60498112864,11.965345289833));
#78288=CARTESIAN_POINT('Ctrl Pts',(3.31873543755969,139.732592082261,12.0311482059054));
#78289=CARTESIAN_POINT('Ctrl Pts',(3.32214415839357,139.792090269984,12.0674143853622));
#78290=CARTESIAN_POINT('Ctrl Pts',(3.32660042568913,139.861929989689,12.1171349916392));
#78291=CARTESIAN_POINT('Ctrl Pts',(3.32745072213696,139.874926613928,12.1267155871335));
#78292=CARTESIAN_POINT('Ctrl Pts',(3.32877785151568,139.894644718368,12.1417608022986));
#78293=CARTESIAN_POINT('Ctrl Pts',(3.32924499701,139.901480974738,12.1470736121598));
#78294=CARTESIAN_POINT('Ctrl Pts',(3.33011984666183,139.914079307095,12.1570449838738));
#78295=CARTESIAN_POINT('Ctrl Pts',(3.33052645503831,139.919853739121,12.1616871086149));
#78296=CARTESIAN_POINT('Ctrl Pts',(3.33150656011536,139.933584173416,12.1728978383743));
#78297=CARTESIAN_POINT('Ctrl Pts',(3.3320828185508,139.941506309057,12.1795070062589));
#78298=CARTESIAN_POINT('Ctrl Pts',(3.33415677366883,139.969514341964,12.2033798929647));
#78299=CARTESIAN_POINT('Ctrl Pts',(3.33568270399178,139.989199755064,12.2211036216512));
#78300=CARTESIAN_POINT('Ctrl Pts',(3.33978701302044,140.040078104931,12.2694752410841));
#78301=CARTESIAN_POINT('Ctrl Pts',(3.34240146224568,140.070396729978,12.3010033881348));
#78302=CARTESIAN_POINT('Ctrl Pts',(3.35202624990321,140.176056050839,12.4212181711514));
#78303=CARTESIAN_POINT('Ctrl Pts',(3.35904978909633,140.242175864504,12.5174576917622));
#78304=CARTESIAN_POINT('Ctrl Pts',(3.36698869559953,140.307228898286,12.6415557244939));
#78305=CARTESIAN_POINT('Ctrl Pts',(3.36831720314937,140.31774186761,12.6628558093501));
#78306=CARTESIAN_POINT('Ctrl Pts',(3.3704163674997,140.333741851227,12.697364915776));
#78307=CARTESIAN_POINT('Ctrl Pts',(3.37119828437813,140.339561486373,12.7104142004422));
#78308=CARTESIAN_POINT('Ctrl Pts',(3.37268596212271,140.350358499503,12.7356097059127));
#78309=CARTESIAN_POINT('Ctrl Pts',(3.37339266964003,140.355365365852,12.7477417073982));
#78310=CARTESIAN_POINT('Ctrl Pts',(3.37503016978599,140.366673694673,12.7762231282036));
#78311=CARTESIAN_POINT('Ctrl Pts',(3.37595659084267,140.372846157504,12.7926217762155));
#78312=CARTESIAN_POINT('Ctrl Pts',(3.37909766204547,140.392970177589,12.8491445248979));
#78313=CARTESIAN_POINT('Ctrl Pts',(3.38126540331281,140.405469221385,12.8897643997763));
#78314=CARTESIAN_POINT('Ctrl Pts',(3.38685258971738,140.433598868699,12.9976859685849));
#78315=CARTESIAN_POINT('Ctrl Pts',(3.3901968497738,140.44626410632,13.0656495535306));
#78316=CARTESIAN_POINT('Ctrl Pts',(3.3973092414232,140.462834893467,13.2110246708388));
#78317=CARTESIAN_POINT('Ctrl Pts',(3.40107005123646,140.465491309069,13.2883605521666));
#78318=CARTESIAN_POINT('Ctrl Pts',(3.40591345538974,140.461322203631,13.3813685678251));
#78319=CARTESIAN_POINT('Ctrl Pts',(3.40674865438157,140.460355393055,13.3971880281685));
#78320=CARTESIAN_POINT('Ctrl Pts',(3.40805704392904,140.458468331259,13.4215576200612));
#78321=CARTESIAN_POINT('Ctrl Pts',(3.40852096604346,140.457729278714,13.430120985265));
#78322=CARTESIAN_POINT('Ctrl Pts',(3.40939343889964,140.456211406476,13.4460674551689));
#78323=CARTESIAN_POINT('Ctrl Pts',(3.40980096622735,140.455451776379,13.4534518807826));
#78324=CARTESIAN_POINT('Ctrl Pts',(3.4107883893904,140.453489871171,13.4711964359356));
#78325=CARTESIAN_POINT('Ctrl Pts',(3.41137116125793,140.452232979571,13.4815499527864));
#78326=CARTESIAN_POINT('Ctrl Pts',(3.41349816954794,140.44728650236,13.5189501144346));
#78327=CARTESIAN_POINT('Ctrl Pts',(3.41507248036451,140.442951222455,13.5459043723841));
#78328=CARTESIAN_POINT('Ctrl Pts',(3.41935454315111,140.429318300634,13.6177814266914));
#78329=CARTESIAN_POINT('Ctrl Pts',(3.42210180326305,140.418658280452,13.662414327594));
#78330=CARTESIAN_POINT('Ctrl Pts',(3.43185250710553,140.373656736234,13.8180678584859));
#78331=CARTESIAN_POINT('Ctrl Pts',(3.43884921043368,140.328214020917,13.9254461577063));
#78332=CARTESIAN_POINT('Ctrl Pts',(3.44666339893655,140.259544985473,14.0455667357442));
#78333=CARTESIAN_POINT('Ctrl Pts',(3.44789987761416,140.248111009153,14.0645536687447));
#78334=CARTESIAN_POINT('Ctrl Pts',(3.44989032871341,140.228774399358,14.0950728334207));
#78335=CARTESIAN_POINT('Ctrl Pts',(3.45065356862008,140.221130330747,14.1067639489332));
#78336=CARTESIAN_POINT('Ctrl Pts',(3.45212895722999,140.205908614946,14.1293324619642));
#78337=CARTESIAN_POINT('Ctrl Pts',(3.452841654362,140.198348264316,14.1402198363276));
#78338=CARTESIAN_POINT('Ctrl Pts',(3.45452930732891,140.179955506056,14.165953192439));
#78339=CARTESIAN_POINT('Ctrl Pts',(3.45549902623404,140.168989213932,14.180700962625));
#78340=CARTESIAN_POINT('Ctrl Pts',(3.45902820676924,140.127651733932,14.2341597458875));
#78341=CARTESIAN_POINT('Ctrl Pts',(3.46152244505263,140.095610810504,14.2715402235041));
#78342=CARTESIAN_POINT('Ctrl Pts',(3.46854943384063,139.998355457973,14.3740586089793));
#78343=CARTESIAN_POINT('Ctrl Pts',(3.47293690423006,139.928801403468,14.4347436011896));
#78344=CARTESIAN_POINT('Ctrl Pts',(3.47999270329075,139.812495117348,14.5183172232605));
#78345=CARTESIAN_POINT('Ctrl Pts',(3.48255588311855,139.769452979622,14.5459479914702));
#78346=CARTESIAN_POINT('Ctrl Pts',(3.48591455762878,139.713920052445,14.5776207636146));
#78347=CARTESIAN_POINT('Ctrl Pts',(3.48659574462048,139.702699495468,14.5838263331335));
#78348=CARTESIAN_POINT('Ctrl Pts',(3.48770917764604,139.684464793677,14.5936004401251));
#78349=CARTESIAN_POINT('Ctrl Pts',(3.48813590575812,139.677500651613,14.5972613513293));
#78350=CARTESIAN_POINT('Ctrl Pts',(3.48899273800856,139.663576309529,14.6044383986713));
#78351=CARTESIAN_POINT('Ctrl Pts',(3.48942277230695,139.656616865855,14.6079554042241));
#78352=CARTESIAN_POINT('Ctrl Pts',(3.49055016368183,139.638435968646,14.6169615841983));
#78353=CARTESIAN_POINT('Ctrl Pts',(3.49125253775838,139.627171939625,14.62236289914));
#78354=CARTESIAN_POINT('Ctrl Pts',(3.49475168624053,139.571280992994,14.6482889416698));
#78355=CARTESIAN_POINT('Ctrl Pts',(3.49764744150161,139.525712507597,14.6667006298247));
#78356=CARTESIAN_POINT('Ctrl Pts',(3.50412935346481,139.423223342205,14.7022260142005));
#78357=CARTESIAN_POINT('Ctrl Pts',(3.50772643042839,139.366007044435,14.7182364696718));
#78358=CARTESIAN_POINT('Ctrl Pts',(3.51602394684218,139.230628240194,14.747377914374));
#78359=CARTESIAN_POINT('Ctrl Pts',(3.52067440013414,139.152049223164,14.7577297911334));
#78360=CARTESIAN_POINT('Ctrl Pts',(3.52630171018029,139.052234413982,14.7627154535567));
#78361=CARTESIAN_POINT('Ctrl Pts',(3.52745959228154,139.031438842244,14.7633101496295));
#78362=CARTESIAN_POINT('Ctrl Pts',(3.52935718492527,138.996939522364,14.7635609009486));
#78363=CARTESIAN_POINT('Ctrl Pts',(3.53010457018412,138.983241139322,14.7634681533269));
#78364=CARTESIAN_POINT('Ctrl Pts',(3.53157259041123,138.956124311386,14.7629037516989));
#78365=CARTESIAN_POINT('Ctrl Pts',(3.53229339027029,138.942707070637,14.7624397421706));
#78366=CARTESIAN_POINT('Ctrl Pts',(3.53403977574091,138.909963086359,14.76085601952));
#78367=CARTESIAN_POINT('Ctrl Pts',(3.53505909665065,138.89064827656,14.7595373248535));
#78368=CARTESIAN_POINT('Ctrl Pts',(3.53912955012471,138.81280590453,14.7526687337649));
#78369=CARTESIAN_POINT('Ctrl Pts',(3.54208391120584,138.754608863449,14.7439779009135));
#78370=CARTESIAN_POINT('Ctrl Pts',(3.54790020566391,138.639192295387,14.7195604892136));
#78371=CARTESIAN_POINT('Ctrl Pts',(3.55075626980304,138.582092090765,14.703811692831));
#78372=CARTESIAN_POINT('Ctrl Pts',(3.55684165504907,138.463924695934,14.6633687868989));
#78373=CARTESIAN_POINT('Ctrl Pts',(3.56007080357649,138.403256085178,14.6379261480481));
#78374=CARTESIAN_POINT('Ctrl Pts',(3.56432930608584,138.32998821099,14.6012225752537));
#78375=CARTESIAN_POINT('Ctrl Pts',(3.56518438860922,138.315590892404,14.5937078954065));
#78376=CARTESIAN_POINT('Ctrl Pts',(3.56651745580689,138.293697128591,14.5818127040727));
#78377=CARTESIAN_POINT('Ctrl Pts',(3.56698561851442,138.286109253497,14.5776022655315));
#78378=CARTESIAN_POINT('Ctrl Pts',(3.56786123990405,138.272116536529,14.5696742694914));
#78379=CARTESIAN_POINT('Ctrl Pts',(3.56826758017445,138.265701804731,14.5659752126448));
#78380=CARTESIAN_POINT('Ctrl Pts',(3.56924547442094,138.250446800748,14.5570234642089));
#78381=CARTESIAN_POINT('Ctrl Pts',(3.56981975541381,138.241633439664,14.5517260625964));
#78382=CARTESIAN_POINT('Ctrl Pts',(3.57187786619908,138.210527683784,14.5325803935952));
#78383=CARTESIAN_POINT('Ctrl Pts',(3.57338939136101,138.188553802301,14.5182265262404));
#78384=CARTESIAN_POINT('Ctrl Pts',(3.57744159269108,138.131545850945,14.4787607341075));
#78385=CARTESIAN_POINT('Ctrl Pts',(3.58001735579869,138.097215016411,14.4526787954019));
#78386=CARTESIAN_POINT('Ctrl Pts',(3.58944410734881,137.976674460903,14.3524091847949));
#78387=CARTESIAN_POINT('Ctrl Pts',(3.59631549599301,137.898019289369,14.2697453113168));
#78388=CARTESIAN_POINT('Ctrl Pts',(3.60422893629836,137.814465641131,14.1584790690359));
#78389=CARTESIAN_POINT('Ctrl Pts',(3.60565486151238,137.799737438369,14.1377636447471));
#78390=CARTESIAN_POINT('Ctrl Pts',(3.60787672680222,137.77731981009,14.1044272606911));
#78391=CARTESIAN_POINT('Ctrl Pts',(3.60868602987274,137.76926965336,14.0920561222972));
#78392=CARTESIAN_POINT('Ctrl Pts',(3.61019600340686,137.754474604263,14.0685493813113));
#78393=CARTESIAN_POINT('Ctrl Pts',(3.61089814679496,137.747688532325,14.0574415264562));
#78394=CARTESIAN_POINT('Ctrl Pts',(3.61248418145654,137.732581638437,14.0319555007784));
#78395=CARTESIAN_POINT('Ctrl Pts',(3.61336459819105,137.724355546632,14.0175231125313));
#78396=CARTESIAN_POINT('Ctrl Pts',(3.61614751055924,137.698895057913,13.9710311595773));
#78397=CARTESIAN_POINT('Ctrl Pts',(3.61801706801827,137.682609534172,13.9384665353132));
#78398=CARTESIAN_POINT('Ctrl Pts',(3.62255867782303,137.645405641842,13.8565732978988));
#78399=CARTESIAN_POINT('Ctrl Pts',(3.62518925385113,137.625948730523,13.8066391913907));
#78400=CARTESIAN_POINT('Ctrl Pts',(3.63071422561598,137.590639235391,13.6988915293272));
#78401=CARTESIAN_POINT('Ctrl Pts',(3.63359797507643,137.575511475382,13.6409462229351));
#78402=CARTESIAN_POINT('Ctrl Pts',(3.63890633058407,137.554795195006,13.5355422872998));
#78403=CARTESIAN_POINT('Ctrl Pts',(3.64130180439216,137.547901220175,13.4884290088702));
#78404=CARTESIAN_POINT('Ctrl Pts',(3.64446671289217,137.542098559195,13.4285099980814));
#78405=CARTESIAN_POINT('Ctrl Pts',(3.64513737310426,137.541044909464,13.4159372811191));
#78406=CARTESIAN_POINT('Ctrl Pts',(3.64623782630549,137.539601435773,13.3955484146922));
#78407=CARTESIAN_POINT('Ctrl Pts',(3.64666233494489,137.539111505068,13.3877397611939));
#78408=CARTESIAN_POINT('Ctrl Pts',(3.64746287321699,137.538312433838,13.3731303719459));
#78409=CARTESIAN_POINT('Ctrl Pts',(3.64783802623788,137.537988086607,13.3663306384269));
#78410=CARTESIAN_POINT('Ctrl Pts',(3.64870338654884,137.537353593872,13.3507447710495));
#78411=CARTESIAN_POINT('Ctrl Pts',(3.6491952381005,137.537075160363,13.341957681216));
#78412=CARTESIAN_POINT('Ctrl Pts',(3.65030652276399,137.53662836591,13.3222489504325));
#78413=CARTESIAN_POINT('Ctrl Pts',(3.65092794022738,137.53650307742,13.3113269345325));
#78414=CARTESIAN_POINT('Ctrl Pts',(3.65155426291434,137.536500055998,13.3004048542518));
#78415=CARTESIAN_POINT('Ctrl Pts',(3.65155423947869,137.536500056111,13.3004052629325));
#78416=CARTESIAN_POINT('Ctrl Pts',(3.65156198605023,137.536500018704,13.3002701749106));
#78417=CARTESIAN_POINT('Ctrl Pts',(3.65156973335021,137.5365,13.3001350872663));
#78418=CARTESIAN_POINT('Ctrl Pts',(3.65157748137715,137.5365,13.3000000000035));
#78419=CARTESIAN_POINT('Origin',(4.2,139.,13.3));
#78420=CARTESIAN_POINT('',(4.22337996970852,137.5365,13.299999999996));
#78421=CARTESIAN_POINT('',(4.15384019369498,137.5365,13.3000000000084));
#78422=CARTESIAN_POINT('',(4.2,137.5365,13.3));
#78423=CARTESIAN_POINT('',(4.22332920524334,137.536500478426,13.3010219306143));
#78424=CARTESIAN_POINT('Ctrl Pts',(4.22337996970853,137.5365,13.299999999996));
#78425=CARTESIAN_POINT('Ctrl Pts',(4.22336296862726,137.5365,13.3003407816243));
#78426=CARTESIAN_POINT('Ctrl Pts',(4.22334596990515,137.536500119028,13.3006815642919));
#78427=CARTESIAN_POINT('Ctrl Pts',(4.22332897353037,137.536500357088,13.3010223479367));
#78428=CARTESIAN_POINT('Ctrl Pts',(4.22332899486318,137.536500356789,13.301021920206));
#78429=CARTESIAN_POINT('Ctrl Pts',(4.21832396167272,137.536570430274,13.4013746880209));
#78430=CARTESIAN_POINT('Ctrl Pts',(4.21356247497565,137.546961721373,13.501450363291));
#78431=CARTESIAN_POINT('Ctrl Pts',(4.20625949287419,137.577206410225,13.6460245454743));
#78432=CARTESIAN_POINT('Ctrl Pts',(4.2038741173552,137.589145841286,13.6918729294185));
#78433=CARTESIAN_POINT('Ctrl Pts',(4.2007293433516,137.60699605147,13.7489172127474));
#78434=CARTESIAN_POINT('Ctrl Pts',(4.20006838602579,137.610857816477,13.7607283776677));
#78435=CARTESIAN_POINT('Ctrl Pts',(4.19897812123783,137.617392718495,13.7798858643397));
#78436=CARTESIAN_POINT('Ctrl Pts',(4.19855385804683,137.619975227322,13.7872627217991));
#78437=CARTESIAN_POINT('Ctrl Pts',(4.19769045099725,137.625305975751,13.8021074667226));
#78438=CARTESIAN_POINT('Ctrl Pts',(4.19725121228529,137.628056266367,13.8095742870747));
#78439=CARTESIAN_POINT('Ctrl Pts',(4.19608030268081,137.635493099844,13.829268011228));
#78440=CARTESIAN_POINT('Ctrl Pts',(4.19534297447281,137.640282990253,13.8414548339741));
#78441=CARTESIAN_POINT('Ctrl Pts',(4.19138793972816,137.666576951624,13.9058040261453));
#78442=CARTESIAN_POINT('Ctrl Pts',(4.18804105151076,137.69091907293,13.9567507941404));
#78443=CARTESIAN_POINT('Ctrl Pts',(4.17940095242827,137.76041668487,14.0829066702024));
#78444=CARTESIAN_POINT('Ctrl Pts',(4.17408198891199,137.809505506131,14.1557070053943));
#78445=CARTESIAN_POINT('Ctrl Pts',(4.16612309618769,137.895189353068,14.2610108926096));
#78446=CARTESIAN_POINT('Ctrl Pts',(4.16335798259313,137.927389710947,14.2968231491989));
#78447=CARTESIAN_POINT('Ctrl Pts',(4.1596396389996,137.974202017753,14.3439857365848));
#78448=CARTESIAN_POINT('Ctrl Pts',(4.15862527155178,137.987348162386,14.3567421716348));
#78449=CARTESIAN_POINT('Ctrl Pts',(4.15689225499151,138.010454426051,14.3783361887832));
#78450=CARTESIAN_POINT('Ctrl Pts',(4.15616865455337,138.020301830803,14.387290620119));
#78451=CARTESIAN_POINT('Ctrl Pts',(4.15468909695458,138.040843800061,14.4054641286139));
#78452=CARTESIAN_POINT('Ctrl Pts',(4.15393392318336,138.051552393547,14.4146652916057));
#78453=CARTESIAN_POINT('Ctrl Pts',(4.15198504780083,138.079758321728,14.4381999019641));
#78454=CARTESIAN_POINT('Ctrl Pts',(4.15080132032213,138.097458037034,14.4522854856909));
#78455=CARTESIAN_POINT('Ctrl Pts',(4.14377563488128,138.205732327792,14.5344249849649));
#78456=CARTESIAN_POINT('Ctrl Pts',(4.13834519302298,138.303629111033,14.5921824183654));
#78457=CARTESIAN_POINT('Ctrl Pts',(4.1305203277536,138.45036357004,14.6571880495186));
#78458=CARTESIAN_POINT('Ctrl Pts',(4.1282020268816,138.494410984787,14.6742048249214));
#78459=CARTESIAN_POINT('Ctrl Pts',(4.12439821662107,138.565602302351,14.6978213880667));
#78460=CARTESIAN_POINT('Ctrl Pts',(4.12296217820215,138.592246537744,14.7058246416548));
#78461=CARTESIAN_POINT('Ctrl Pts',(4.12092944040672,138.629275923906,14.7158061173772));
#78462=CARTESIAN_POINT('Ctrl Pts',(4.12036546485904,138.639479927177,14.7184387779075));
#78463=CARTESIAN_POINT('Ctrl Pts',(4.11939088860207,138.656970193759,14.72275039893));
#78464=CARTESIAN_POINT('Ctrl Pts',(4.1189833285372,138.664242387833,14.7244841066348));
#78465=CARTESIAN_POINT('Ctrl Pts',(4.11809792430773,138.679943585532,14.7281003894961));
#78466=CARTESIAN_POINT('Ctrl Pts',(4.1176191396927,138.688376058465,14.7299641052484));
#78467=CARTESIAN_POINT('Ctrl Pts',(4.11624842282245,138.712371431767,14.7350451587972));
#78468=CARTESIAN_POINT('Ctrl Pts',(4.11534747507424,138.727970516207,14.7380836969089));
#78469=CARTESIAN_POINT('Ctrl Pts',(4.11000067197004,138.819758727907,14.7544162823216));
#78470=CARTESIAN_POINT('Ctrl Pts',(4.10533361085638,138.896851199879,14.7619070972357));
#78471=CARTESIAN_POINT('Ctrl Pts',(4.0965249698177,139.043044489215,14.7644879103771));
#78472=CARTESIAN_POINT('Ctrl Pts',(4.09239212990641,139.111925392132,14.7608393751406));
#78473=CARTESIAN_POINT('Ctrl Pts',(4.08590382078877,139.22243486444,14.7471205691818));
#78474=CARTESIAN_POINT('Ctrl Pts',(4.08347646765041,139.264327656169,14.7400578479565));
#78475=CARTESIAN_POINT('Ctrl Pts',(4.08012324827709,139.323050790133,14.727508165028));
#78476=CARTESIAN_POINT('Ctrl Pts',(4.0791511836517,139.340177354777,14.7235240705886));
#78477=CARTESIAN_POINT('Ctrl Pts',(4.07746656338379,139.370029072654,14.7160102297428));
#78478=CARTESIAN_POINT('Ctrl Pts',(4.07674979555009,139.382785732073,14.7126151579989));
#78479=CARTESIAN_POINT('Ctrl Pts',(4.07526250813431,139.40936197078,14.7051556741769));
#78480=CARTESIAN_POINT('Ctrl Pts',(4.07449312496803,139.423171032005,14.7010588815359));
#78481=CARTESIAN_POINT('Ctrl Pts',(4.07245696156446,139.459856487304,14.6895833675664));
#78482=CARTESIAN_POINT('Ctrl Pts',(4.07120197561785,139.482615791233,14.6818436988438));
#78483=CARTESIAN_POINT('Ctrl Pts',(4.06375892309784,139.618147055573,14.6319968227625));
#78484=CARTESIAN_POINT('Ctrl Pts',(4.05803570713088,139.725556964742,14.5766711369999));
#78485=CARTESIAN_POINT('Ctrl Pts',(4.0494252812342,139.870779407724,14.4775608976839));
#78486=CARTESIAN_POINT('Ctrl Pts',(4.04667198732655,139.91475926861,14.443731140496));
#78487=CARTESIAN_POINT('Ctrl Pts',(4.04297409797902,139.968474658797,14.3973289233344));
#78488=CARTESIAN_POINT('Ctrl Pts',(4.04215378873461,139.980075894789,14.3869798219101));
#78489=CARTESIAN_POINT('Ctrl Pts',(4.04086684303432,139.997740827494,14.3707087659492));
#78490=CARTESIAN_POINT('Ctrl Pts',(4.04040914065602,140.003921935408,14.3649153772748));
#78491=CARTESIAN_POINT('Ctrl Pts',(4.03953710197643,140.015497933818,14.3538751472433));
#78492=CARTESIAN_POINT('Ctrl Pts',(4.03912358710051,140.020903183948,14.3486398615032));
#78493=CARTESIAN_POINT('Ctrl Pts',(4.03810502958813,140.03401866212,14.3357392816082));
#78494=CARTESIAN_POINT('Ctrl Pts',(4.03749669052269,140.041684220147,14.3280293886896));
#78495=CARTESIAN_POINT('Ctrl Pts',(4.03528762660687,140.068953893885,14.2999838342035));
#78496=CARTESIAN_POINT('Ctrl Pts',(4.03365521910621,140.088053277994,14.2791679953743));
#78497=CARTESIAN_POINT('Ctrl Pts',(4.02533018537058,140.180955193076,14.1718408670755));
#78498=CARTESIAN_POINT('Ctrl Pts',(4.0183368030541,140.245101376927,14.0774874229262));
#78499=CARTESIAN_POINT('Ctrl Pts',(4.00848636368444,140.322393842191,13.9292567472796));
#78500=CARTESIAN_POINT('Ctrl Pts',(4.00540179150499,140.344494810375,13.88053785794));
#78501=CARTESIAN_POINT('Ctrl Pts',(4.0013455241145,140.370740453831,13.8130892129656));
#78502=CARTESIAN_POINT('Ctrl Pts',(4.00029674931193,140.377256677992,13.7953322343927));
#78503=CARTESIAN_POINT('Ctrl Pts',(3.99852387552302,140.387801391026,13.7647787938723));
#78504=CARTESIAN_POINT('Ctrl Pts',(3.99779420961181,140.39200138224,13.752044463254));
#78505=CARTESIAN_POINT('Ctrl Pts',(3.99640730556487,140.399711145863,13.7275414835868));
#78506=CARTESIAN_POINT('Ctrl Pts',(3.99574920202892,140.403248941935,13.7157829139579));
#78507=CARTESIAN_POINT('Ctrl Pts',(3.99402140463634,140.412211674865,13.6845751947648));
#78508=CARTESIAN_POINT('Ctrl Pts',(3.99295993035147,140.417382925553,13.6650555982226));
#78509=CARTESIAN_POINT('Ctrl Pts',(3.98864700581961,140.43696556345,13.5844341850033));
#78510=CARTESIAN_POINT('Ctrl Pts',(3.98550628881357,140.447843135909,13.522540179273));
#78511=CARTESIAN_POINT('Ctrl Pts',(3.97875172484933,140.462886796984,13.3858789997987));
#78512=CARTESIAN_POINT('Ctrl Pts',(3.97517243221057,140.465363170715,13.3111083327715));
#78513=CARTESIAN_POINT('Ctrl Pts',(3.96896817222459,140.45989805607,13.1853170078063));
#78514=CARTESIAN_POINT('Ctrl Pts',(3.96639948695296,140.454991930039,13.1343132177153));
#78515=CARTESIAN_POINT('Ctrl Pts',(3.96304235686779,140.445552480088,13.0711537807292));
#78516=CARTESIAN_POINT('Ctrl Pts',(3.96236934615564,140.443518577131,13.0586565503957));
#78517=CARTESIAN_POINT('Ctrl Pts',(3.96126426766466,140.43995880168,13.0384416675561));
#78518=CARTESIAN_POINT('Ctrl Pts',(3.96083751023105,140.438532357344,13.0307069195181));
#78519=CARTESIAN_POINT('Ctrl Pts',(3.96002705522299,140.435728836242,13.0161634079045));
#78520=CARTESIAN_POINT('Ctrl Pts',(3.9596441642781,140.43436548649,13.009352190306));
#78521=CARTESIAN_POINT('Ctrl Pts',(3.95859865643289,140.430536431775,12.9909058019425));
#78522=CARTESIAN_POINT('Ctrl Pts',(3.95793108622625,140.427977344407,12.9792907998497));
#78523=CARTESIAN_POINT('Ctrl Pts',(3.95515483415933,140.416855888449,12.931588212518));
#78524=CARTESIAN_POINT('Ctrl Pts',(3.9529906206915,140.407065234994,12.8958034128813));
#78525=CARTESIAN_POINT('Ctrl Pts',(3.94459923446142,140.364516640614,12.7606827633394));
#78526=CARTESIAN_POINT('Ctrl Pts',(3.93819516766651,140.322505061653,12.6645855781701));
#78527=CARTESIAN_POINT('Ctrl Pts',(3.92898793419198,140.244856830283,12.528730705472));
#78528=CARTESIAN_POINT('Ctrl Pts',(3.92599731878192,140.216728219209,12.4850778032827));
#78529=CARTESIAN_POINT('Ctrl Pts',(3.92203972465949,140.175360037575,12.4278116871143));
#78530=CARTESIAN_POINT('Ctrl Pts',(3.92100053856733,140.164091379071,12.4128275374667));
#78531=CARTESIAN_POINT('Ctrl Pts',(3.91923880735301,140.144291787919,12.3875266733303));
#78532=CARTESIAN_POINT('Ctrl Pts',(3.91851086829859,140.135901725426,12.3771031722908));
#78533=CARTESIAN_POINT('Ctrl Pts',(3.91703393597284,140.118454840155,12.3560262281017));
#78534=CARTESIAN_POINT('Ctrl Pts',(3.91628554258756,140.109385915296,12.3453845691111));
#78535=CARTESIAN_POINT('Ctrl Pts',(3.91437868821074,140.085701650427,12.318386413845));
#78536=CARTESIAN_POINT('Ctrl Pts',(3.91322936510204,140.070868354315,12.3022253058966));
#78537=CARTESIAN_POINT('Ctrl Pts',(3.90598094691075,139.973904239718,12.2012356758357));
#78538=CARTESIAN_POINT('Ctrl Pts',(3.90033833442323,139.882129184797,12.1262785233545));
#78539=CARTESIAN_POINT('Ctrl Pts',(3.89238120764606,139.744387148381,12.0391523330544));
#78540=CARTESIAN_POINT('Ctrl Pts',(3.89016961381543,139.70535038004,12.016906278948));
#78541=CARTESIAN_POINT('Ctrl Pts',(3.88651932870261,139.641335683084,11.9842310113233));
#78542=CARTESIAN_POINT('Ctrl Pts',(3.88512535964433,139.616983478467,11.9726376876532));
#78543=CARTESIAN_POINT('Ctrl Pts',(3.88314274142508,139.582796035947,11.9575061818194));
#78544=CARTESIAN_POINT('Ctrl Pts',(3.88258473334658,139.573221139347,11.9533900400839));
#78545=CARTESIAN_POINT('Ctrl Pts',(3.88161693500578,139.556717614581,11.9465032627926));
#78546=CARTESIAN_POINT('Ctrl Pts',(3.88121006579688,139.549810401357,11.9436827653763));
#78547=CARTESIAN_POINT('Ctrl Pts',(3.88032172934466,139.534802596547,11.9376879515425));
#78548=CARTESIAN_POINT('Ctrl Pts',(3.87983924859187,139.526695186371,11.9345330075545));
#78549=CARTESIAN_POINT('Ctrl Pts',(3.87844760808565,139.503417803409,11.9257129183067));
#78550=CARTESIAN_POINT('Ctrl Pts',(3.87752902467003,139.488181697183,11.9202271729243));
#78551=CARTESIAN_POINT('Ctrl Pts',(3.87263576209454,139.407494779144,11.8926796183376));
#78552=CARTESIAN_POINT('Ctrl Pts',(3.86848685203145,139.340637921975,11.875020313664));
#78553=CARTESIAN_POINT('Ctrl Pts',(3.86014374127758,139.204560953943,11.8492037326183));
#78554=CARTESIAN_POINT('Ctrl Pts',(3.85596079064354,139.135492925998,11.841131326362));
#78555=CARTESIAN_POINT('Ctrl Pts',(3.84908373439546,139.018277317928,11.8358310225527));
#78556=CARTESIAN_POINT('Ctrl Pts',(3.84633334790217,138.970364498649,11.8360166315343));
#78557=CARTESIAN_POINT('Ctrl Pts',(3.84263075183139,138.904282574278,11.8395189814417));
#78558=CARTESIAN_POINT('Ctrl Pts',(3.84161809719459,138.886041308312,11.8408289714711));
#78559=CARTESIAN_POINT('Ctrl Pts',(3.83988705475158,138.854578887924,11.8436820562074));
#78560=CARTESIAN_POINT('Ctrl Pts',(3.83916374590359,138.841345707555,11.8450642333475));
#78561=CARTESIAN_POINT('Ctrl Pts',(3.83768396061898,138.814102905639,11.8482858016616));
#78562=CARTESIAN_POINT('Ctrl Pts',(3.83692828080843,138.800097354914,11.8501480093337));
#78563=CARTESIAN_POINT('Ctrl Pts',(3.83497628356272,138.763696575985,11.855525440397));
#78564=CARTESIAN_POINT('Ctrl Pts',(3.83379000339494,138.74135179744,11.8593587394846));
#78565=CARTESIAN_POINT('Ctrl Pts',(3.82678163231227,138.60828751533,11.8853821633067));
#78566=CARTESIAN_POINT('Ctrl Pts',(3.82136769962694,138.500353465382,11.9198053462218));
#78567=CARTESIAN_POINT('Ctrl Pts',(3.81355275051088,138.354269567926,11.9858047700099));
#78568=CARTESIAN_POINT('Ctrl Pts',(3.81122592844991,138.312068630723,12.0073953166884));
#78569=CARTESIAN_POINT('Ctrl Pts',(3.80740991363426,138.246814161613,12.0448821599283));
#78570=CARTESIAN_POINT('Ctrl Pts',(3.80597057988463,138.223040152559,12.0594586220882));
#78571=CARTESIAN_POINT('Ctrl Pts',(3.80393392049375,138.190868025508,12.080471837516));
#78572=CARTESIAN_POINT('Ctrl Pts',(3.8033694847094,138.1821004754,12.0863345412152));
#78573=CARTESIAN_POINT('Ctrl Pts',(3.8023943832412,138.167226701139,12.0965147294686));
#78574=CARTESIAN_POINT('Ctrl Pts',(3.80198676743256,138.161088912129,12.1007851114584));
#78575=CARTESIAN_POINT('Ctrl Pts',(3.80110157825485,138.147936699133,12.1100861879634));
#78576=CARTESIAN_POINT('Ctrl Pts',(3.80062306992748,138.140933972358,12.1151319477517));
#78577=CARTESIAN_POINT('Ctrl Pts',(3.79925391112954,138.121183754555,12.1296299321361));
#78578=CARTESIAN_POINT('Ctrl Pts',(3.79835427523849,138.108545144009,12.139227719482));
#78579=CARTESIAN_POINT('Ctrl Pts',(3.79271121648546,138.031157533831,12.200005360638));
#78580=CARTESIAN_POINT('Ctrl Pts',(3.78771596629495,137.970682110082,12.2563779836028));
#78581=CARTESIAN_POINT('Ctrl Pts',(3.77880622281925,137.871357519453,12.3660406535302));
#78582=CARTESIAN_POINT('Ctrl Pts',(3.77489039654456,137.830730073361,12.4174338972059));
#78583=CARTESIAN_POINT('Ctrl Pts',(3.76868459473099,137.770337398581,12.5053545947858));
#78584=CARTESIAN_POINT('Ctrl Pts',(3.76633086988188,137.748442817897,12.540304984396));
#78585=CARTESIAN_POINT('Ctrl Pts',(3.76305838130558,137.719442002921,12.5912641816702));
#78586=CARTESIAN_POINT('Ctrl Pts',(3.7620964147948,137.711102775709,12.6065454404336));
#78587=CARTESIAN_POINT('Ctrl Pts',(3.76042321510648,137.696933329037,12.6336494008941));
#78588=CARTESIAN_POINT('Ctrl Pts',(3.75970794376827,137.690986613755,12.6454086462637));
#78589=CARTESIAN_POINT('Ctrl Pts',(3.75821806247147,137.678838684959,12.6702581626843));
#78590=CARTESIAN_POINT('Ctrl Pts',(3.75744468255218,137.672671334046,12.6833634498767));
#78591=CARTESIAN_POINT('Ctrl Pts',(3.75538401435701,137.656624989219,12.7188177564366));
#78592=CARTESIAN_POINT('Ctrl Pts',(3.75410905246291,137.647109260933,12.7413266091364));
#78593=CARTESIAN_POINT('Ctrl Pts',(3.74860499163086,137.607972059841,12.8407761050442));
#78594=CARTESIAN_POINT('Ctrl Pts',(3.74456837703722,137.58431694611,12.91990606702));
#78595=CARTESIAN_POINT('Ctrl Pts',(3.73731512557805,137.553800044451,13.0659263820307));
#78596=CARTESIAN_POINT('Ctrl Pts',(3.73409385448265,137.544633281552,13.1320963501165));
#78597=CARTESIAN_POINT('Ctrl Pts',(3.72904437780249,137.537671566675,13.2323895721751));
#78598=CARTESIAN_POINT('Ctrl Pts',(3.72731356542675,137.5365,13.2661909020476));
#78599=CARTESIAN_POINT('Ctrl Pts',(3.72552751600545,137.5365,13.2999999999998));
#78600=CARTESIAN_POINT('Ctrl Pts',(3.65157748137715,137.5365,13.3000000000035));
#78601=CARTESIAN_POINT('Ctrl Pts',(3.6559595390121,137.5365,13.2235985914167));
#78602=CARTESIAN_POINT('Ctrl Pts',(3.66056768225208,137.542482743807,13.1473188192194));
#78603=CARTESIAN_POINT('Ctrl Pts',(3.66936004533574,137.565232991498,13.0031619070513));
#78604=CARTESIAN_POINT('Ctrl Pts',(3.67353428369732,137.580958599639,12.9353192368978));
#78605=CARTESIAN_POINT('Ctrl Pts',(3.68007346966338,137.614016173195,12.8280886455043));
#78606=CARTESIAN_POINT('Ctrl Pts',(3.68251207469555,137.628358372174,12.787895273671));
#78607=CARTESIAN_POINT('Ctrl Pts',(3.68587396188387,137.651049815535,12.7321325411057));
#78608=CARTESIAN_POINT('Ctrl Pts',(3.68684399021867,137.657954399548,12.7160019733571));
#78609=CARTESIAN_POINT('Ctrl Pts',(3.68852268610921,137.6705293786,12.6880257872626));
#78610=CARTESIAN_POINT('Ctrl Pts',(3.6892355856517,137.676072141994,12.676125322923));
#78611=CARTESIAN_POINT('Ctrl Pts',(3.69071238411208,137.687975716195,12.651441328679));
#78612=CARTESIAN_POINT('Ctrl Pts',(3.69147520262237,137.694365008948,12.6386730300857));
#78613=CARTESIAN_POINT('Ctrl Pts',(3.69348738642181,137.711853620816,12.6049656862361));
#78614=CARTESIAN_POINT('Ctrl Pts',(3.69472535154334,137.723276600438,12.5841988859888));
#78615=CARTESIAN_POINT('Ctrl Pts',(3.70130413365152,137.787449489421,12.4739613712733));
#78616=CARTESIAN_POINT('Ctrl Pts',(3.70631289035946,137.849104639831,12.3900218699495));
#78617=CARTESIAN_POINT('Ctrl Pts',(3.71503692647108,137.969992526518,12.2575950189444));
#78618=CARTESIAN_POINT('Ctrl Pts',(3.7187272117014,138.025081508897,12.2058998390586));
#78619=CARTESIAN_POINT('Ctrl Pts',(3.72340276834783,138.094727030487,12.1499974887333));
#78620=CARTESIAN_POINT('Ctrl Pts',(3.72413811930958,138.105674644592,12.1414633988737));
#78621=CARTESIAN_POINT('Ctrl Pts',(3.72531844024373,138.123194436607,12.1282023427525));
#78622=CARTESIAN_POINT('Ctrl Pts',(3.72575663245445,138.129687535584,12.123371786218));
#78623=CARTESIAN_POINT('Ctrl Pts',(3.72661015792459,138.142303347593,12.1141477795188));
#78624=CARTESIAN_POINT('Ctrl Pts',(3.72702501439003,138.148420498184,12.1097473462109));
#78625=CARTESIAN_POINT('Ctrl Pts',(3.72808430974567,138.164010835324,12.0987139792721));
#78626=CARTESIAN_POINT('Ctrl Pts',(3.72873284863476,138.173529074821,12.0921457953897));
#78627=CARTESIAN_POINT('Ctrl Pts',(3.73131953313215,138.211435226257,12.0666459929452));
#78628=CARTESIAN_POINT('Ctrl Pts',(3.73330454516756,138.240402152435,12.0485978674107));
#78629=CARTESIAN_POINT('Ctrl Pts',(3.74099668692803,138.353285264456,11.9836289133351));
#78630=CARTESIAN_POINT('Ctrl Pts',(3.74687556360808,138.441121135358,11.9440028837653));
#78631=CARTESIAN_POINT('Ctrl Pts',(3.75624718454596,138.590809290217,11.8935080021171));
#78632=CARTESIAN_POINT('Ctrl Pts',(3.75983843349468,138.650606629817,11.8774731937288));
#78633=CARTESIAN_POINT('Ctrl Pts',(3.76441307319211,138.730476774297,11.8613984877837));
#78634=CARTESIAN_POINT('Ctrl Pts',(3.7655026005123,138.749784726641,11.857914895081));
#78635=CARTESIAN_POINT('Ctrl Pts',(3.76731973342343,138.782460885137,11.8526954442103));
#78636=CARTESIAN_POINT('Ctrl Pts',(3.76805370594936,138.795793203704,11.8507542150959));
#78637=CARTESIAN_POINT('Ctrl Pts',(3.76951914198925,138.822673593312,11.8472186584254));
#78638=CARTESIAN_POINT('Ctrl Pts',(3.77025038808297,138.836220938847,11.8456290991434));
#78639=CARTESIAN_POINT('Ctrl Pts',(3.77206619432492,138.870181056187,11.8421249843269));
#78640=CARTESIAN_POINT('Ctrl Pts',(3.77314323531011,138.890615834623,11.84044949435));
#78641=CARTESIAN_POINT('Ctrl Pts',(3.77782905041354,138.980662903238,11.8349682324521));
#78642=CARTESIAN_POINT('Ctrl Pts',(3.78129774082775,139.050463875804,11.8357094864554));
#78643=CARTESIAN_POINT('Ctrl Pts',(3.78970860472904,139.221773486801,11.8497976731603));
#78644=CARTESIAN_POINT('Ctrl Pts',(3.79455420759934,139.322429880264,11.8688097087033));
#78645=CARTESIAN_POINT('Ctrl Pts',(3.80094312821479,139.441914740646,11.9046312610839));
#78646=CARTESIAN_POINT('Ctrl Pts',(3.80211897084394,139.463398976648,11.9116182661255));
#78647=CARTESIAN_POINT('Ctrl Pts',(3.80383804376152,139.493891934969,11.922321639245));
#78648=CARTESIAN_POINT('Ctrl Pts',(3.80436030882322,139.503039495858,11.9256353597822));
#78649=CARTESIAN_POINT('Ctrl Pts',(3.80528296155999,139.518978881099,11.9315898770309));
#78650=CARTESIAN_POINT('Ctrl Pts',(3.80568104985409,139.52578509335,11.9341905784235));
#78651=CARTESIAN_POINT('Ctrl Pts',(3.80657888458789,139.540974485965,11.9401249186257));
#78652=CARTESIAN_POINT('Ctrl Pts',(3.80708011039229,139.549346377047,11.9434852817703));
#78653=CARTESIAN_POINT('Ctrl Pts',(3.80862275282325,139.574806919939,11.9539791389318));
#78654=CARTESIAN_POINT('Ctrl Pts',(3.8096771898035,139.591791154296,11.9613595256413));
#78655=CARTESIAN_POINT('Ctrl Pts',(3.81675792220808,139.703461500401,12.0124256210612));
#78656=CARTESIAN_POINT('Ctrl Pts',(3.82314857806906,139.793383380652,12.0658006937683));
#78657=CARTESIAN_POINT('Ctrl Pts',(3.83233156481164,139.916404085803,12.1578641275573));
#78658=CARTESIAN_POINT('Ctrl Pts',(3.83524590337054,139.954420029233,12.1894353538638));
#78659=CARTESIAN_POINT('Ctrl Pts',(3.84008511997826,140.01617245682,12.2462367012198));
#78660=CARTESIAN_POINT('Ctrl Pts',(3.84204256879515,140.040742288077,12.2704955953336));
#78661=CARTESIAN_POINT('Ctrl Pts',(3.84486968343108,140.075620493591,12.3074585437684));
#78662=CARTESIAN_POINT('Ctrl Pts',(3.84576810047058,140.08660960416,12.3195013579638));
#78663=CARTESIAN_POINT('Ctrl Pts',(3.8473672055468,140.10598985916,12.3414660053249));
#78664=CARTESIAN_POINT('Ctrl Pts',(3.84807090950391,140.114454300091,12.3513205938423));
#78665=CARTESIAN_POINT('Ctrl Pts',(3.84957368263292,140.132383976573,12.3727661223391));
#78666=CARTESIAN_POINT('Ctrl Pts',(3.85037091508543,140.141804957003,12.3843922254662));
#78667=CARTESIAN_POINT('Ctrl Pts',(3.85255550461618,140.167347713134,12.4169211328737));
#78668=CARTESIAN_POINT('Ctrl Pts',(3.85392787961937,140.18308515989,12.4381191588654));
#78669=CARTESIAN_POINT('Ctrl Pts',(3.86152059563325,140.268103248291,12.5593569099986));
#78670=CARTESIAN_POINT('Ctrl Pts',(3.86728023822072,140.325265167053,12.6672992339697));
#78671=CARTESIAN_POINT('Ctrl Pts',(3.87593215114509,140.38767303944,12.831868490789));
#78672=CARTESIAN_POINT('Ctrl Pts',(3.87864837312771,140.404091023392,12.8836937053413));
#78673=CARTESIAN_POINT('Ctrl Pts',(3.88217383030035,140.420764698408,12.9486836125298));
#78674=CARTESIAN_POINT('Ctrl Pts',(3.88285276687226,140.423777854834,12.961101592924));
#78675=CARTESIAN_POINT('Ctrl Pts',(3.88396342406861,140.428380797936,12.9812174701327));
#78676=CARTESIAN_POINT('Ctrl Pts',(3.88438967694581,140.43007190478,12.9888917446427));
#78677=CARTESIAN_POINT('Ctrl Pts',(3.885195338534,140.433125524312,13.0033003438746));
#78678=CARTESIAN_POINT('Ctrl Pts',(3.88557389634429,140.43450258235,13.0100313961806));
#78679=CARTESIAN_POINT('Ctrl Pts',(3.88660031175646,140.43808361763,13.0281855364697));
#78680=CARTESIAN_POINT('Ctrl Pts',(3.88725286792019,140.440198823085,13.0396254115975));
#78681=CARTESIAN_POINT('Ctrl Pts',(3.8898819530568,140.448094364926,13.0853717521105));
#78682=CARTESIAN_POINT('Ctrl Pts',(3.89190725257507,140.452786659995,13.1198524018986));
#78683=CARTESIAN_POINT('Ctrl Pts',(3.90028349260316,140.466880633635,13.2608787353366));
#78684=CARTESIAN_POINT('Ctrl Pts',(3.90683979102233,140.465820146062,13.3681395152964));
#78685=CARTESIAN_POINT('Ctrl Pts',(3.91621259908423,140.446851056471,13.5262481215619));
#78686=CARTESIAN_POINT('Ctrl Pts',(3.91922685476312,140.437844468185,13.5777955916369));
#78687=CARTESIAN_POINT('Ctrl Pts',(3.92320544304582,140.421891484899,13.6469976041969));
#78688=CARTESIAN_POINT('Ctrl Pts',(3.92424329842703,140.417336252384,13.6651584939201));
#78689=CARTESIAN_POINT('Ctrl Pts',(3.92600006245297,140.408947843428,13.6960750332449));
#78690=CARTESIAN_POINT('Ctrl Pts',(3.92672439351498,140.405286819029,13.7088745897112));
#78691=CARTESIAN_POINT('Ctrl Pts',(3.92819150907265,140.397457887946,13.734897541871));
#78692=CARTESIAN_POINT('Ctrl Pts',(3.92893374248915,140.3932756959,13.7481152460229));
#78693=CARTESIAN_POINT('Ctrl Pts',(3.93081911675292,140.382086819839,13.7818053565549));
#78694=CARTESIAN_POINT('Ctrl Pts',(3.93195342471692,140.374812684126,13.8021857489357));
#78695=CARTESIAN_POINT('Ctrl Pts',(3.93927729960581,140.324348613182,13.9342476408025));
#78696=CARTESIAN_POINT('Ctrl Pts',(3.9449938094545,140.268045884759,14.040425815554));
#78697=CARTESIAN_POINT('Ctrl Pts',(3.95300197059865,140.174105246651,14.1747932881044));
#78698=CARTESIAN_POINT('Ctrl Pts',(3.95518081178516,140.147148540434,14.2098550739459));
#78699=CARTESIAN_POINT('Ctrl Pts',(3.95878237032418,140.101450845468,14.2640278231389));
#78700=CARTESIAN_POINT('Ctrl Pts',(3.96016169376737,140.083700500262,14.2839393631438));
#78701=CARTESIAN_POINT('Ctrl Pts',(3.96212485849522,140.058326064124,14.3108833624017));
#78702=CARTESIAN_POINT('Ctrl Pts',(3.96267872459099,140.051155548001,14.3183374843031));
#78703=CARTESIAN_POINT('Ctrl Pts',(3.96363968540931,140.038711716985,14.3310020190881));
#78704=CARTESIAN_POINT('Ctrl Pts',(3.96404390844426,140.03347682495,14.3362494125651));
#78705=CARTESIAN_POINT('Ctrl Pts',(3.96492643957711,140.022051407912,14.3475294141827));
#78706=CARTESIAN_POINT('Ctrl Pts',(3.96540574897659,140.0158472488,14.3535470152796));
#78707=CARTESIAN_POINT('Ctrl Pts',(3.966787466933,139.997952635452,14.3705985228441));
#78708=CARTESIAN_POINT('Ctrl Pts',(3.96769916455442,139.986133510134,14.381494945388));
#78709=CARTESIAN_POINT('Ctrl Pts',(3.97223139678058,139.927184240608,14.4340723373437));
#78710=CARTESIAN_POINT('Ctrl Pts',(3.97599627123935,139.877582270678,14.4728763297018));
#78711=CARTESIAN_POINT('Ctrl Pts',(3.98304077816822,139.780947300625,14.5389042712005));
#78712=CARTESIAN_POINT('Ctrl Pts',(3.98630986891245,139.73459128679,14.5669405815518));
#78713=CARTESIAN_POINT('Ctrl Pts',(3.9921503458027,139.647883558447,14.613019469843));
#78714=CARTESIAN_POINT('Ctrl Pts',(3.99473585633516,139.608063501114,14.6319281078316));
#78715=CARTESIAN_POINT('Ctrl Pts',(3.99910354093672,139.537999086306,14.6613999964778));
#78716=CARTESIAN_POINT('Ctrl Pts',(4.00091024156335,139.508150550561,14.6728205297644));
#78717=CARTESIAN_POINT('Ctrl Pts',(4.00356584191722,139.462962008761,14.6884343340623));
#78718=CARTESIAN_POINT('Ctrl Pts',(4.00443867784491,139.447890073429,14.6933693808845));
#78719=CARTESIAN_POINT('Ctrl Pts',(4.00594189783183,139.421557837628,14.7015199862459));
#78720=CARTESIAN_POINT('Ctrl Pts',(4.00657586982329,139.410333859412,14.7048471152453));
#78721=CARTESIAN_POINT('Ctrl Pts',(4.00800246387277,139.38481504522,14.7120797380649));
#78722=CARTESIAN_POINT('Ctrl Pts',(4.00879238663683,139.370498280608,14.7159035459655));
#78723=CARTESIAN_POINT('Ctrl Pts',(4.01093361213583,139.331203440597,14.7257618087751));
#78724=CARTESIAN_POINT('Ctrl Pts',(4.01227093681568,139.306120124011,14.7313570578386));
#78725=CARTESIAN_POINT('Ctrl Pts',(4.01940991845956,139.169661360009,14.7580449039939));
#78726=CARTESIAN_POINT('Ctrl Pts',(4.02481732361069,139.056274180173,14.7668040410783));
#78727=CARTESIAN_POINT('Ctrl Pts',(4.03246117195231,138.900033933597,14.7607151134656));
#78728=CARTESIAN_POINT('Ctrl Pts',(4.03458388500347,138.857156287189,14.7571469230109));
#78729=CARTESIAN_POINT('Ctrl Pts',(4.03810396074534,138.788503002239,14.7483743202933));
#78730=CARTESIAN_POINT('Ctrl Pts',(4.03946031416457,138.762600955802,14.7443547656003));
#78731=CARTESIAN_POINT('Ctrl Pts',(4.04139606006478,138.726711888992,14.7377939684263));
#78732=CARTESIAN_POINT('Ctrl Pts',(4.04194657371947,138.71662148115,14.7358392981711));
#78733=CARTESIAN_POINT('Ctrl Pts',(4.04290375600285,138.699298700405,14.7322938959975));
#78734=CARTESIAN_POINT('Ctrl Pts',(4.04330761959031,138.692056429221,14.7307542876261));
#78735=CARTESIAN_POINT('Ctrl Pts',(4.0441919269265,138.676348822641,14.7272902717135));
#78736=CARTESIAN_POINT('Ctrl Pts',(4.04467341440647,138.667888840573,14.7253454929711));
#78737=CARTESIAN_POINT('Ctrl Pts',(4.04606752076343,138.643639357422,14.719543421416));
#78738=CARTESIAN_POINT('Ctrl Pts',(4.04698967263832,138.62789658688,14.7154983004126));
#78739=CARTESIAN_POINT('Ctrl Pts',(4.05222164705189,138.540007805663,14.6913477525239));
#78740=CARTESIAN_POINT('Ctrl Pts',(4.05673629204259,138.469425139258,14.6659905546303));
#78741=CARTESIAN_POINT('Ctrl Pts',(4.06547668218033,138.337053820994,14.6066221283293));
#78742=CARTESIAN_POINT('Ctrl Pts',(4.06969138821679,138.275154199536,14.5733259382087));
#78743=CARTESIAN_POINT('Ctrl Pts',(4.07628260744218,138.179679065078,14.512742344237));
#78744=CARTESIAN_POINT('Ctrl Pts',(4.07873436937187,138.144502860815,14.4881900494096));
#78745=CARTESIAN_POINT('Ctrl Pts',(4.08211062087354,138.096497320693,14.4514443232666));
#78746=CARTESIAN_POINT('Ctrl Pts',(4.08308240477574,138.082734844035,14.4405111979827));
#78747=CARTESIAN_POINT('Ctrl Pts',(4.08476309656061,138.05903918876,14.4209805680931));
#78748=CARTESIAN_POINT('Ctrl Pts',(4.08547626664903,138.049018825852,14.4124924738826));
#78749=CARTESIAN_POINT('Ctrl Pts',(4.08695267026238,138.028355264155,14.3945054624182));
#78750=CARTESIAN_POINT('Ctrl Pts',(4.08771483885581,138.017733943762,14.3849834626508));
#78751=CARTESIAN_POINT('Ctrl Pts',(4.08972304396049,137.989889434926,14.3592768196595));
#78752=CARTESIAN_POINT('Ctrl Pts',(4.09095776450311,137.972915866849,14.3428274063508));
#78753=CARTESIAN_POINT('Ctrl Pts',(4.09756780077649,137.883081158669,14.2514447140352));
#78754=CARTESIAN_POINT('Ctrl Pts',(4.10260592464691,137.818008848913,14.169283283989));
#78755=CARTESIAN_POINT('Ctrl Pts',(4.11021619046105,137.734559770707,14.0370105296152));
#78756=CARTESIAN_POINT('Ctrl Pts',(4.11275240513295,137.709233261231,13.9916965908737));
#78757=CARTESIAN_POINT('Ctrl Pts',(4.11686444382543,137.673393637549,13.9187196249728));
#78758=CARTESIAN_POINT('Ctrl Pts',(4.11838035725497,137.661220664982,13.8919189927172));
#78759=CARTESIAN_POINT('Ctrl Pts',(4.12050593524552,137.645731550318,13.8548909103951));
#78760=CARTESIAN_POINT('Ctrl Pts',(4.12107868444872,137.641707180174,13.8449656486929));
#78761=CARTESIAN_POINT('Ctrl Pts',(4.12206127345906,137.635063919493,13.8280506110251));
#78762=CARTESIAN_POINT('Ctrl Pts',(4.12246787956441,137.632388848541,13.821083188101));
#78763=CARTESIAN_POINT('Ctrl Pts',(4.12334197325096,137.626797716945,13.8061809927464));
#78764=CARTESIAN_POINT('Ctrl Pts',(4.12381025777677,137.623896974158,13.7982410687968));
#78765=CARTESIAN_POINT('Ctrl Pts',(4.12513005722918,137.615978320578,13.775969344801));
#78766=CARTESIAN_POINT('Ctrl Pts',(4.12598968430334,137.61111456798,13.7615842786274));
#78767=CARTESIAN_POINT('Ctrl Pts',(4.13198503240694,137.579120818063,13.6618719060824));
#78768=CARTESIAN_POINT('Ctrl Pts',(4.13742270801435,137.559649003968,13.5742919889431));
#78769=CARTESIAN_POINT('Ctrl Pts',(4.1465190212976,137.540485762504,13.4243136421574));
#78770=CARTESIAN_POINT('Ctrl Pts',(4.15019876702927,137.536543412072,13.3627020648448));
#78771=CARTESIAN_POINT('Ctrl Pts',(4.15380065009266,137.536500118786,13.3006810578158));
#78772=CARTESIAN_POINT('Ctrl Pts',(4.15382042339436,137.5365,13.3003405284137));
#78773=CARTESIAN_POINT('Ctrl Pts',(4.15384019369498,137.5365,13.3000000000084));
#78774=CARTESIAN_POINT('Origin',(4.2,139.,13.3));
#78775=CARTESIAN_POINT('',(4.72326784382708,137.5365,13.299999999986));
#78776=CARTESIAN_POINT('',(4.65349091708139,137.5365,13.3000000000138));
#78777=CARTESIAN_POINT('',(4.2,137.5365,13.3));
#78778=CARTESIAN_POINT('Ctrl Pts',(4.72326784382709,137.5365,13.299999999986));
#78779=CARTESIAN_POINT('Ctrl Pts',(4.72061524380913,137.5365,13.3453339538471));
#78780=CARTESIAN_POINT('Ctrl Pts',(4.71801361931224,137.53860639665,13.3906465426194));
#78781=CARTESIAN_POINT('Ctrl Pts',(4.71444138633859,137.544527309669,13.4541839839692));
#78782=CARTESIAN_POINT('Ctrl Pts',(4.7134180312487,137.546589320802,13.4725424436615));
#78783=CARTESIAN_POINT('Ctrl Pts',(4.71167463899143,137.550737327058,13.5040778128034));
#78784=CARTESIAN_POINT('Ctrl Pts',(4.71094949104831,137.552656886909,13.5172739706296));
#78785=CARTESIAN_POINT('Ctrl Pts',(4.7094710256624,137.556971359962,13.5443326401013));
#78786=CARTESIAN_POINT('Ctrl Pts',(4.70871842341543,137.559386331807,13.5581905745248));
#78787=CARTESIAN_POINT('Ctrl Pts',(4.70678543932857,137.566156359927,13.5939805379733));
#78788=CARTESIAN_POINT('Ctrl Pts',(4.70561471242539,137.570814966113,13.6158517843623));
#78789=CARTESIAN_POINT('Ctrl Pts',(4.70306634081857,137.582180418672,13.6637910703942));
#78790=CARTESIAN_POINT('Ctrl Pts',(4.70169559515881,137.589108896027,13.6897982854271));
#78791=CARTESIAN_POINT('Ctrl Pts',(4.69734817772567,137.613644266652,13.7726404065773));
#78792=CARTESIAN_POINT('Ctrl Pts',(4.69444289289453,137.634000460912,13.8285990321994));
#78793=CARTESIAN_POINT('Ctrl Pts',(4.68700466870989,137.69495885825,13.9689093254457));
#78794=CARTESIAN_POINT('Ctrl Pts',(4.68251287172916,137.740337030202,14.0508778103034));
#78795=CARTESIAN_POINT('Ctrl Pts',(4.67685289757051,137.801705914959,14.1403266265909));
#78796=CARTESIAN_POINT('Ctrl Pts',(4.67605988082319,137.810387216702,14.1525719588196));
#78797=CARTESIAN_POINT('Ctrl Pts',(4.67480661410092,137.824195091883,14.1714269787448));
#78798=CARTESIAN_POINT('Ctrl Pts',(4.67435456923428,137.829192801036,14.1781302051289));
#78799=CARTESIAN_POINT('Ctrl Pts',(4.67348574573492,137.838822564522,14.1908178705304));
#78800=CARTESIAN_POINT('Ctrl Pts',(4.67306965128551,137.843444025805,14.1968097814536));
#78801=CARTESIAN_POINT('Ctrl Pts',(4.67203382195927,137.854977300894,14.211525726363));
#78802=CARTESIAN_POINT('Ctrl Pts',(4.67141052552929,137.861942504336,14.2202071790097));
#78803=CARTESIAN_POINT('Ctrl Pts',(4.66893853649453,137.889696386245,14.2540026206678));
#78804=CARTESIAN_POINT('Ctrl Pts',(4.66704650263296,137.911221698844,14.278497131732));
#78805=CARTESIAN_POINT('Ctrl Pts',(4.66147800265538,137.975936429219,14.3473574751078));
#78806=CARTESIAN_POINT('Ctrl Pts',(4.65773413139017,138.02114533015,14.3897279393647));
#78807=CARTESIAN_POINT('Ctrl Pts',(4.64865261700329,138.137540046658,14.4857110019324));
#78808=CARTESIAN_POINT('Ctrl Pts',(4.64336233459033,138.211207212264,14.5359439597559));
#78809=CARTESIAN_POINT('Ctrl Pts',(4.63692862724951,138.310329913068,14.5910397088626));
#78810=CARTESIAN_POINT('Ctrl Pts',(4.63556149513708,138.33196454868,14.6023659605611));
#78811=CARTESIAN_POINT('Ctrl Pts',(4.63341360162938,138.366865154074,14.619538618867));
#78812=CARTESIAN_POINT('Ctrl Pts',(4.63262075420044,138.379951364202,14.625738137889));
#78813=CARTESIAN_POINT('Ctrl Pts',(4.6311191113978,138.40511887321,14.6372069176151));
#78814=CARTESIAN_POINT('Ctrl Pts',(4.63040923946097,138.417183494506,14.6425091553187));
#78815=CARTESIAN_POINT('Ctrl Pts',(4.62877395032389,138.445354060618,14.6544384028692));
#78816=CARTESIAN_POINT('Ctrl Pts',(4.62785274418139,138.461510106765,14.660942384727));
#78817=CARTESIAN_POINT('Ctrl Pts',(4.62477881320439,138.516335551381,14.6818843929356));
#78818=CARTESIAN_POINT('Ctrl Pts',(4.62266996606128,138.555499756284,14.6949751549734));
#78819=CARTESIAN_POINT('Ctrl Pts',(4.61730915445143,138.658186686741,14.7245337516346));
#78820=CARTESIAN_POINT('Ctrl Pts',(4.61412380821832,138.722356023647,14.7384182611133));
#78821=CARTESIAN_POINT('Ctrl Pts',(4.60693935348308,138.868633644632,14.7599119310595));
#78822=CARTESIAN_POINT('Ctrl Pts',(4.60295292946381,138.950881513117,14.7649862391874));
#78823=CARTESIAN_POINT('Ctrl Pts',(4.59784738573456,139.049008834441,14.7627656247637));
#78824=CARTESIAN_POINT('Ctrl Pts',(4.59700942133953,139.064899696617,14.7621467532466));
#78825=CARTESIAN_POINT('Ctrl Pts',(4.5956958951159,139.089401785117,14.7607923160744));
#78826=CARTESIAN_POINT('Ctrl Pts',(4.59522965068714,139.098022288642,14.760239190423));
#78827=CARTESIAN_POINT('Ctrl Pts',(4.59435195000735,139.114093233815,14.7590650683276));
#78828=CARTESIAN_POINT('Ctrl Pts',(4.59394151438726,139.121544565854,14.7584632491666));
#78829=CARTESIAN_POINT('Ctrl Pts',(4.59294528427974,139.139483738102,14.7568759385589));
#78830=CARTESIAN_POINT('Ctrl Pts',(4.59235653955841,139.149966024748,14.7558342596704));
#78831=CARTESIAN_POINT('Ctrl Pts',(4.59019548031936,139.188053226898,14.7516336424636));
#78832=CARTESIAN_POINT('Ctrl Pts',(4.58859200771951,139.215576642738,14.7478020474996));
#78833=CARTESIAN_POINT('Ctrl Pts',(4.58420553275568,139.289427177466,14.7353687199519));
#78834=CARTESIAN_POINT('Ctrl Pts',(4.58138109121222,139.335475147444,14.7253096112762));
#78835=CARTESIAN_POINT('Ctrl Pts',(4.57171610680341,139.49049036792,14.683517750077));
#78836=CARTESIAN_POINT('Ctrl Pts',(4.56489066287521,139.596238515597,14.6413461354945));
#78837=CARTESIAN_POINT('Ctrl Pts',(4.55719925712931,139.715934922768,14.5766283203304));
#78838=CARTESIAN_POINT('Ctrl Pts',(4.55593780948091,139.735557950647,14.5654237485081));
#78839=CARTESIAN_POINT('Ctrl Pts',(4.55391464452965,139.767004786916,14.5464891002431));
#78840=CARTESIAN_POINT('Ctrl Pts',(4.55314318417796,139.778989432255,14.5390346662714));
#78841=CARTESIAN_POINT('Ctrl Pts',(4.55165641420507,139.802064920249,14.5242145655376));
#78842=CARTESIAN_POINT('Ctrl Pts',(4.55094047554314,139.813166740185,14.5168686484249));
#78843=CARTESIAN_POINT('Ctrl Pts',(4.54925189567034,139.839314072328,14.4990496749514));
#78844=CARTESIAN_POINT('Ctrl Pts',(4.54828439141823,139.854266244477,14.4884432920331));
#78845=CARTESIAN_POINT('Ctrl Pts',(4.54480660739406,139.907834774698,14.4489107395221));
#78846=CARTESIAN_POINT('Ctrl Pts',(4.54235867710823,139.945215399676,14.4183596358661));
#78847=CARTESIAN_POINT('Ctrl Pts',(4.53557279854838,140.046384972724,14.3269710087976));
#78848=CARTESIAN_POINT('Ctrl Pts',(4.53136585453615,140.106283400253,14.2621475302998));
#78849=CARTESIAN_POINT('Ctrl Pts',(4.5242997567057,140.194046433971,14.1480597011772));
#78850=CARTESIAN_POINT('Ctrl Pts',(4.52151282410431,140.22553785362,14.1018777984787));
#78851=CARTESIAN_POINT('Ctrl Pts',(4.51789491042624,140.261045618056,14.0428102653399));
#78852=CARTESIAN_POINT('Ctrl Pts',(4.51720085158219,140.267630106552,14.0315169379568));
#78853=CARTESIAN_POINT('Ctrl Pts',(4.51606981659935,140.277975434385,14.013214052116));
#78854=CARTESIAN_POINT('Ctrl Pts',(4.5156386232797,140.281832077576,14.0062591690428));
#78855=CARTESIAN_POINT('Ctrl Pts',(4.51477613502987,140.289368207323,13.9924038041014));
#78856=CARTESIAN_POINT('Ctrl Pts',(4.51434496133859,140.29304943079,13.9855046056288));
#78857=CARTESIAN_POINT('Ctrl Pts',(4.51321909779949,140.302445750852,13.9675494080406));
#78858=CARTESIAN_POINT('Ctrl Pts',(4.51251946431231,140.308075329569,13.9564495845292));
#78859=CARTESIAN_POINT('Ctrl Pts',(4.50910723641913,140.334571586698,13.9025125266296));
#78860=CARTESIAN_POINT('Ctrl Pts',(4.50630157970903,140.353477921117,13.8587481052505));
#78861=CARTESIAN_POINT('Ctrl Pts',(4.4998458088929,140.391464907886,13.7575111675326));
#78862=CARTESIAN_POINT('Ctrl Pts',(4.49617951182463,140.409183511943,13.6996159626668));
#78863=CARTESIAN_POINT('Ctrl Pts',(4.48779353900733,140.441767722605,13.5635320661247));
#78864=CARTESIAN_POINT('Ctrl Pts',(4.48312263413881,140.453947311259,13.4848876952869));
#78865=CARTESIAN_POINT('Ctrl Pts',(4.47747031874333,140.461191682427,13.3847830675418));
#78866=CARTESIAN_POINT('Ctrl Pts',(4.47630646862535,140.462253741338,13.3639011811713));
#78867=CARTESIAN_POINT('Ctrl Pts',(4.4743985819566,140.463272922123,13.329230808299));
#78868=CARTESIAN_POINT('Ctrl Pts',(4.47364680406799,140.463483275162,13.3154533593042));
#78869=CARTESIAN_POINT('Ctrl Pts',(4.47216953385779,140.463514507769,13.2881588164907));
#78870=CARTESIAN_POINT('Ctrl Pts',(4.4714438862747,140.463342739576,13.2746431194095));
#78871=CARTESIAN_POINT('Ctrl Pts',(4.46968422028167,140.462465340623,13.2416184899986));
#78872=CARTESIAN_POINT('Ctrl Pts',(4.4686565901549,140.461556570574,13.2221173199478));
#78873=CARTESIAN_POINT('Ctrl Pts',(4.46452411382651,140.456277016541,13.1429320972543));
#78874=CARTESIAN_POINT('Ctrl Pts',(4.4615197971198,140.448637769159,13.0835222071212));
#78875=CARTESIAN_POINT('Ctrl Pts',(4.45566792211834,140.426294644332,12.9668475265027));
#78876=CARTESIAN_POINT('Ctrl Pts',(4.45282367913398,140.41171996263,12.9096747290141));
#78877=CARTESIAN_POINT('Ctrl Pts',(4.44679792735274,140.374005493121,12.7919403061043));
#78878=CARTESIAN_POINT('Ctrl Pts',(4.44361672799574,140.350213753348,12.7317244313659));
#78879=CARTESIAN_POINT('Ctrl Pts',(4.4394133888414,140.315580022539,12.6586388360612));
#78880=CARTESIAN_POINT('Ctrl Pts',(4.4385599254505,140.308396865528,12.6441093549624));
#78881=CARTESIAN_POINT('Ctrl Pts',(4.4372271592523,140.296988252589,12.6219664753817));
#78882=CARTESIAN_POINT('Ctrl Pts',(4.43675760533899,140.292933482964,12.6142660947776));
#78883=CARTESIAN_POINT('Ctrl Pts',(4.43587749063871,140.285275541539,12.6000323617701));
#78884=CARTESIAN_POINT('Ctrl Pts',(4.43546802553276,140.281690730425,12.5934897204696));
#78885=CARTESIAN_POINT('Ctrl Pts',(4.43447943289447,140.272981014828,12.5778780610627));
#78886=CARTESIAN_POINT('Ctrl Pts',(4.43389747496432,140.267809086137,12.5688359507009));
#78887=CARTESIAN_POINT('Ctrl Pts',(4.43179231625153,140.248922432107,12.5366192614772));
#78888=CARTESIAN_POINT('Ctrl Pts',(4.43023992948614,140.234665841876,12.5137700864426));
#78889=CARTESIAN_POINT('Ctrl Pts',(4.42604350681794,140.19503015121,12.4539841918559));
#78890=CARTESIAN_POINT('Ctrl Pts',(4.42336176831437,140.16857141976,12.4177980494649));
#78891=CARTESIAN_POINT('Ctrl Pts',(4.41355124002165,140.066380135663,12.2907162004508));
#78892=CARTESIAN_POINT('Ctrl Pts',(4.40642153497016,139.981350967856,12.2078556047324));
#78893=CARTESIAN_POINT('Ctrl Pts',(4.39850797964479,139.869847984118,12.1228524484857));
#78894=CARTESIAN_POINT('Ctrl Pts',(4.39728661682781,139.852134989961,12.1099672670553));
#78895=CARTESIAN_POINT('Ctrl Pts',(4.39531081857828,139.822656524541,12.0895191979166));
#78896=CARTESIAN_POINT('Ctrl Pts',(4.39454748063528,139.811060532055,12.0817190956297));
#78897=CARTESIAN_POINT('Ctrl Pts',(4.39306525688809,139.788143506692,12.0667761027732));
#78898=CARTESIAN_POINT('Ctrl Pts',(4.39234592795921,139.776832717028,12.0596200929069));
#78899=CARTESIAN_POINT('Ctrl Pts',(4.39063134363075,139.749428355323,12.0428040566279));
#78900=CARTESIAN_POINT('Ctrl Pts',(4.38964167918662,139.733243825585,12.0332963903809));
#78901=CARTESIAN_POINT('Ctrl Pts',(4.38594435343274,139.671463446012,11.9985842466251));
#78902=CARTESIAN_POINT('Ctrl Pts',(4.38331066303194,139.624714240454,11.9755080521171));
#78903=CARTESIAN_POINT('Ctrl Pts',(4.37548701779975,139.479703507052,11.9133185222476));
#78904=CARTESIAN_POINT('Ctrl Pts',(4.37049556356813,139.378357345495,11.8823101177945));
#78905=CARTESIAN_POINT('Ctrl Pts',(4.363406849765,139.239242829361,11.8557396286439));
#78906=CARTESIAN_POINT('Ctrl Pts',(4.36157267617855,139.203690079903,11.8502982564802));
#78907=CARTESIAN_POINT('Ctrl Pts',(4.35905495496564,139.156263194633,11.8448185410939));
#78908=CARTESIAN_POINT('Ctrl Pts',(4.35842662066347,139.144535125688,11.8436069060677));
#78909=CARTESIAN_POINT('Ctrl Pts',(4.35741707671776,139.125894563764,11.8419085051731));
#78910=CARTESIAN_POINT('Ctrl Pts',(4.3570408182921,139.118990814221,11.8413288819334));
#78911=CARTESIAN_POINT('Ctrl Pts',(4.35622997632615,139.104214740743,11.8401939107736));
#78912=CARTESIAN_POINT('Ctrl Pts',(4.35579457795852,139.096341558384,11.8396531821344));
#78913=CARTESIAN_POINT('Ctrl Pts',(4.35464505300111,139.075701386944,11.8384032544777));
#78914=CARTESIAN_POINT('Ctrl Pts',(4.35392561240461,139.062929051513,11.8377976685513));
#78915=CARTESIAN_POINT('Ctrl Pts',(4.35015562016846,138.996644400834,11.8355249066066));
#78916=CARTESIAN_POINT('Ctrl Pts',(4.34698783984977,138.943081776475,11.8366278953048));
#78917=CARTESIAN_POINT('Ctrl Pts',(4.33672789560924,138.772288474592,11.8495362427571));
#78918=CARTESIAN_POINT('Ctrl Pts',(4.32956424276089,138.656351667912,11.8725509790387));
#78919=CARTESIAN_POINT('Ctrl Pts',(4.32129741046464,138.519115914299,11.9175052109642));
#78920=CARTESIAN_POINT('Ctrl Pts',(4.31979359506577,138.494040061178,11.9264840682957));
#78921=CARTESIAN_POINT('Ctrl Pts',(4.31739925764554,138.453935876973,11.9420915793491));
#78922=CARTESIAN_POINT('Ctrl Pts',(4.31649515605332,138.438750446375,11.9482972683423));
#78923=CARTESIAN_POINT('Ctrl Pts',(4.31488594808555,138.411656240579,11.9599049467496));
#78924=CARTESIAN_POINT('Ctrl Pts',(4.31417778983348,138.39970963308,11.9652136418841));
#78925=CARTESIAN_POINT('Ctrl Pts',(4.31266524806803,138.374152975368,11.9769827422231));
#78926=CARTESIAN_POINT('Ctrl Pts',(4.31186273103771,138.360568246003,11.9834946952689));
#78927=CARTESIAN_POINT('Ctrl Pts',(4.30962179824281,138.322592345118,12.0024252831896));
#78928=CARTESIAN_POINT('Ctrl Pts',(4.3081999258387,138.298444985847,12.0153202882339));
#78929=CARTESIAN_POINT('Ctrl Pts',(4.302493013396,138.201662661238,12.0705465396761));
#78930=CARTESIAN_POINT('Ctrl Pts',(4.29839919908082,138.13237429301,12.1184225302951));
#78931=CARTESIAN_POINT('Ctrl Pts',(4.29015156213149,138.001555283847,12.2265580233159));
#78932=CARTESIAN_POINT('Ctrl Pts',(4.28601050084204,137.940458406364,12.2868178083429));
#78933=CARTESIAN_POINT('Ctrl Pts',(4.28074611099032,137.874993355294,12.3638213943632));
#78934=CARTESIAN_POINT('Ctrl Pts',(4.27993216898166,137.865186055896,12.3757340168827));
#78935=CARTESIAN_POINT('Ctrl Pts',(4.2786484915229,137.850247940468,12.3944751029844));
#78936=CARTESIAN_POINT('Ctrl Pts',(4.27818742170565,137.844985212898,12.401197478999));
#78937=CARTESIAN_POINT('Ctrl Pts',(4.27731325681139,137.835207917254,12.4139142461282));
#78938=CARTESIAN_POINT('Ctrl Pts',(4.27690106272641,137.830680183305,12.4198978944214));
#78939=CARTESIAN_POINT('Ctrl Pts',(4.27589179586616,137.819788962989,12.4345236362853));
#78940=CARTESIAN_POINT('Ctrl Pts',(4.27529157010167,137.813474220414,12.4432013139837));
#78941=CARTESIAN_POINT('Ctrl Pts',(4.27303235851283,137.790279705423,12.4758232592277));
#78942=CARTESIAN_POINT('Ctrl Pts',(4.27133859180853,137.774025505082,12.5002020192344));
#78943=CARTESIAN_POINT('Ctrl Pts',(4.26660342064742,137.731303958476,12.5686428125337));
#78944=CARTESIAN_POINT('Ctrl Pts',(4.26351337388326,137.706409026388,12.6136364328211));
#78945=CARTESIAN_POINT('Ctrl Pts',(4.25380586780446,137.635921784948,12.7585478612234));
#78946=CARTESIAN_POINT('Ctrl Pts',(4.24723054336891,137.599159407215,12.8623556247961));
#78947=CARTESIAN_POINT('Ctrl Pts',(4.23984036412408,137.569535098134,12.9900700359249));
#78948=CARTESIAN_POINT('Ctrl Pts',(4.23865307596634,137.565173513987,13.0109335015103));
#78949=CARTESIAN_POINT('Ctrl Pts',(4.23671752771,137.558730285462,13.0455085653541));
#78950=CARTESIAN_POINT('Ctrl Pts',(4.23596105933893,137.556385137852,13.0591672184189));
#78951=CARTESIAN_POINT('Ctrl Pts',(4.23454010988995,137.552312125227,13.085092005668));
#78952=CARTESIAN_POINT('Ctrl Pts',(4.23387445778955,137.550545307902,13.0973507036926));
#78953=CARTESIAN_POINT('Ctrl Pts',(4.23251030404093,137.547219753015,13.1226993111181));
#78954=CARTESIAN_POINT('Ctrl Pts',(4.23181250406407,137.545681827711,13.1357908375227));
#78955=CARTESIAN_POINT('Ctrl Pts',(4.2300265921284,137.542172459393,13.1696000340503));
#78956=CARTESIAN_POINT('Ctrl Pts',(4.22894654802664,137.540465631519,13.1903424854856));
#78957=CARTESIAN_POINT('Ctrl Pts',(4.22635640040071,137.537401034063,13.2407082029399));
#78958=CARTESIAN_POINT('Ctrl Pts',(4.22485915534941,137.5365,13.2703501628265));
#78959=CARTESIAN_POINT('Ctrl Pts',(4.22337996970853,137.5365,13.299999999996));
#78960=CARTESIAN_POINT('Ctrl Pts',(4.15384019369498,137.5365,13.3000000000084));
#78961=CARTESIAN_POINT('Ctrl Pts',(4.15607472658841,137.5365,13.2615118688951));
#78962=CARTESIAN_POINT('Ctrl Pts',(4.15826981926394,137.538018265763,13.2230364088225));
#78963=CARTESIAN_POINT('Ctrl Pts',(4.16138452616685,137.542414759486,13.1674233280491));
#78964=CARTESIAN_POINT('Ctrl Pts',(4.16234063728151,137.544083120963,13.1502088626569));
#78965=CARTESIAN_POINT('Ctrl Pts',(4.16400620404721,137.547554843945,13.1199782017664));
#78966=CARTESIAN_POINT('Ctrl Pts',(4.16471960742066,137.549229078288,13.1069494169621));
#78967=CARTESIAN_POINT('Ctrl Pts',(4.16619567982448,137.553085232305,13.0798340624415));
#78968=CARTESIAN_POINT('Ctrl Pts',(4.16695729710165,137.555298003072,13.0657532400044));
#78969=CARTESIAN_POINT('Ctrl Pts',(4.16896212673931,137.561716254987,13.0284709664775));
#78970=CARTESIAN_POINT('Ctrl Pts',(4.17019409437374,137.566277391314,13.0053345800878));
#78971=CARTESIAN_POINT('Ctrl Pts',(4.17512285334786,137.587016298755,12.9120725908745));
#78972=CARTESIAN_POINT('Ctrl Pts',(4.17867733745783,137.607797370253,12.843071436529));
#78973=CARTESIAN_POINT('Ctrl Pts',(4.18724347397128,137.670706117532,12.6790640776115));
#78974=CARTESIAN_POINT('Ctrl Pts',(4.19217589461417,137.7180194162,12.5864842493955));
#78975=CARTESIAN_POINT('Ctrl Pts',(4.19839563671274,137.783410891301,12.4863683765902));
#78976=CARTESIAN_POINT('Ctrl Pts',(4.19923411764975,137.792329299431,12.4731887054791));
#78977=CARTESIAN_POINT('Ctrl Pts',(4.20054658233332,137.80640078228,12.4531072847093));
#78978=CARTESIAN_POINT('Ctrl Pts',(4.20101120726351,137.811403084096,12.4461008679168));
#78979=CARTESIAN_POINT('Ctrl Pts',(4.20188418953157,137.820831637893,12.4331382539465));
#78980=CARTESIAN_POINT('Ctrl Pts',(4.20229150759562,137.825241806847,12.4271709835776));
#78981=CARTESIAN_POINT('Ctrl Pts',(4.20327729496526,137.835944467099,12.4129175803851));
#78982=CARTESIAN_POINT('Ctrl Pts',(4.20385861482471,137.842280217851,12.4046646460619));
#78983=CARTESIAN_POINT('Ctrl Pts',(4.20597367810308,137.865442541586,12.375150396395));
#78984=CARTESIAN_POINT('Ctrl Pts',(4.20753707628258,137.882770402185,12.3542911320474));
#78985=CARTESIAN_POINT('Ctrl Pts',(4.21177866697193,137.930619061791,12.2998422352468));
#78986=CARTESIAN_POINT('Ctrl Pts',(4.214495573892,137.962139311721,12.2671708928763));
#78987=CARTESIAN_POINT('Ctrl Pts',(4.22427759497091,138.080331219417,12.1555447967853));
#78988=CARTESIAN_POINT('Ctrl Pts',(4.23133951014079,138.174911759852,12.085583986997));
#78989=CARTESIAN_POINT('Ctrl Pts',(4.23920112383857,138.295971676181,12.0167771759081));
#78990=CARTESIAN_POINT('Ctrl Pts',(4.24042891555272,138.31535059719,12.0063339045895));
#78991=CARTESIAN_POINT('Ctrl Pts',(4.24240909776419,138.347373588144,11.9899979915115));
#78992=CARTESIAN_POINT('Ctrl Pts',(4.24317057485579,138.359878810792,11.9838421911854));
#78993=CARTESIAN_POINT('Ctrl Pts',(4.24464497763192,138.384458341932,11.9721759139507));
#78994=CARTESIAN_POINT('Ctrl Pts',(4.24535841163774,138.396523400525,11.9666492036496));
#78995=CARTESIAN_POINT('Ctrl Pts',(4.24705171010445,138.425558422576,11.9538238200286));
#78996=CARTESIAN_POINT('Ctrl Pts',(4.24802623978598,138.442594855711,11.9466807548848));
#78997=CARTESIAN_POINT('Ctrl Pts',(4.25160258310699,138.506254909727,11.9213954182307));
#78998=CARTESIAN_POINT('Ctrl Pts',(4.25413671055688,138.553665804301,11.9053239774023));
#78999=CARTESIAN_POINT('Ctrl Pts',(4.26137678335802,138.693884513256,11.8656775026844));
#79000=CARTESIAN_POINT('Ctrl Pts',(4.26592427193415,138.788286129175,11.8487370356814));
#79001=CARTESIAN_POINT('Ctrl Pts',(4.27297104799777,138.930352013112,11.837408095101));
#79002=CARTESIAN_POINT('Ctrl Pts',(4.27533008182458,138.977188667297,11.8359286707962));
#79003=CARTESIAN_POINT('Ctrl Pts',(4.27845650512993,139.03665357107,11.8369044351704));
#79004=CARTESIAN_POINT('Ctrl Pts',(4.27912855590273,139.049292043918,11.8372756961673));
#79005=CARTESIAN_POINT('Ctrl Pts',(4.28023072289703,139.069746510032,11.8381419423788));
#79006=CARTESIAN_POINT('Ctrl Pts',(4.28065552394442,139.077566363101,11.8385360046013));
#79007=CARTESIAN_POINT('Ctrl Pts',(4.28151252844178,139.093203606233,11.8394498582668));
#79008=CARTESIAN_POINT('Ctrl Pts',(4.28194472159916,139.10102073758,11.8399697148931));
#79009=CARTESIAN_POINT('Ctrl Pts',(4.28308416592121,139.121463599015,11.8414941686687));
#79010=CARTESIAN_POINT('Ctrl Pts',(4.28379662180679,139.13408087908,11.8425999308707));
#79011=CARTESIAN_POINT('Ctrl Pts',(4.28747903731392,139.198557637978,11.8490949280712));
#79012=CARTESIAN_POINT('Ctrl Pts',(4.29056038634395,139.250113118417,11.8570886422134));
#79013=CARTESIAN_POINT('Ctrl Pts',(4.30030688216188,139.409456753762,11.8905918066465));
#79014=CARTESIAN_POINT('Ctrl Pts',(4.30704757444879,139.514867928042,11.9255900863472));
#79015=CARTESIAN_POINT('Ctrl Pts',(4.31546563218395,139.647184363066,11.9869054016359));
#79016=CARTESIAN_POINT('Ctrl Pts',(4.31745813701234,139.678501142851,12.0028101469375));
#79017=CARTESIAN_POINT('Ctrl Pts',(4.32032485832862,139.723563824557,12.0277749297356));
#79018=CARTESIAN_POINT('Ctrl Pts',(4.32122900209576,139.73777596668,12.035963651045));
#79019=CARTESIAN_POINT('Ctrl Pts',(4.32283430509653,139.762999104231,12.051067034467));
#79020=CARTESIAN_POINT('Ctrl Pts',(4.32353857684145,139.774061119087,12.0578926839658));
#79021=CARTESIAN_POINT('Ctrl Pts',(4.3250383922315,139.797601019457,12.0728542473699));
#79022=CARTESIAN_POINT('Ctrl Pts',(4.3258321710095,139.810048647682,12.0810351543719));
#79023=CARTESIAN_POINT('Ctrl Pts',(4.32803501370844,139.844536163861,12.104462873564));
#79024=CARTESIAN_POINT('Ctrl Pts',(4.32942834291698,139.86628582693,12.1201274073436));
#79025=CARTESIAN_POINT('Ctrl Pts',(4.33536940140819,139.958424254276,12.1904094482468));
#79026=CARTESIAN_POINT('Ctrl Pts',(4.33969559168371,140.024177114373,12.2507950853459));
#79027=CARTESIAN_POINT('Ctrl Pts',(4.34796129116489,140.138448072097,12.3767833530805));
#79028=CARTESIAN_POINT('Ctrl Pts',(4.35189127976683,140.187784750827,12.4411881430152));
#79029=CARTESIAN_POINT('Ctrl Pts',(4.35692571791642,140.240055642322,12.5226050352027));
#79030=CARTESIAN_POINT('Ctrl Pts',(4.35775689949884,140.248359845524,12.5360113978862));
#79031=CARTESIAN_POINT('Ctrl Pts',(4.35906030018459,140.260844324583,12.5569135788284));
#79032=CARTESIAN_POINT('Ctrl Pts',(4.35952336097061,140.265178229208,12.56431672502));
#79033=CARTESIAN_POINT('Ctrl Pts',(4.36039521688847,140.273142837004,12.5782003462117));
#79034=CARTESIAN_POINT('Ctrl Pts',(4.36080300811647,140.27678965871,12.5846709972));
#79035=CARTESIAN_POINT('Ctrl Pts',(4.36179247004454,140.285453544043,12.6003208856314));
#79036=CARTESIAN_POINT('Ctrl Pts',(4.36237704847317,140.290421674015,12.6095265630458));
#79037=CARTESIAN_POINT('Ctrl Pts',(4.3645190165567,140.308103218136,12.6431469583352));
#79038=CARTESIAN_POINT('Ctrl Pts',(4.36610701042705,140.32022524925,12.6678646877221));
#79039=CARTESIAN_POINT('Ctrl Pts',(4.37044014009899,140.350925110714,12.7352041152564));
#79040=CARTESIAN_POINT('Ctrl Pts',(4.37322579466914,140.368180924087,12.7783932322061));
#79041=CARTESIAN_POINT('Ctrl Pts',(4.38293779713587,140.420846521304,12.9309142816477));
#79042=CARTESIAN_POINT('Ctrl Pts',(4.38985318374172,140.445432061495,13.0435565857797));
#79043=CARTESIAN_POINT('Ctrl Pts',(4.39760789358402,140.458756688159,13.1801649168837));
#79044=CARTESIAN_POINT('Ctrl Pts',(4.39885502942365,140.460416330658,13.20245133984));
#79045=CARTESIAN_POINT('Ctrl Pts',(4.40085807773653,140.462284942251,13.2387536449457));
#79046=CARTESIAN_POINT('Ctrl Pts',(4.40162348130133,140.462804073718,13.2527492918936));
#79047=CARTESIAN_POINT('Ctrl Pts',(4.40310012625846,140.463422956029,13.2799828698539));
#79048=CARTESIAN_POINT('Ctrl Pts',(4.40381196462155,140.463544145673,13.2932189071393));
#79049=CARTESIAN_POINT('Ctrl Pts',(4.40549293358754,140.463405210924,13.3247180023036));
#79050=CARTESIAN_POINT('Ctrl Pts',(4.40645694290561,140.462982807187,13.3429783231926));
#79051=CARTESIAN_POINT('Ctrl Pts',(4.40993133599375,140.460200443284,13.4094270583793));
#79052=CARTESIAN_POINT('Ctrl Pts',(4.41237929135753,140.455800031882,13.4575006173614));
#79053=CARTESIAN_POINT('Ctrl Pts',(4.41917243735557,140.436658022981,13.5926255284767));
#79054=CARTESIAN_POINT('Ctrl Pts',(4.42338589466456,140.416410351921,13.678678694971));
#79055=CARTESIAN_POINT('Ctrl Pts',(4.43045813602883,140.370896496535,13.8153564368705));
#79056=CARTESIAN_POINT('Ctrl Pts',(4.43324411987877,140.350241329141,13.8672712804011));
#79057=CARTESIAN_POINT('Ctrl Pts',(4.43685858259673,140.321175226722,13.9296807888178));
#79058=CARTESIAN_POINT('Ctrl Pts',(4.43755011055743,140.315519445971,13.9414128463607));
#79059=CARTESIAN_POINT('Ctrl Pts',(4.43867630317367,140.306177936797,13.9601469751066));
#79060=CARTESIAN_POINT('Ctrl Pts',(4.43910521712508,140.302590571982,13.967197592269));
#79061=CARTESIAN_POINT('Ctrl Pts',(4.43996203409697,140.295371713058,13.9811054109097));
#79062=CARTESIAN_POINT('Ctrl Pts',(4.44038980146203,140.291742511708,13.9879634670568));
#79063=CARTESIAN_POINT('Ctrl Pts',(4.44150442629145,140.282215954222,14.0056245314454));
#79064=CARTESIAN_POINT('Ctrl Pts',(4.4421961032529,140.276236629808,14.0163824235733));
#79065=CARTESIAN_POINT('Ctrl Pts',(4.44552117242477,140.247133961319,14.0672225057958));
#79066=CARTESIAN_POINT('Ctrl Pts',(4.44824247441362,140.22225538904,14.1062658160743));
#79067=CARTESIAN_POINT('Ctrl Pts',(4.45764078123967,140.131383440153,14.2349814341667));
#79068=CARTESIAN_POINT('Ctrl Pts',(4.46443966126184,140.05702367351,14.3182948759328));
#79069=CARTESIAN_POINT('Ctrl Pts',(4.4731259126145,139.945314792796,14.41789200921));
#79070=CARTESIAN_POINT('Ctrl Pts',(4.47531218732434,139.915700060866,14.4422768381431));
#79071=CARTESIAN_POINT('Ctrl Pts',(4.47841368021054,139.871451882207,14.4758827133057));
#79072=CARTESIAN_POINT('Ctrl Pts',(4.47936516660053,139.857561132568,14.4860512122345));
#79073=CARTESIAN_POINT('Ctrl Pts',(4.48102544600319,139.832769383045,14.5035363006908));
#79074=CARTESIAN_POINT('Ctrl Pts',(4.48173810907615,139.821943491134,14.5109555670904));
#79075=CARTESIAN_POINT('Ctrl Pts',(4.48321526204958,139.799125441095,14.5261463742231));
#79076=CARTESIAN_POINT('Ctrl Pts',(4.4839786578458,139.787116279016,14.5338899402026));
#79077=CARTESIAN_POINT('Ctrl Pts',(4.48599437570639,139.754845114647,14.5540356322645));
#79078=CARTESIAN_POINT('Ctrl Pts',(4.48723522260499,139.734390943077,14.5661226400624));
#79079=CARTESIAN_POINT('Ctrl Pts',(4.49223878229768,139.649683184851,14.6134353397257));
#79080=CARTESIAN_POINT('Ctrl Pts',(4.49585354788017,139.583119267484,14.6443116633613));
#79081=CARTESIAN_POINT('Ctrl Pts',(4.50349064738112,139.436430045322,14.6993994975616));
#79082=CARTESIAN_POINT('Ctrl Pts',(4.50748617562391,139.355982038661,14.7219933863773));
#79083=CARTESIAN_POINT('Ctrl Pts',(4.51315067967486,139.246042824063,14.7429512498732));
#79084=CARTESIAN_POINT('Ctrl Pts',(4.51461990057514,139.217883352072,14.7474709086357));
#79085=CARTESIAN_POINT('Ctrl Pts',(4.51670410694126,139.178832909682,14.7525733043793));
#79086=CARTESIAN_POINT('Ctrl Pts',(4.51728509833133,139.168039160471,14.7538614929084));
#79087=CARTESIAN_POINT('Ctrl Pts',(4.5182772899113,139.149787369549,14.7558338055957));
#79088=CARTESIAN_POINT('Ctrl Pts',(4.51868509143302,139.142336416472,14.7565811577237));
#79089=CARTESIAN_POINT('Ctrl Pts',(4.51955623090263,139.126535283995,14.7580436559551));
#79090=CARTESIAN_POINT('Ctrl Pts',(4.52002027989087,139.11818429914,14.7587443042348));
#79091=CARTESIAN_POINT('Ctrl Pts',(4.52133938144975,139.094614844516,14.7605180694513));
#79092=CARTESIAN_POINT('Ctrl Pts',(4.52220274678679,139.079385344195,14.7614249654902));
#79093=CARTESIAN_POINT('Ctrl Pts',(4.52421434770709,139.044273616558,14.7629653899106));
#79094=CARTESIAN_POINT('Ctrl Pts',(4.5253692183087,139.024387228937,14.7634319538735));
#79095=CARTESIAN_POINT('Ctrl Pts',(4.52948969943811,138.954143630889,14.763647862995));
#79096=CARTESIAN_POINT('Ctrl Pts',(4.53251549486401,138.903816500256,14.7612036772121));
#79097=CARTESIAN_POINT('Ctrl Pts',(4.54200948280427,138.746987118872,14.7454491140233));
#79098=CARTESIAN_POINT('Ctrl Pts',(4.54844624827276,138.641742350195,14.723023743515));
#79099=CARTESIAN_POINT('Ctrl Pts',(4.55584159818675,138.517736029587,14.681954450664));
#79100=CARTESIAN_POINT('Ctrl Pts',(4.55714595008593,138.495764719356,14.6740900664668));
#79101=CARTESIAN_POINT('Ctrl Pts',(4.55921660185348,138.460735912598,14.6605984794889));
#79102=CARTESIAN_POINT('Ctrl Pts',(4.55999362517918,138.447556612074,14.6553008158658));
#79103=CARTESIAN_POINT('Ctrl Pts',(4.56147779752238,138.422325593943,14.6447295316362));
#79104=CARTESIAN_POINT('Ctrl Pts',(4.56218579288799,138.410263810942,14.6394836600474));
#79105=CARTESIAN_POINT('Ctrl Pts',(4.56383494720659,138.382120329102,14.6267897321185));
#79106=CARTESIAN_POINT('Ctrl Pts',(4.56477153368218,138.366099789032,14.6192106881229));
#79107=CARTESIAN_POINT('Ctrl Pts',(4.56799853473739,138.310836042586,14.5918271010185));
#79108=CARTESIAN_POINT('Ctrl Pts',(4.57023827876785,138.27234903339,14.5705466274166));
#79109=CARTESIAN_POINT('Ctrl Pts',(4.57610858690483,138.172286305583,14.5091787369855));
#79110=CARTESIAN_POINT('Ctrl Pts',(4.5796525711301,138.112672446209,14.4661361168609));
#79111=CARTESIAN_POINT('Ctrl Pts',(4.58665240335781,138.002708581535,14.3734061090697));
#79112=CARTESIAN_POINT('Ctrl Pts',(4.59009890308002,137.95222787324,14.3241887643335));
#79113=CARTESIAN_POINT('Ctrl Pts',(4.59459720308539,137.894781716608,14.259471212818));
#79114=CARTESIAN_POINT('Ctrl Pts',(4.59544675541706,137.884273809671,14.247231486277));
#79115=CARTESIAN_POINT('Ctrl Pts',(4.59677296166917,137.868442384981,14.228161904938));
#79116=CARTESIAN_POINT('Ctrl Pts',(4.5972399490073,137.862973304891,14.2214539841473));
#79117=CARTESIAN_POINT('Ctrl Pts',(4.59811468002497,137.852932862765,14.2089137149107));
#79118=CARTESIAN_POINT('Ctrl Pts',(4.59852133145856,137.848345824272,14.203094573959));
#79119=CARTESIAN_POINT('Ctrl Pts',(4.59950178623109,137.837474772798,14.1890859907664));
#79120=CARTESIAN_POINT('Ctrl Pts',(4.6000783567779,137.831232940549,14.1808645474776));
#79121=CARTESIAN_POINT('Ctrl Pts',(4.60215482182166,137.809264712078,14.1512844557708));
#79122=CARTESIAN_POINT('Ctrl Pts',(4.60368303567754,137.794033341633,14.1295661522787));
#79123=CARTESIAN_POINT('Ctrl Pts',(4.60779563820658,137.755224738493,14.0709001319609));
#79124=CARTESIAN_POINT('Ctrl Pts',(4.61041625493469,137.732702791868,14.0332870496166));
#79125=CARTESIAN_POINT('Ctrl Pts',(4.61961011309098,137.660132224584,13.8987326932972));
#79126=CARTESIAN_POINT('Ctrl Pts',(4.6261989894649,137.619245512181,13.7972420806901));
#79127=CARTESIAN_POINT('Ctrl Pts',(4.63385416431974,137.583308717479,13.6680279026232));
#79128=CARTESIAN_POINT('Ctrl Pts',(4.63526437986805,137.577221561168,13.6437445978089));
#79129=CARTESIAN_POINT('Ctrl Pts',(4.63753889101354,137.568288659596,13.6037894219891));
#79130=CARTESIAN_POINT('Ctrl Pts',(4.63841472944284,137.565070658528,13.5882068498785));
#79131=CARTESIAN_POINT('Ctrl Pts',(4.63998979705221,137.559692067439,13.5598335493491));
#79132=CARTESIAN_POINT('Ctrl Pts',(4.64069166069231,137.557446232436,13.547060836032));
#79133=CARTESIAN_POINT('Ctrl Pts',(4.64204800344924,137.553404150259,13.5221341739343));
#79134=CARTESIAN_POINT('Ctrl Pts',(4.64270297354198,137.551590594976,13.5099841697536));
#79135=CARTESIAN_POINT('Ctrl Pts',(4.64415000269553,137.547896026201,13.4829010368947));
#79136=CARTESIAN_POINT('Ctrl Pts',(4.64493963952388,137.546091947451,13.4679587339457));
#79137=CARTESIAN_POINT('Ctrl Pts',(4.64838128406959,137.539176794057,13.4021713089129));
#79138=CARTESIAN_POINT('Ctrl Pts',(4.65095968919661,137.5365,13.3511048930752));
#79139=CARTESIAN_POINT('Ctrl Pts',(4.65349091708139,137.5365,13.3000000000138));
#79140=CARTESIAN_POINT('Origin',(4.2,139.,13.3));
#79141=CARTESIAN_POINT('',(5.22549387428705,137.5365,13.2999999999999));
#79142=CARTESIAN_POINT('',(5.15144231116594,137.5365,13.3));
#79143=CARTESIAN_POINT('',(4.2,137.5365,13.3));
#79144=CARTESIAN_POINT('Ctrl Pts',(5.22549387428705,137.5365,13.2999999999999));
#79145=CARTESIAN_POINT('Ctrl Pts',(5.22431648033678,137.5365,13.3208217959711));
#79146=CARTESIAN_POINT('Ctrl Pts',(5.22311897584145,137.536944360793,13.3416403099394));
#79147=CARTESIAN_POINT('Ctrl Pts',(5.21846390751971,137.540355485263,13.4215175314062));
#79148=CARTESIAN_POINT('Ctrl Pts',(5.21490846015814,137.546456176573,13.4803836302408));
#79149=CARTESIAN_POINT('Ctrl Pts',(5.20729369344285,137.567074131322,13.6050936794817));
#79150=CARTESIAN_POINT('Ctrl Pts',(5.2032430825151,137.582612999915,13.6706397550122));
#79151=CARTESIAN_POINT('Ctrl Pts',(5.19644604084043,137.617049107716,13.7812909378183));
#79152=CARTESIAN_POINT('Ctrl Pts',(5.19365270477895,137.633794068136,13.8269499321652));
#79153=CARTESIAN_POINT('Ctrl Pts',(5.18990422377233,137.65995846791,13.8886072377813));
#79154=CARTESIAN_POINT('Ctrl Pts',(5.18888660424214,137.667453348639,13.9053835589099));
#79155=CARTESIAN_POINT('Ctrl Pts',(5.18714983477347,137.680922800274,13.934070154979));
#79156=CARTESIAN_POINT('Ctrl Pts',(5.18642567596165,137.686747635177,13.9460478797736));
#79157=CARTESIAN_POINT('Ctrl Pts',(5.18494652791685,137.699073575902,13.9705381857021));
#79158=CARTESIAN_POINT('Ctrl Pts',(5.18419229718666,137.705593645546,13.9830396971194));
#79159=CARTESIAN_POINT('Ctrl Pts',(5.18224925247977,137.722995725423,14.0152618858895));
#79160=CARTESIAN_POINT('Ctrl Pts',(5.18107029499875,137.734154297162,14.0348293751879));
#79161=CARTESIAN_POINT('Ctrl Pts',(5.17401263216525,137.804489654537,14.1518080432635));
#79162=CARTESIAN_POINT('Ctrl Pts',(5.16855169606009,137.874425432198,14.2422873462168));
#79163=CARTESIAN_POINT('Ctrl Pts',(5.16070838078417,137.986934110349,14.3572253827301));
#79164=CARTESIAN_POINT('Ctrl Pts',(5.15840574566655,138.021300340968,14.3891164018531));
#79165=CARTESIAN_POINT('Ctrl Pts',(5.15462439430924,138.078315182926,14.4371439100982));
#79166=CARTESIAN_POINT('Ctrl Pts',(5.15319443863056,138.099996351133,14.4543796710292));
#79167=CARTESIAN_POINT('Ctrl Pts',(5.15116894004427,138.130570668894,14.4773001284452));
#79168=CARTESIAN_POINT('Ctrl Pts',(5.150605815392,138.139056882537,14.4835201264684));
#79169=CARTESIAN_POINT('Ctrl Pts',(5.14963220817474,138.153684740911,14.4940010866857));
#79170=CARTESIAN_POINT('Ctrl Pts',(5.1492247491626,138.159793199931,14.4983074081484));
#79171=CARTESIAN_POINT('Ctrl Pts',(5.14833893985886,138.173038248708,14.5074937873587));
#79172=CARTESIAN_POINT('Ctrl Pts',(5.14785963888882,138.180185164641,14.5123574607467));
#79173=CARTESIAN_POINT('Ctrl Pts',(5.14648600893945,138.200626294917,14.5260048184096));
#79174=CARTESIAN_POINT('Ctrl Pts',(5.14558260813531,138.21402109619,14.5346348674491));
#79175=CARTESIAN_POINT('Ctrl Pts',(5.13996987247755,138.297137283842,14.5862845249898));
#79176=CARTESIAN_POINT('Ctrl Pts',(5.13501289323092,138.370224414343,14.6236030014981));
#79177=CARTESIAN_POINT('Ctrl Pts',(5.12611934787148,138.50691583713,14.6795018385329));
#79178=CARTESIAN_POINT('Ctrl Pts',(5.12218275058585,138.56940059672,14.7002652097761));
#79179=CARTESIAN_POINT('Ctrl Pts',(5.11594971739297,138.673096359438,14.7271213988878));
#79180=CARTESIAN_POINT('Ctrl Pts',(5.11358877472775,138.713542318993,14.7357868719834));
#79181=CARTESIAN_POINT('Ctrl Pts',(5.11030835350008,138.771480765783,14.7456537658146));
#79182=CARTESIAN_POINT('Ctrl Pts',(5.10934538263123,138.788708976814,14.7482720709701));
#79183=CARTESIAN_POINT('Ctrl Pts',(5.10767104980481,138.819042813287,14.752329310508));
#79184=CARTESIAN_POINT('Ctrl Pts',(5.10695563241221,138.832128530929,14.7538999674374));
#79185=CARTESIAN_POINT('Ctrl Pts',(5.10546602418558,138.859627448787,14.7568243928691));
#79186=CARTESIAN_POINT('Ctrl Pts',(5.10469305388997,138.874043158052,14.7581415086025));
#79187=CARTESIAN_POINT('Ctrl Pts',(5.10263489763599,138.912797624306,14.7611033408969));
#79188=CARTESIAN_POINT('Ctrl Pts',(5.10136198308602,138.937162345626,14.7623538373338));
#79189=CARTESIAN_POINT('Ctrl Pts',(5.0953846989902,139.053174861332,14.765403010299));
#79190=CARTESIAN_POINT('Ctrl Pts',(5.09092659283357,139.144830604221,14.7591981909216));
#79191=CARTESIAN_POINT('Ctrl Pts',(5.083557811952,139.294499947794,14.7348166941196));
#79192=CARTESIAN_POINT('Ctrl Pts',(5.0806472093606,139.353042359927,14.7215447744809));
#79193=CARTESIAN_POINT('Ctrl Pts',(5.07601317639603,139.441351221602,14.6957319367232));
#79194=CARTESIAN_POINT('Ctrl Pts',(5.07436908577361,139.471794943004,14.6857372784024));
#79195=CARTESIAN_POINT('Ctrl Pts',(5.07208987477992,139.512278453656,14.6709578686598));
#79196=CARTESIAN_POINT('Ctrl Pts',(5.07149878865746,139.522629098198,14.6670455378476));
#79197=CARTESIAN_POINT('Ctrl Pts',(5.07049276547103,139.539971451507,14.6602647454083));
#79198=CARTESIAN_POINT('Ctrl Pts',(5.07008140083164,139.546987307034,14.6574587400175));
#79199=CARTESIAN_POINT('Ctrl Pts',(5.06920633791023,139.561744841373,14.6514234491596));
#79200=CARTESIAN_POINT('Ctrl Pts',(5.06874197743711,139.569480888435,14.6481817816459));
#79201=CARTESIAN_POINT('Ctrl Pts',(5.06742929754634,139.59109969396,14.6389034954454));
#79202=CARTESIAN_POINT('Ctrl Pts',(5.06657284404308,139.604916925543,14.6327178602115));
#79203=CARTESIAN_POINT('Ctrl Pts',(5.06042488099548,139.702294296705,14.5872981288399));
#79204=CARTESIAN_POINT('Ctrl Pts',(5.05481085427807,139.782068756456,14.5404516704972));
#79205=CARTESIAN_POINT('Ctrl Pts',(5.04450560618098,139.921001405237,14.4401062183733));
#79206=CARTESIAN_POINT('Ctrl Pts',(5.03981278437006,139.981256226024,14.3886802167703));
#79207=CARTESIAN_POINT('Ctrl Pts',(5.03377431621596,140.056020141462,14.3135952660986));
#79208=CARTESIAN_POINT('Ctrl Pts',(5.03226481078145,140.074447906305,14.2940401062208));
#79209=CARTESIAN_POINT('Ctrl Pts',(5.02994978801104,140.102287472923,14.262818018029));
#79210=CARTESIAN_POINT('Ctrl Pts',(5.02912873020647,140.112075474131,14.2514958602498));
#79211=CARTESIAN_POINT('Ctrl Pts',(5.02760325243495,140.130091922281,14.2299976718177));
#79212=CARTESIAN_POINT('Ctrl Pts',(5.0268972212633,140.138360825223,14.21985763538));
#79213=CARTESIAN_POINT('Ctrl Pts',(5.02531051656691,140.156776801803,14.1966456706902));
#79214=CARTESIAN_POINT('Ctrl Pts',(5.02443319537824,140.16684046828,14.1835096939502));
#79215=CARTESIAN_POINT('Ctrl Pts',(5.02169319657924,140.197860823561,14.1415644114764));
#79216=CARTESIAN_POINT('Ctrl Pts',(5.01986179067266,140.217990296151,14.1121582994356));
#79217=CARTESIAN_POINT('Ctrl Pts',(5.01249800742321,140.295840750304,13.9890156029986));
#79218=CARTESIAN_POINT('Ctrl Pts',(5.00728157368047,140.343969674476,13.8896531849894));
#79219=CARTESIAN_POINT('Ctrl Pts',(4.99930229820903,140.397759585905,13.7368085105194));
#79220=CARTESIAN_POINT('Ctrl Pts',(4.99669734801785,140.412387922633,13.6869017447962));
#79221=CARTESIAN_POINT('Ctrl Pts',(4.99329824343388,140.427249520676,13.6239636512686));
#79222=CARTESIAN_POINT('Ctrl Pts',(4.99262305764535,140.430007821726,13.6115625934559));
#79223=CARTESIAN_POINT('Ctrl Pts',(4.99151530026912,140.434213669998,13.5914196324865));
#79224=CARTESIAN_POINT('Ctrl Pts',(4.9910880874694,140.435760826695,13.5836989535385));
#79225=CARTESIAN_POINT('Ctrl Pts',(4.99027754234871,140.438554228036,13.5691507892851));
#79226=CARTESIAN_POINT('Ctrl Pts',(4.98989502755304,140.439814362344,13.5623261562576));
#79227=CARTESIAN_POINT('Ctrl Pts',(4.98885191915191,140.443096014263,13.5438170543221));
#79228=CARTESIAN_POINT('Ctrl Pts',(4.98818641009163,140.445024096006,13.532116793384));
#79229=CARTESIAN_POINT('Ctrl Pts',(4.98543512099859,140.452335038783,13.4841231767654));
#79230=CARTESIAN_POINT('Ctrl Pts',(4.98329502740733,140.456494015416,13.4476590858289));
#79231=CARTESIAN_POINT('Ctrl Pts',(4.97490769957814,140.467245002696,13.3064215570208));
#79232=CARTESIAN_POINT('Ctrl Pts',(4.96847894171036,140.463930188275,13.2012076657758));
#79233=CARTESIAN_POINT('Ctrl Pts',(4.95924429192299,140.442188488971,13.0457861633595));
#79234=CARTESIAN_POINT('Ctrl Pts',(4.956249362654,140.432253592853,12.994741330572));
#79235=CARTESIAN_POINT('Ctrl Pts',(4.95228722505338,140.415065497773,12.9261369225789));
#79236=CARTESIAN_POINT('Ctrl Pts',(4.95124758902434,140.410158350388,12.9080338833798));
#79237=CARTESIAN_POINT('Ctrl Pts',(4.94948533529721,140.401155994288,12.8771842211054));
#79238=CARTESIAN_POINT('Ctrl Pts',(4.94875731558008,140.397231474106,12.86439062496));
#79239=CARTESIAN_POINT('Ctrl Pts',(4.9472804193623,140.388849607488,12.838346000716));
#79240=CARTESIAN_POINT('Ctrl Pts',(4.94653213955791,140.384376747959,12.825101394582));
#79241=CARTESIAN_POINT('Ctrl Pts',(4.9446259938738,140.372403904487,12.7912561322809));
#79242=CARTESIAN_POINT('Ctrl Pts',(4.94347725197428,140.364629455367,12.7707559016435));
#79243=CARTESIAN_POINT('Ctrl Pts',(4.9362252062303,140.312031472422,12.6409367650834));
#79244=CARTESIAN_POINT('Ctrl Pts',(4.93057914401306,140.25457188878,12.5372144466056));
#79245=CARTESIAN_POINT('Ctrl Pts',(4.9226197969618,140.158942398364,12.405182519189));
#79246=CARTESIAN_POINT('Ctrl Pts',(4.92040989973246,140.130964277353,12.3700724757106));
#79247=CARTESIAN_POINT('Ctrl Pts',(4.91676206613021,140.083670618105,12.3160199488406));
#79248=CARTESIAN_POINT('Ctrl Pts',(4.91536877810655,140.06536600081,12.2962301732213));
#79249=CARTESIAN_POINT('Ctrl Pts',(4.91338697196033,140.039242414412,12.269506896768));
#79250=CARTESIAN_POINT('Ctrl Pts',(4.91282906174203,140.031879099899,12.2621337551059));
#79251=CARTESIAN_POINT('Ctrl Pts',(4.9118613739175,140.019109618759,12.249617449956));
#79252=CARTESIAN_POINT('Ctrl Pts',(4.91145451540155,140.013741810766,12.2444359536495));
#79253=CARTESIAN_POINT('Ctrl Pts',(4.91056612817975,140.002028284513,12.2333007591275));
#79254=CARTESIAN_POINT('Ctrl Pts',(4.91008358473448,139.995669031698,12.2273625379867));
#79255=CARTESIAN_POINT('Ctrl Pts',(4.90869158810821,139.977320149219,12.2105322584695));
#79256=CARTESIAN_POINT('Ctrl Pts',(4.90777270424951,139.96520245095,12.1997823766872));
#79257=CARTESIAN_POINT('Ctrl Pts',(4.90313870872369,139.903921509832,12.147210275159));
#79258=CARTESIAN_POINT('Ctrl Pts',(4.8992720420793,139.852210516469,12.1084739714692));
#79259=CARTESIAN_POINT('Ctrl Pts',(4.89183240199377,139.7486353442,12.0410869216755));
#79260=CARTESIAN_POINT('Ctrl Pts',(4.88826911363359,139.697249759838,12.0119160375971));
#79261=CARTESIAN_POINT('Ctrl Pts',(4.88122387674749,139.590465039665,11.959563403886));
#79262=CARTESIAN_POINT('Ctrl Pts',(4.87775068112213,139.535116749234,11.9365225949072));
#79263=CARTESIAN_POINT('Ctrl Pts',(4.87329227671756,139.460055272962,11.9105531330193));
#79264=CARTESIAN_POINT('Ctrl Pts',(4.87220820256922,139.441477533651,11.9045391121224));
#79265=CARTESIAN_POINT('Ctrl Pts',(4.8703941252912,139.409843985337,11.8949936448065));
#79266=CARTESIAN_POINT('Ctrl Pts',(4.86965790811844,139.396849851136,11.8912682429645));
#79267=CARTESIAN_POINT('Ctrl Pts',(4.86818303625158,139.370510858223,11.8841102586444));
#79268=CARTESIAN_POINT('Ctrl Pts',(4.86744468255715,139.357165410997,11.8806850445975));
#79269=CARTESIAN_POINT('Ctrl Pts',(4.86560110869692,139.323457670658,11.8725392434399));
#79270=CARTESIAN_POINT('Ctrl Pts',(4.86450381242269,139.303038620099,11.8680653895067));
#79271=CARTESIAN_POINT('Ctrl Pts',(4.85930034877243,139.204657337507,11.8487086668416));
#79272=CARTESIAN_POINT('Ctrl Pts',(4.85538129394282,139.125662589388,11.8397459995933));
#79273=CARTESIAN_POINT('Ctrl Pts',(4.84856790425203,138.985923751041,11.8353204378668));
#79274=CARTESIAN_POINT('Ctrl Pts',(4.84565586842749,138.925462449639,11.8371506670341));
#79275=CARTESIAN_POINT('Ctrl Pts',(4.84030771838227,138.817711515504,11.8471111082985));
#79276=CARTESIAN_POINT('Ctrl Pts',(4.83790196758462,138.770381561137,11.8538361629626));
#79277=CARTESIAN_POINT('Ctrl Pts',(4.83473357131472,138.711239614577,11.8652161144749));
#79278=CARTESIAN_POINT('Ctrl Pts',(4.83407118444928,138.699040651448,11.8677253027943));
#79279=CARTESIAN_POINT('Ctrl Pts',(4.83297916583313,138.67923506587,11.8720632767878));
#79280=CARTESIAN_POINT('Ctrl Pts',(4.83255460970626,138.671608205385,11.873797962008));
#79281=CARTESIAN_POINT('Ctrl Pts',(4.83174446885236,138.657203079681,11.8771959975687));
#79282=CARTESIAN_POINT('Ctrl Pts',(4.83135963611221,138.650422095979,11.8788468616057));
#79283=CARTESIAN_POINT('Ctrl Pts',(4.83030185495524,138.631941871041,11.8834862280648));
#79284=CARTESIAN_POINT('Ctrl Pts',(4.829623758664,138.620267637226,11.886571061028));
#79285=CARTESIAN_POINT('Ctrl Pts',(4.82671483766814,138.570844130305,11.900287351417));
#79286=CARTESIAN_POINT('Ctrl Pts',(4.8244217778305,138.533494433918,11.9122888055571));
#79287=CARTESIAN_POINT('Ctrl Pts',(4.81600791076604,138.400372776943,11.9610460801033));
#79288=CARTESIAN_POINT('Ctrl Pts',(4.8097337224059,138.308042899344,12.0063431193744));
#79289=CARTESIAN_POINT('Ctrl Pts',(4.80067139355871,138.177597192873,12.0883323779925));
#79290=CARTESIAN_POINT('Ctrl Pts',(4.79770403475069,138.135466159805,12.1180241468914));
#79291=CARTESIAN_POINT('Ctrl Pts',(4.79377095516974,138.080285980148,12.1614446838187));
#79292=CARTESIAN_POINT('Ctrl Pts',(4.79273420937021,138.065809758149,12.173292085729));
#79293=CARTESIAN_POINT('Ctrl Pts',(4.7909753099417,138.041379689634,12.1940803928994));
#79294=CARTESIAN_POINT('Ctrl Pts',(4.79024780622353,138.031314284487,12.202886023247));
#79295=CARTESIAN_POINT('Ctrl Pts',(4.7887706684013,138.010966116866,12.2211858167205));
#79296=CARTESIAN_POINT('Ctrl Pts',(4.78802165158011,138.000695997261,12.2306920029107));
#79297=CARTESIAN_POINT('Ctrl Pts',(4.78611091541732,137.97463706906,12.2555159442617));
#79298=CARTESIAN_POINT('Ctrl Pts',(4.78495841017063,137.959054154115,12.2710452412685));
#79299=CARTESIAN_POINT('Ctrl Pts',(4.7777299298348,137.862392491039,12.3718186444322));
#79300=CARTESIAN_POINT('Ctrl Pts',(4.77210627988811,137.791493457466,12.4662224993563));
#79301=CARTESIAN_POINT('Ctrl Pts',(4.76416132558251,137.710099106485,12.6071632660803));
#79302=CARTESIAN_POINT('Ctrl Pts',(4.76194039249237,137.68935927512,12.647246194033));
#79303=CARTESIAN_POINT('Ctrl Pts',(4.75827661865235,137.65920000554,12.7127871428391));
#79304=CARTESIAN_POINT('Ctrl Pts',(4.75687890750066,137.648579165048,12.737661026311));
#79305=CARTESIAN_POINT('Ctrl Pts',(4.7548918269284,137.634824729027,12.7725177075315));
#79306=CARTESIAN_POINT('Ctrl Pts',(4.75433328109003,137.631099363174,12.7822624958746));
#79307=CARTESIAN_POINT('Ctrl Pts',(4.75336487447504,137.624888491528,12.799044633777));
#79308=CARTESIAN_POINT('Ctrl Pts',(4.7529579455227,137.622352099886,12.8060625531796));
#79309=CARTESIAN_POINT('Ctrl Pts',(4.75206988458404,137.616976987586,12.8212984444337));
#79310=CARTESIAN_POINT('Ctrl Pts',(4.75158774581658,137.61415778368,12.8295223960637));
#79311=CARTESIAN_POINT('Ctrl Pts',(4.75019804766149,137.606306518591,12.8531084672919));
#79312=CARTESIAN_POINT('Ctrl Pts',(4.74928110284224,137.601455625317,12.8685290850124));
#79313=CARTESIAN_POINT('Ctrl Pts',(4.74468326752112,137.578683589876,12.9453423946502));
#79314=CARTESIAN_POINT('Ctrl Pts',(4.74085350185027,137.564545861888,13.0077799023517));
#79315=CARTESIAN_POINT('Ctrl Pts',(4.73240862021616,137.542590011186,13.1463281796392));
#79316=CARTESIAN_POINT('Ctrl Pts',(4.72780130089799,137.536558490182,13.2225444839638));
#79317=CARTESIAN_POINT('Ctrl Pts',(4.72331126934335,137.53650014106,13.2992578962685));
#79318=CARTESIAN_POINT('Ctrl Pts',(4.7232895549327,137.5365,13.2996289488461));
#79319=CARTESIAN_POINT('Ctrl Pts',(4.72326784382709,137.5365,13.299999999986));
#79320=CARTESIAN_POINT('',(4.65354584395168,137.536500526148,13.298887278614));
#79321=CARTESIAN_POINT('Ctrl Pts',(4.65349091708139,137.5365,13.3000000000138));
#79322=CARTESIAN_POINT('Ctrl Pts',(4.65350929441382,137.5365,13.2996289660132));
#79323=CARTESIAN_POINT('Ctrl Pts',(4.65352766935275,137.5365001411,13.2992579299891));
#79324=CARTESIAN_POINT('Ctrl Pts',(4.65354604191487,137.536500423304,13.2988868920213));
#79325=CARTESIAN_POINT('Ctrl Pts',(4.65354602233856,137.536500423003,13.2988872873692));
#79326=CARTESIAN_POINT('Ctrl Pts',(4.6577293092493,137.536564655774,13.2144048882518));
#79327=CARTESIAN_POINT('Ctrl Pts',(4.66176523213553,137.543943858772,13.1300884198745));
#79328=CARTESIAN_POINT('Ctrl Pts',(4.66770202050596,137.564816053257,13.0112274796867));
#79329=CARTESIAN_POINT('Ctrl Pts',(4.66950433321345,137.572396927557,12.975821440743));
#79330=CARTESIAN_POINT('Ctrl Pts',(4.67255190081265,137.587027913655,12.9180445111731));
#79331=CARTESIAN_POINT('Ctrl Pts',(4.67376859434626,137.593317034569,12.8954965619373));
#79332=CARTESIAN_POINT('Ctrl Pts',(4.67553689863044,137.603019658087,12.8636797256772));
#79333=CARTESIAN_POINT('Ctrl Pts',(4.67606586182223,137.605990696879,12.8542786638995));
#79334=CARTESIAN_POINT('Ctrl Pts',(4.67699931657034,137.611345985791,12.8379107324697));
#79335=CARTESIAN_POINT('Ctrl Pts',(4.67740143162642,137.613688184537,12.8309306983713));
#79336=CARTESIAN_POINT('Ctrl Pts',(4.6782996574533,137.618996209603,12.8154992325445));
#79337=CARTESIAN_POINT('Ctrl Pts',(4.67879711645867,137.621986977745,12.8070572398695));
#79338=CARTESIAN_POINT('Ctrl Pts',(4.68031617372947,137.631279886708,12.7815719056368));
#79339=CARTESIAN_POINT('Ctrl Pts',(4.6813502497828,137.637821941617,12.7646185338567));
#79340=CARTESIAN_POINT('Ctrl Pts',(4.6884303602977,137.684183619342,12.6508298199644));
#79341=CARTESIAN_POINT('Ctrl Pts',(4.69484769726215,137.733979064281,12.5583903501883));
#79342=CARTESIAN_POINT('Ctrl Pts',(4.70406066107294,137.821184918616,12.4312810680816));
#79343=CARTESIAN_POINT('Ctrl Pts',(4.70697924740942,137.851210623,12.3919464916551));
#79344=CARTESIAN_POINT('Ctrl Pts',(4.71182447440425,137.905498477526,12.3278414899117));
#79345=CARTESIAN_POINT('Ctrl Pts',(4.71378379700898,137.928752374379,12.3022753113496));
#79346=CARTESIAN_POINT('Ctrl Pts',(4.71661303131404,137.964283281533,12.2658873165816));
#79347=CARTESIAN_POINT('Ctrl Pts',(4.71751175655903,137.97587024234,12.2544109637432));
#79348=CARTESIAN_POINT('Ctrl Pts',(4.71910470302774,137.996942031261,12.2342267436489));
#79349=CARTESIAN_POINT('Ctrl Pts',(4.71980204478394,138.00635438291,12.225445987874));
#79350=CARTESIAN_POINT('Ctrl Pts',(4.72129605731582,138.02692023061,12.2067614887341));
#79351=CARTESIAN_POINT('Ctrl Pts',(4.72209084117459,138.038111812014,12.1969017196732));
#79352=CARTESIAN_POINT('Ctrl Pts',(4.72426087409004,138.069343435545,12.1702234934595));
#79353=CARTESIAN_POINT('Ctrl Pts',(4.72562148158929,138.089687127381,12.1537682704418));
#79354=CARTESIAN_POINT('Ctrl Pts',(4.73274708444683,138.199989058206,12.0693392616625));
#79355=CARTESIAN_POINT('Ctrl Pts',(4.73812522945409,138.297131622474,12.0113882208182));
#79356=CARTESIAN_POINT('Ctrl Pts',(4.74573324193404,138.439060493645,11.9475887371679));
#79357=CARTESIAN_POINT('Ctrl Pts',(4.74784913313509,138.478905060962,11.9317423323137));
#79358=CARTESIAN_POINT('Ctrl Pts',(4.75135928007426,138.544086838964,11.9090796684693));
#79359=CARTESIAN_POINT('Ctrl Pts',(4.75271281234012,138.569012832597,11.9011554464974));
#79360=CARTESIAN_POINT('Ctrl Pts',(4.75464518845147,138.604003338899,11.8910555845466));
#79361=CARTESIAN_POINT('Ctrl Pts',(4.75519528672644,138.613899867883,11.8883115084047));
#79362=CARTESIAN_POINT('Ctrl Pts',(4.75615200229201,138.630978920424,11.8837689084596));
#79363=CARTESIAN_POINT('Ctrl Pts',(4.75655582279702,138.638147564674,11.8819203565725));
#79364=CARTESIAN_POINT('Ctrl Pts',(4.75744035672023,138.653756774579,11.878021337886));
#79365=CARTESIAN_POINT('Ctrl Pts',(4.75792211920961,138.662201649147,11.8759915895538));
#79366=CARTESIAN_POINT('Ctrl Pts',(4.75931779363978,138.68652271521,11.8703744684641));
#79367=CARTESIAN_POINT('Ctrl Pts',(4.76024126965751,138.702440909593,11.8669767232499));
#79368=CARTESIAN_POINT('Ctrl Pts',(4.7654736357832,138.791886269775,11.8494390852533));
#79369=CARTESIAN_POINT('Ctrl Pts',(4.76998707633885,138.86635306689,11.8406935610312));
#79370=CARTESIAN_POINT('Ctrl Pts',(4.78067379438162,139.043590360665,11.8335614827661));
#79371=CARTESIAN_POINT('Ctrl Pts',(4.78679874052828,139.146189003452,11.8402134983184));
#79372=CARTESIAN_POINT('Ctrl Pts',(4.79385500135757,139.269286943371,11.8613144146805));
#79373=CARTESIAN_POINT('Ctrl Pts',(4.79510233003266,139.291224833312,11.8655942535914));
#79374=CARTESIAN_POINT('Ctrl Pts',(4.7971056062786,139.326737720072,11.873370808738));
#79375=CARTESIAN_POINT('Ctrl Pts',(4.79787104900426,139.340375059701,11.8765628833789));
#79376=CARTESIAN_POINT('Ctrl Pts',(4.79934771716192,139.366807249459,11.883151431197));
#79377=CARTESIAN_POINT('Ctrl Pts',(4.80005954043639,139.379605936125,11.8865266984298));
#79378=CARTESIAN_POINT('Ctrl Pts',(4.8017403908532,139.409949977277,11.8949709135095));
#79379=CARTESIAN_POINT('Ctrl Pts',(4.80270429876016,139.427449893669,11.9001956045442));
#79380=CARTESIAN_POINT('Ctrl Pts',(4.80599205970899,139.487406210783,11.9193251593732));
#79381=CARTESIAN_POINT('Ctrl Pts',(4.80826406382799,139.529322388639,11.9348457612707));
#79382=CARTESIAN_POINT('Ctrl Pts',(4.8158739985949,139.669699711035,11.994264093138));
#79383=CARTESIAN_POINT('Ctrl Pts',(4.82096425383808,139.763985276689,12.0470958002338));
#79384=CARTESIAN_POINT('Ctrl Pts',(4.82840832789733,139.885746281297,12.134218201754));
#79385=CARTESIAN_POINT('Ctrl Pts',(4.83053567654524,139.918809352761,12.1600953947755));
#79386=CARTESIAN_POINT('Ctrl Pts',(4.83337846541901,139.959826218681,12.1951427279094));
#79387=CARTESIAN_POINT('Ctrl Pts',(4.83401688123966,139.968843916272,12.2030417468687));
#79388=CARTESIAN_POINT('Ctrl Pts',(4.83507781751693,139.983487947561,12.216190560888));
#79389=CARTESIAN_POINT('Ctrl Pts',(4.83549575378303,139.989171925473,12.2213757177941));
#79390=CARTESIAN_POINT('Ctrl Pts',(4.83635494859805,140.000677108576,12.2320386418503));
#79391=CARTESIAN_POINT('Ctrl Pts',(4.83679642533085,140.006494775698,12.2375196950466));
#79392=CARTESIAN_POINT('Ctrl Pts',(4.8379875998989,140.021951854619,12.2523232930375));
#79393=CARTESIAN_POINT('Ctrl Pts',(4.83874333923753,140.031508312428,12.2617309352858));
#79394=CARTESIAN_POINT('Ctrl Pts',(4.84367714058061,140.092403765029,12.3233486817743));
#79395=CARTESIAN_POINT('Ctrl Pts',(4.84807196708989,140.139888540211,12.3792143788359));
#79396=CARTESIAN_POINT('Ctrl Pts',(4.85700107141657,140.227165073143,12.4990453624152));
#79397=CARTESIAN_POINT('Ctrl Pts',(4.8615213544411,140.266613495803,12.5630100150866));
#79398=CARTESIAN_POINT('Ctrl Pts',(4.86850072466635,140.321352486862,12.669256205408));
#79399=CARTESIAN_POINT('Ctrl Pts',(4.87104763310839,140.339909781994,12.7097013625851));
#79400=CARTESIAN_POINT('Ctrl Pts',(4.87452737305845,140.363271775711,12.7674224993983));
#79401=CARTESIAN_POINT('Ctrl Pts',(4.8755115517479,140.36964503468,12.7840336765302));
#79402=CARTESIAN_POINT('Ctrl Pts',(4.87720637966401,140.380204129535,12.8131303461209));
#79403=CARTESIAN_POINT('Ctrl Pts',(4.87792150524246,140.384527186493,12.8255635082221));
#79404=CARTESIAN_POINT('Ctrl Pts',(4.87939537261687,140.393156505919,12.8515045709968));
#79405=CARTESIAN_POINT('Ctrl Pts',(4.88015315563447,140.397435419971,12.8650201544894));
#79406=CARTESIAN_POINT('Ctrl Pts',(4.88213449702556,140.40819654698,12.900809825447));
#79407=CARTESIAN_POINT('Ctrl Pts',(4.88334730157221,140.414346852789,12.9231799263664));
#79408=CARTESIAN_POINT('Ctrl Pts',(4.89014334604605,140.446214748924,13.0508955733023));
#79409=CARTESIAN_POINT('Ctrl Pts',(4.89535738076678,140.460693104425,13.1586935896334));
#79410=CARTESIAN_POINT('Ctrl Pts',(4.90306074918849,140.464248291956,13.3168378993344));
#79411=CARTESIAN_POINT('Ctrl Pts',(4.90549779740134,140.462830072721,13.3665901598664));
#79412=CARTESIAN_POINT('Ctrl Pts',(4.90946957942771,140.456604106806,13.4447763686312));
#79413=CARTESIAN_POINT('Ctrl Pts',(4.91094920990118,140.453485521771,13.4733071243042));
#79414=CARTESIAN_POINT('Ctrl Pts',(4.91303174597363,140.448067297232,13.5122405489863));
#79415=CARTESIAN_POINT('Ctrl Pts',(4.91359965026627,140.446489698711,13.5227386050876));
#79416=CARTESIAN_POINT('Ctrl Pts',(4.91457663704094,140.443610973675,13.5405724422096));
#79417=CARTESIAN_POINT('Ctrl Pts',(4.91498258233514,140.442367761664,13.5479172889239));
#79418=CARTESIAN_POINT('Ctrl Pts',(4.91585860534388,140.439586224405,13.5636209047145));
#79419=CARTESIAN_POINT('Ctrl Pts',(4.91632953283807,140.438031106115,13.5719761191759));
#79420=CARTESIAN_POINT('Ctrl Pts',(4.91766406165464,140.433454369699,13.5954282721577));
#79421=CARTESIAN_POINT('Ctrl Pts',(4.91853604874715,140.430267235034,13.6104913721952));
#79422=CARTESIAN_POINT('Ctrl Pts',(4.92432476240232,140.407791051954,13.7090164531306));
#79423=CARTESIAN_POINT('Ctrl Pts',(4.92951661196094,140.381444500495,13.7906927793563));
#79424=CARTESIAN_POINT('Ctrl Pts',(4.93852291305073,140.323217398582,13.9285049773874));
#79425=CARTESIAN_POINT('Ctrl Pts',(4.94234584116324,140.294488520076,13.9857283621063));
#79426=CARTESIAN_POINT('Ctrl Pts',(4.94842690466793,140.241535982016,14.075932747213));
#79427=CARTESIAN_POINT('Ctrl Pts',(4.95074559909251,140.219514517456,14.1101037028003));
#79428=CARTESIAN_POINT('Ctrl Pts',(4.95397595522907,140.186153025661,14.1574211898993));
#79429=CARTESIAN_POINT('Ctrl Pts',(4.95492950487781,140.175959261039,14.1713494990618));
#79430=CARTESIAN_POINT('Ctrl Pts',(4.95658955039651,140.157605403645,14.1955184499758));
#79431=CARTESIAN_POINT('Ctrl Pts',(4.95729999584974,140.149549959481,14.2058357858829));
#79432=CARTESIAN_POINT('Ctrl Pts',(4.9587809694609,140.132339777438,14.2272790394083));
#79433=CARTESIAN_POINT('Ctrl Pts',(4.95955026609241,140.123156946185,14.238380670513));
#79434=CARTESIAN_POINT('Ctrl Pts',(4.961602110347,140.098022015188,14.267870022555));
#79435=CARTESIAN_POINT('Ctrl Pts',(4.9628724049213,140.081772335783,14.2859986960734));
#79436=CARTESIAN_POINT('Ctrl Pts',(4.96880755549505,140.002746320679,14.3698560435872));
#79437=CARTESIAN_POINT('Ctrl Pts',(4.97323077851787,139.934386113374,14.430051520221));
#79438=CARTESIAN_POINT('Ctrl Pts',(4.98059408309831,139.811844899949,14.519187012722));
#79439=CARTESIAN_POINT('Ctrl Pts',(4.98353536043907,139.760641217656,14.5517720739616));
#79440=CARTESIAN_POINT('Ctrl Pts',(4.98821003081118,139.679381464709,14.5966533321517));
#79441=CARTESIAN_POINT('Ctrl Pts',(4.98986222412942,139.650691353748,14.6112854493932));
#79442=CARTESIAN_POINT('Ctrl Pts',(4.99214888547682,139.611545870546,14.6296487733508));
#79443=CARTESIAN_POINT('Ctrl Pts',(4.99273878963075,139.601495193339,14.6342255168632));
#79444=CARTESIAN_POINT('Ctrl Pts',(4.99374145690061,139.584518091223,14.6417255143741));
#79445=CARTESIAN_POINT('Ctrl Pts',(4.99415064172394,139.577618995616,14.6447100243752));
#79446=CARTESIAN_POINT('Ctrl Pts',(4.99501900857966,139.563047429241,14.6508807702581));
#79447=CARTESIAN_POINT('Ctrl Pts',(4.99547881388643,139.555370426522,14.6540550009044));
#79448=CARTESIAN_POINT('Ctrl Pts',(4.99677352348183,139.5338466528,14.6627406601994));
#79449=CARTESIAN_POINT('Ctrl Pts',(4.99761628450161,139.51994244611,14.6681060534114));
#79450=CARTESIAN_POINT('Ctrl Pts',(5.0038526295739,139.41761102848,14.705808752729));
#79451=CARTESIAN_POINT('Ctrl Pts',(5.0095836642536,139.326333119556,14.7297559339527));
#79452=CARTESIAN_POINT('Ctrl Pts',(5.01880232494781,139.174930702076,14.7542141032738));
#79453=CARTESIAN_POINT('Ctrl Pts',(5.02232880022041,139.11594429806,14.7601018052138));
#79454=CARTESIAN_POINT('Ctrl Pts',(5.02801402233816,139.018005018681,14.7639030859506));
#79455=CARTESIAN_POINT('Ctrl Pts',(5.03022326647168,138.979203811503,14.7638662279143));
#79456=CARTESIAN_POINT('Ctrl Pts',(5.03333257655306,138.923477506688,14.7615967319414));
#79457=CARTESIAN_POINT('Ctrl Pts',(5.03427031242056,138.90652063568,14.7606102633936));
#79458=CARTESIAN_POINT('Ctrl Pts',(5.03591262208634,138.876566243085,14.7583438539825));
#79459=CARTESIAN_POINT('Ctrl Pts',(5.03662087629769,138.863561713782,14.7571847165865));
#79460=CARTESIAN_POINT('Ctrl Pts',(5.03810674242522,138.83610562449,14.7543666754639));
#79461=CARTESIAN_POINT('Ctrl Pts',(5.03888296666831,138.821659724293,14.752666017947));
#79462=CARTESIAN_POINT('Ctrl Pts',(5.04097729194917,138.782428296083,14.747453402945));
#79463=CARTESIAN_POINT('Ctrl Pts',(5.04228219856684,138.757703187908,14.743520401952));
#79464=CARTESIAN_POINT('Ctrl Pts',(5.04946532204629,138.620400192299,14.718052248975));
#79465=CARTESIAN_POINT('Ctrl Pts',(5.05493407459768,138.510559260962,14.6839859156849));
#79466=CARTESIAN_POINT('Ctrl Pts',(5.06265286310582,138.366234640612,14.6198672128381));
#79467=CARTESIAN_POINT('Ctrl Pts',(5.06478975637915,138.327457004694,14.6005358620952));
#79468=CARTESIAN_POINT('Ctrl Pts',(5.06833045295634,138.266578987038,14.5667355480619));
#79469=CARTESIAN_POINT('Ctrl Pts',(5.06969265011079,138.243912509433,14.5533382939366));
#79470=CARTESIAN_POINT('Ctrl Pts',(5.07163537463751,138.212903160918,14.5338625515269));
#79471=CARTESIAN_POINT('Ctrl Pts',(5.07218674618762,138.204243578797,14.528295541012));
#79472=CARTESIAN_POINT('Ctrl Pts',(5.07314489350277,138.18945617945,14.5185671179001));
#79473=CARTESIAN_POINT('Ctrl Pts',(5.07354884717647,138.183300029537,14.5144497776335));
#79474=CARTESIAN_POINT('Ctrl Pts',(5.07443269150977,138.170004399232,14.5054106098516));
#79475=CARTESIAN_POINT('Ctrl Pts',(5.07491361493358,138.16287733258,14.5004720186524));
#79476=CARTESIAN_POINT('Ctrl Pts',(5.07630450722704,138.142555661318,14.486121467005));
#79477=CARTESIAN_POINT('Ctrl Pts',(5.07722394552476,138.129473323293,14.4765535217626));
#79478=CARTESIAN_POINT('Ctrl Pts',(5.08190186572212,138.064495102423,14.4273537908969));
#79479=CARTESIAN_POINT('Ctrl Pts',(5.08581549023863,138.01513705013,14.3844997577729));
#79480=CARTESIAN_POINT('Ctrl Pts',(5.0942867185469,137.915306700359,14.2853717699152));
#79481=CARTESIAN_POINT('Ctrl Pts',(5.09883474597897,137.865986216653,14.2281871016063));
#79482=CARTESIAN_POINT('Ctrl Pts',(5.10595098669164,137.793892199592,14.1302245870076));
#79483=CARTESIAN_POINT('Ctrl Pts',(5.10860223332788,137.768271521638,14.0917161676484));
#79484=CARTESIAN_POINT('Ctrl Pts',(5.11219468617073,137.735256992552,14.036601609092));
#79485=CARTESIAN_POINT('Ctrl Pts',(5.11319186334254,137.726285197964,14.0209767328904));
#79486=CARTESIAN_POINT('Ctrl Pts',(5.11490159218869,137.711245108907,13.9936261456993));
#79487=CARTESIAN_POINT('Ctrl Pts',(5.11561884639264,137.705042881322,13.9819768882044));
#79488=CARTESIAN_POINT('Ctrl Pts',(5.11709049190248,137.692545861232,13.9577191389076));
#79489=CARTESIAN_POINT('Ctrl Pts',(5.11784403035187,137.686273891123,13.94510039557));
#79490=CARTESIAN_POINT('Ctrl Pts',(5.11979932245047,137.670344496966,13.9118554631895));
#79491=CARTESIAN_POINT('Ctrl Pts',(5.12099085694664,137.660984394251,13.8910906408747));
#79492=CARTESIAN_POINT('Ctrl Pts',(5.12794340021902,137.608572669799,13.7671768538486));
#79493=CARTESIAN_POINT('Ctrl Pts',(5.13330636907962,137.57696824617,13.6595921755099));
#79494=CARTESIAN_POINT('Ctrl Pts',(5.14218297669775,137.54592361668,13.4801235496561));
#79495=CARTESIAN_POINT('Ctrl Pts',(5.14564447161847,137.538947345914,13.410026280976));
#79496=CARTESIAN_POINT('Ctrl Pts',(5.15002837370352,137.536679592768,13.3264741820039));
#79497=CARTESIAN_POINT('Ctrl Pts',(5.15073066744659,137.5365,13.3132371636019));
#79498=CARTESIAN_POINT('Ctrl Pts',(5.15144231116594,137.5365,13.3));
#79499=CARTESIAN_POINT('Origin',(4.2,139.,13.3));
#79500=CARTESIAN_POINT('',(5.72391728548022,137.5365,13.299999999962));
#79501=CARTESIAN_POINT('',(5.65336626804119,137.5365,13.3000000000336));
#79502=CARTESIAN_POINT('',(4.2,137.5365,13.3));
#79503=CARTESIAN_POINT('',(5.2255072336721,137.536499824611,13.2997577413145));
#79504=CARTESIAN_POINT('Ctrl Pts',(5.72391728548022,137.5365,13.299999999962));
#79505=CARTESIAN_POINT('Ctrl Pts',(5.72389637822813,137.5365,13.3004283951292));
#79506=CARTESIAN_POINT('Ctrl Pts',(5.72387547249502,137.536500188098,13.3008567940772));
#79507=CARTESIAN_POINT('Ctrl Pts',(5.71865265859192,137.536594181926,13.4078908979809));
#79508=CARTESIAN_POINT('Ctrl Pts',(5.7135925703568,137.548335533245,13.5141545643487));
#79509=CARTESIAN_POINT('Ctrl Pts',(5.70723738865168,137.574864658269,13.6332564662892));
#79510=CARTESIAN_POINT('Ctrl Pts',(5.70642300759539,137.57845946586,13.648271571164));
#79511=CARTESIAN_POINT('Ctrl Pts',(5.70513895596488,137.584409563309,13.671495397304));
#79512=CARTESIAN_POINT('Ctrl Pts',(5.70467797229086,137.586600386487,13.6797454935331));
#79513=CARTESIAN_POINT('Ctrl Pts',(5.70380404553555,137.590851812169,13.6952086850735));
#79514=CARTESIAN_POINT('Ctrl Pts',(5.70339200516247,137.592895891053,13.7024258159171));
#79515=CARTESIAN_POINT('Ctrl Pts',(5.70238346454748,137.597996370207,13.7199202726893));
#79516=CARTESIAN_POINT('Ctrl Pts',(5.70178381971873,137.601110374666,13.7301802128068));
#79517=CARTESIAN_POINT('Ctrl Pts',(5.69952978702925,137.613128469687,13.7682661235052));
#79518=CARTESIAN_POINT('Ctrl Pts',(5.69784081637494,137.622751992439,13.7958563424438));
#79519=CARTESIAN_POINT('Ctrl Pts',(5.69312465437233,137.651478924373,13.8709113489526));
#79520=CARTESIAN_POINT('Ctrl Pts',(5.6900492266378,137.672255226099,13.9176910625191));
#79521=CARTESIAN_POINT('Ctrl Pts',(5.68060372021012,137.743319690697,14.0574622007059));
#79522=CARTESIAN_POINT('Ctrl Pts',(5.67426820867668,137.801267145866,14.1461915252801));
#79523=CARTESIAN_POINT('Ctrl Pts',(5.66694802020969,137.883214985727,14.2461389450492));
#79524=CARTESIAN_POINT('Ctrl Pts',(5.66563009526459,137.898596194119,14.2640007357975));
#79525=CARTESIAN_POINT('Ctrl Pts',(5.66354012923289,137.924000012934,14.2920993247205));
#79526=CARTESIAN_POINT('Ctrl Pts',(5.66275711945597,137.933752684019,14.302573550367));
#79527=CARTESIAN_POINT('Ctrl Pts',(5.6612625736126,137.952816984269,14.3224554355365));
#79528=CARTESIAN_POINT('Ctrl Pts',(5.66055016371869,137.962105641241,14.3318830854263));
#79529=CARTESIAN_POINT('Ctrl Pts',(5.65889193409669,137.984191531386,14.3536994780832));
#79530=CARTESIAN_POINT('Ctrl Pts',(5.6579507193345,137.997089696933,14.36598329992));
#79531=CARTESIAN_POINT('Ctrl Pts',(5.65471068725743,138.042709486387,14.4078690426697));
#79532=CARTESIAN_POINT('Ctrl Pts',(5.65246288138475,138.076544003566,14.4362255112131));
#79533=CARTESIAN_POINT('Ctrl Pts',(5.64656531863272,138.170277436183,14.5078256707518));
#79534=CARTESIAN_POINT('Ctrl Pts',(5.64300302555776,138.232253012377,14.5481375679306));
#79535=CARTESIAN_POINT('Ctrl Pts',(5.63602132383873,138.358058514244,14.617037904631));
#79536=CARTESIAN_POINT('Ctrl Pts',(5.632612065005,138.42141378614,14.646073537052));
#79537=CARTESIAN_POINT('Ctrl Pts',(5.62815343091723,138.501743713544,14.6761667309332));
#79538=CARTESIAN_POINT('Ctrl Pts',(5.62730111691074,138.51699246217,14.681592513932));
#79539=CARTESIAN_POINT('Ctrl Pts',(5.62596970057426,138.540570722669,14.6895440508814));
#79540=CARTESIAN_POINT('Ctrl Pts',(5.62550031015406,138.548838434775,14.6922503957847));
#79541=CARTESIAN_POINT('Ctrl Pts',(5.62462020890355,138.564242986697,14.6971412873433));
#79542=CARTESIAN_POINT('Ctrl Pts',(5.62421058799822,138.571373137075,14.6993451879723));
#79543=CARTESIAN_POINT('Ctrl Pts',(5.62322113619387,138.588507002627,14.7044979638206));
#79544=CARTESIAN_POINT('Ctrl Pts',(5.62263846368407,138.598525820858,14.7073945743019));
#79545=CARTESIAN_POINT('Ctrl Pts',(5.62052769670455,138.634604237196,14.7174088821815));
#79546=CARTESIAN_POINT('Ctrl Pts',(5.61897022514301,138.660827578822,14.7239114771334));
#79547=CARTESIAN_POINT('Ctrl Pts',(5.6147551592352,138.731204470769,14.7393085104492));
#79548=CARTESIAN_POINT('Ctrl Pts',(5.61205950614645,138.775613650252,14.7468968252568));
#79549=CARTESIAN_POINT('Ctrl Pts',(5.60226436306562,138.937188858354,14.7668876046108));
#79550=CARTESIAN_POINT('Ctrl Pts',(5.59516570191898,139.055417762657,14.7671884546904));
#79551=CARTESIAN_POINT('Ctrl Pts',(5.5872746105708,139.194233374073,14.7507199658923));
#79552=CARTESIAN_POINT('Ctrl Pts',(5.58604909393427,139.215992171165,14.7476403140392));
#79553=CARTESIAN_POINT('Ctrl Pts',(5.58406836846119,139.251477418635,14.7417999329865));
#79554=CARTESIAN_POINT('Ctrl Pts',(5.58330417193893,139.265247633504,14.7393302785854));
#79555=CARTESIAN_POINT('Ctrl Pts',(5.58182146426441,139.292111278597,14.7341137211655));
#79556=CARTESIAN_POINT('Ctrl Pts',(5.58110249043369,139.305206599046,14.7313839850039));
#79557=CARTESIAN_POINT('Ctrl Pts',(5.57939068850764,139.336536138022,14.7244037916816));
#79558=CARTESIAN_POINT('Ctrl Pts',(5.57840340179084,139.354730022388,14.7199821785688));
#79559=CARTESIAN_POINT('Ctrl Pts',(5.57473089708195,139.422787296265,14.7020526395447));
#79560=CARTESIAN_POINT('Ctrl Pts',(5.57211827514126,139.472010574343,14.6862566088054));
#79561=CARTESIAN_POINT('Ctrl Pts',(5.56442898639115,139.616893465292,14.6311480523088));
#79562=CARTESIAN_POINT('Ctrl Pts',(5.55954090568322,139.709318528831,14.5842811928146));
#79563=CARTESIAN_POINT('Ctrl Pts',(5.55246840493619,139.828257901125,14.5071851007473));
#79564=CARTESIAN_POINT('Ctrl Pts',(5.55051524489856,139.859646042782,14.4850380898172));
#79565=CARTESIAN_POINT('Ctrl Pts',(5.54785935113477,139.899654459646,14.4543821905583));
#79566=CARTESIAN_POINT('Ctrl Pts',(5.54721996416373,139.90909377802,14.4469633266888));
#79567=CARTESIAN_POINT('Ctrl Pts',(5.54619721030052,139.923864333395,14.435057476911));
#79568=CARTESIAN_POINT('Ctrl Pts',(5.54581903187127,139.929256819687,14.4306469569978));
#79569=CARTESIAN_POINT('Ctrl Pts',(5.54500939844907,139.940648532755,14.4211931198686));
#79570=CARTESIAN_POINT('Ctrl Pts',(5.54457719797828,139.946639097534,14.4161398148752));
#79571=CARTESIAN_POINT('Ctrl Pts',(5.54344548138047,139.962101216796,14.4028828169579));
#79572=CARTESIAN_POINT('Ctrl Pts',(5.54274092982271,139.971508354934,14.3946052959675));
#79573=CARTESIAN_POINT('Ctrl Pts',(5.53924676317011,140.017168473478,14.3533758222069));
#79574=CARTESIAN_POINT('Ctrl Pts',(5.53635880439322,140.051854881851,14.3187408150879));
#79575=CARTESIAN_POINT('Ctrl Pts',(5.52987984334206,140.124641088656,14.2383753653396));
#79576=CARTESIAN_POINT('Ctrl Pts',(5.52627752556616,140.161824111303,14.1919252695472));
#79577=CARTESIAN_POINT('Ctrl Pts',(5.51797867341239,140.241635265008,14.078732269978));
#79578=CARTESIAN_POINT('Ctrl Pts',(5.51333182801939,140.281885954351,14.010530343963));
#79579=CARTESIAN_POINT('Ctrl Pts',(5.50770395810861,140.325550132345,13.9206323577577));
#79580=CARTESIAN_POINT('Ctrl Pts',(5.50654235398232,140.334264689012,13.9016689121472));
#79581=CARTESIAN_POINT('Ctrl Pts',(5.50463715044389,140.348051952222,13.8698927913858));
#79582=CARTESIAN_POINT('Ctrl Pts',(5.5038858529879,140.353354423861,13.8571837050474));
#79583=CARTESIAN_POINT('Ctrl Pts',(5.50240882193819,140.363506394877,13.8318508922021));
#79584=CARTESIAN_POINT('Ctrl Pts',(5.50168294448817,140.36836186416,13.8192310525399));
#79585=CARTESIAN_POINT('Ctrl Pts',(5.49992148939154,140.379808536156,13.7882037079661));
#79586=CARTESIAN_POINT('Ctrl Pts',(5.49889233365343,140.386207197057,13.7697276993828));
#79587=CARTESIAN_POINT('Ctrl Pts',(5.4947398886582,140.410790720533,13.6938601324959));
#79588=CARTESIAN_POINT('Ctrl Pts',(5.49171847632477,140.42579725201,13.6354987578867));
#79589=CARTESIAN_POINT('Ctrl Pts',(5.48582101902314,140.448412099927,13.5178998681133));
#79590=CARTESIAN_POINT('Ctrl Pts',(5.48294889062536,140.456077893386,13.458792970542));
#79591=CARTESIAN_POINT('Ctrl Pts',(5.47693737706805,140.464450500837,13.3357848690572));
#79592=CARTESIAN_POINT('Ctrl Pts',(5.47379931191519,140.464619094939,13.2719761437451));
#79593=CARTESIAN_POINT('Ctrl Pts',(5.46964664275004,140.459616931282,13.1922426392474));
#79594=CARTESIAN_POINT('Ctrl Pts',(5.4687958546543,140.458338558129,13.1761378072726));
#79595=CARTESIAN_POINT('Ctrl Pts',(5.46746642633736,140.455962839974,13.151406602761));
#79596=CARTESIAN_POINT('Ctrl Pts',(5.46699746099894,140.455054733,13.1427629007822));
#79597=CARTESIAN_POINT('Ctrl Pts',(5.46611779991708,140.453223864314,13.1267131090235));
#79598=CARTESIAN_POINT('Ctrl Pts',(5.46570818692665,140.452321361576,13.1193052287706));
#79599=CARTESIAN_POINT('Ctrl Pts',(5.46471835710986,140.450020992145,13.101555346394));
#79600=CARTESIAN_POINT('Ctrl Pts',(5.46413529008978,140.448569103508,13.0912209359819));
#79601=CARTESIAN_POINT('Ctrl Pts',(5.46202111818797,140.442954835541,13.0541419545273));
#79602=CARTESIAN_POINT('Ctrl Pts',(5.46046051416501,140.438161426173,13.0274997788727));
#79603=CARTESIAN_POINT('Ctrl Pts',(5.45623386065201,140.423404113051,12.9567896154052));
#79604=CARTESIAN_POINT('Ctrl Pts',(5.45352952400148,140.412133945916,12.913024566162));
#79605=CARTESIAN_POINT('Ctrl Pts',(5.44374294222581,140.364326547212,12.7575526153661));
#79606=CARTESIAN_POINT('Ctrl Pts',(5.4366625875207,140.31639024624,12.6497989908346));
#79607=CARTESIAN_POINT('Ctrl Pts',(5.42878468025893,140.244777001058,12.5300343004235));
#79608=CARTESIAN_POINT('Ctrl Pts',(5.42755661454506,140.233052939967,12.511395230575));
#79609=CARTESIAN_POINT('Ctrl Pts',(5.42557288282212,140.21319406304,12.4813496792768));
#79610=CARTESIAN_POINT('Ctrl Pts',(5.42480817596103,140.205308494417,12.4697833809009));
#79611=CARTESIAN_POINT('Ctrl Pts',(5.42332521182643,140.189568372943,12.4473933414201));
#79612=CARTESIAN_POINT('Ctrl Pts',(5.42260647974065,140.181729035038,12.436560637797));
#79613=CARTESIAN_POINT('Ctrl Pts',(5.42089644896204,140.162577485868,12.4108457868462));
#79614=CARTESIAN_POINT('Ctrl Pts',(5.41991066083533,140.151126334015,12.3960697866276));
#79615=CARTESIAN_POINT('Ctrl Pts',(5.4162533701934,140.1071431454,12.3415078546338));
#79616=CARTESIAN_POINT('Ctrl Pts',(5.41365362948447,140.072804949657,12.3032235283665));
#79617=CARTESIAN_POINT('Ctrl Pts',(5.40604299584359,139.964521200469,12.1945893362171));
#79618=CARTESIAN_POINT('Ctrl Pts',(5.40121505470921,139.885172302452,12.1300844713586));
#79619=CARTESIAN_POINT('Ctrl Pts',(5.39415212338304,139.766427698706,12.0526005056986));
#79620=CARTESIAN_POINT('Ctrl Pts',(5.39213093264031,139.732218250109,12.0322173358668));
#79621=CARTESIAN_POINT('Ctrl Pts',(5.38939545877631,139.686553104341,12.0074736492702));
#79622=CARTESIAN_POINT('Ctrl Pts',(5.38874939080079,139.67581168462,12.001825096474));
#79623=CARTESIAN_POINT('Ctrl Pts',(5.38771861103018,139.658774511172,11.9931345670738));
#79624=CARTESIAN_POINT('Ctrl Pts',(5.38733923226514,139.652524859342,11.9900028930779));
#79625=CARTESIAN_POINT('Ctrl Pts',(5.38653008246416,139.639247501558,11.9834682499054));
#79626=CARTESIAN_POINT('Ctrl Pts',(5.38609960638404,139.632214590793,11.980076547275));
#79627=CARTESIAN_POINT('Ctrl Pts',(5.38497770191796,139.61395370643,11.9714494469709));
#79628=CARTESIAN_POINT('Ctrl Pts',(5.38428139150684,139.602685956641,11.9663001303511));
#79629=CARTESIAN_POINT('Ctrl Pts',(5.38092214719258,139.54856011565,11.9423907878854));
#79630=CARTESIAN_POINT('Ctrl Pts',(5.37816948083471,139.504887055656,11.9255512638113));
#79631=CARTESIAN_POINT('Ctrl Pts',(5.36859128213735,139.352522387501,11.875044805052));
#79632=CARTESIAN_POINT('Ctrl Pts',(5.36164375114044,139.240737436001,11.851959883935));
#79633=CARTESIAN_POINT('Ctrl Pts',(5.35291289419451,139.090464055092,11.8388280316334));
#79634=CARTESIAN_POINT('Ctrl Pts',(5.35080417091939,139.053412249684,11.8370048736925));
#79635=CARTESIAN_POINT('Ctrl Pts',(5.34780341457363,138.99954809044,11.8364038565968));
#79636=CARTESIAN_POINT('Ctrl Pts',(5.34687747424622,138.982765000258,11.8365052569061));
#79637=CARTESIAN_POINT('Ctrl Pts',(5.34524445508551,138.952885706068,11.8371998679991));
#79638=CARTESIAN_POINT('Ctrl Pts',(5.34453395360437,138.939788955931,11.8376803945055));
#79639=CARTESIAN_POINT('Ctrl Pts',(5.3430317626913,138.911902479224,11.8390788530151));
#79640=CARTESIAN_POINT('Ctrl Pts',(5.34224167617368,138.897116613836,11.8400456166482));
#79641=CARTESIAN_POINT('Ctrl Pts',(5.34007816415281,138.856326418779,11.8433354338352));
#79642=CARTESIAN_POINT('Ctrl Pts',(5.33871940407466,138.830365124708,11.8461300356354));
#79643=CARTESIAN_POINT('Ctrl Pts',(5.3356780056225,138.771648982735,11.8540448533916));
#79644=CARTESIAN_POINT('Ctrl Pts',(5.33400772487917,138.738965258159,11.8595863411916));
#79645=CARTESIAN_POINT('Ctrl Pts',(5.32787996588602,138.618292921139,11.8842889232365));
#79646=CARTESIAN_POINT('Ctrl Pts',(5.32358549382512,138.531946212759,11.9104448448433));
#79647=CARTESIAN_POINT('Ctrl Pts',(5.31652840601565,138.399012477598,11.9645201713861));
#79648=CARTESIAN_POINT('Ctrl Pts',(5.31385344278118,138.350620067362,11.9873701649532));
#79649=CARTESIAN_POINT('Ctrl Pts',(5.31036447819183,138.292185530774,12.0189851317788));
#79650=CARTESIAN_POINT('Ctrl Pts',(5.30967577803063,138.280862874708,12.0253070222855));
#79651=CARTESIAN_POINT('Ctrl Pts',(5.30855135615362,138.262753915427,12.0357360435736));
#79652=CARTESIAN_POINT('Ctrl Pts',(5.30812129578216,138.255914162491,12.0397494689021));
#79653=CARTESIAN_POINT('Ctrl Pts',(5.30725880344192,138.242378267333,12.0478406557384));
#79654=CARTESIAN_POINT('Ctrl Pts',(5.30682645844377,138.235681622389,12.0519170203705));
#79655=CARTESIAN_POINT('Ctrl Pts',(5.30569398860872,138.218358540849,12.0626535824364));
#79656=CARTESIAN_POINT('Ctrl Pts',(5.30498881718051,138.207784566565,12.069396809259));
#79657=CARTESIAN_POINT('Ctrl Pts',(5.30148438581034,138.156194204514,12.1032374464806));
#79658=CARTESIAN_POINT('Ctrl Pts',(5.29858611670499,138.116477271433,12.1322518993748));
#79659=CARTESIAN_POINT('Ctrl Pts',(5.29210541126258,138.032240467435,12.2005502924573));
#79660=CARTESIAN_POINT('Ctrl Pts',(5.28851227052994,137.988494315543,12.2406584725215));
#79661=CARTESIAN_POINT('Ctrl Pts',(5.28022459515594,137.892405800322,12.3401501579366));
#79662=CARTESIAN_POINT('Ctrl Pts',(5.27557990580273,137.842197838869,12.4013489706316));
#79663=CARTESIAN_POINT('Ctrl Pts',(5.26995414774073,137.785286932719,12.4834586694853));
#79664=CARTESIAN_POINT('Ctrl Pts',(5.2687926787047,137.773769005332,12.5008597173924));
#79665=CARTESIAN_POINT('Ctrl Pts',(5.26688760417105,137.755273607153,12.5301441245525));
#79666=CARTESIAN_POINT('Ctrl Pts',(5.26613630418817,137.748085057403,12.5418899442028));
#79667=CARTESIAN_POINT('Ctrl Pts',(5.26465920006158,137.734168031286,12.5653677631145));
#79668=CARTESIAN_POINT('Ctrl Pts',(5.26393325316231,137.727434281331,12.5770950235596));
#79669=CARTESIAN_POINT('Ctrl Pts',(5.26217150526856,137.711362780758,12.606005229778));
#79670=CARTESIAN_POINT('Ctrl Pts',(5.26114212995328,137.702204909271,12.6232854558685));
#79671=CARTESIAN_POINT('Ctrl Pts',(5.25698723001979,137.666258370454,12.6945293134945));
#79672=CARTESIAN_POINT('Ctrl Pts',(5.2539637372614,137.64246644401,12.7499408288739));
#79673=CARTESIAN_POINT('Ctrl Pts',(5.24709262408483,137.595432626154,12.8813025273928));
#79674=CARTESIAN_POINT('Ctrl Pts',(5.24330052769944,137.574818391967,12.9579853109963));
#79675=CARTESIAN_POINT('Ctrl Pts',(5.23802369550025,137.555506771268,13.0632672224454));
#79676=CARTESIAN_POINT('Ctrl Pts',(5.23664098441709,137.551275932362,13.090711779619));
#79677=CARTESIAN_POINT('Ctrl Pts',(5.23386176523994,137.544474589783,13.1450567819482));
#79678=CARTESIAN_POINT('Ctrl Pts',(5.23246718569157,137.541863418749,13.1719407837177));
#79679=CARTESIAN_POINT('Ctrl Pts',(5.23047084162199,137.539259359563,13.2095390088446));
#79680=CARTESIAN_POINT('Ctrl Pts',(5.22989933575708,137.53863788567,13.2202054712121));
#79681=CARTESIAN_POINT('Ctrl Pts',(5.22892328871679,137.537785449126,13.2382335798347));
#79682=CARTESIAN_POINT('Ctrl Pts',(5.22852203532409,137.537493159396,13.2455920639323));
#79683=CARTESIAN_POINT('Ctrl Pts',(5.22771005788807,137.537017846487,13.2603699195707));
#79684=CARTESIAN_POINT('Ctrl Pts',(5.2272993791108,137.536835702114,13.2677888646555));
#79685=CARTESIAN_POINT('Ctrl Pts',(5.22642976870488,137.536571363474,13.2833912809813));
#79686=CARTESIAN_POINT('Ctrl Pts',(5.22597023111713,137.53650137286,13.2915746869978));
#79687=CARTESIAN_POINT('Ctrl Pts',(5.22550755435867,137.536500019999,13.2997580565886));
#79688=CARTESIAN_POINT('Ctrl Pts',(5.22550757110334,137.536500020048,13.2997577604254));
#79689=CARTESIAN_POINT('Ctrl Pts',(5.22550300580094,137.536500006683,13.2998385069991));
#79690=CARTESIAN_POINT('Ctrl Pts',(5.22549844019539,137.5365,13.2999192535242));
#79691=CARTESIAN_POINT('Ctrl Pts',(5.22549387428705,137.5365,13.2999999999999));
#79692=CARTESIAN_POINT('',(5.65328936190197,137.536500632965,13.3012892780789));
#79693=CARTESIAN_POINT('Ctrl Pts',(5.15144231116594,137.5365,13.3));
#79694=CARTESIAN_POINT('Ctrl Pts',(5.15144646621951,137.5365,13.2999227125564));
#79695=CARTESIAN_POINT('Ctrl Pts',(5.15145062163286,137.536500006051,13.29984542511));
#79696=CARTESIAN_POINT('Ctrl Pts',(5.15188347220723,137.536501281478,13.2917952796205));
#79697=CARTESIAN_POINT('Ctrl Pts',(5.15231554190402,137.536567696437,13.2838227555621));
#79698=CARTESIAN_POINT('Ctrl Pts',(5.15317263650352,137.536826449736,13.26814344612));
#79699=CARTESIAN_POINT('Ctrl Pts',(5.15359743401917,137.537014548003,13.2604369174702));
#79700=CARTESIAN_POINT('Ctrl Pts',(5.1546951210923,137.537653110221,13.2406760253341));
#79701=CARTESIAN_POINT('Ctrl Pts',(5.15537256982121,137.538191741659,13.2286252396572));
#79702=CARTESIAN_POINT('Ctrl Pts',(5.15849059953924,137.541325323637,13.1737379114092));
#79703=CARTESIAN_POINT('Ctrl Pts',(5.16100682102238,137.545654579616,13.1310244124952));
#79704=CARTESIAN_POINT('Ctrl Pts',(5.17040674743905,137.568476826116,12.9747106951274));
#79705=CARTESIAN_POINT('Ctrl Pts',(5.17745000925033,137.598472760067,12.8631954233111));
#79706=CARTESIAN_POINT('Ctrl Pts',(5.18635965703472,137.655493181044,12.7206821770838));
#79707=CARTESIAN_POINT('Ctrl Pts',(5.18854988645136,137.671161592884,12.6855924882341));
#79708=CARTESIAN_POINT('Ctrl Pts',(5.19165583146573,137.69583001922,12.6357187467277));
#79709=CARTESIAN_POINT('Ctrl Pts',(5.19260796013722,137.703738527365,12.620415455939));
#79710=CARTESIAN_POINT('Ctrl Pts',(5.19426897269919,137.718146201342,12.5937030700346));
#79711=CARTESIAN_POINT('Ctrl Pts',(5.19498173743427,137.724532062223,12.5822353660219));
#79712=CARTESIAN_POINT('Ctrl Pts',(5.1964587349886,137.738187621774,12.5584706478231));
#79713=CARTESIAN_POINT('Ctrl Pts',(5.19722187964384,137.745484844507,12.5461910041623));
#79714=CARTESIAN_POINT('Ctrl Pts',(5.19923606196109,137.765380514118,12.5138002443835));
#79715=CARTESIAN_POINT('Ctrl Pts',(5.20047565704583,137.778290522975,12.4938850162607));
#79716=CARTESIAN_POINT('Ctrl Pts',(5.20546860748793,137.832913404767,12.4139512832592));
#79717=CARTESIAN_POINT('Ctrl Pts',(5.20907482337719,137.878611397436,12.3567808620436));
#79718=CARTESIAN_POINT('Ctrl Pts',(5.21668441351769,137.984936661586,12.2424690942639));
#79719=CARTESIAN_POINT('Ctrl Pts',(5.22066134704973,138.046548021553,12.1866030186736));
#79720=CARTESIAN_POINT('Ctrl Pts',(5.2263257844008,138.135612605281,12.1186840919646));
#79721=CARTESIAN_POINT('Ctrl Pts',(5.22781859081503,138.159183010634,12.1017932440421));
#79722=CARTESIAN_POINT('Ctrl Pts',(5.2299308936223,138.192311079561,12.0795122212282));
#79723=CARTESIAN_POINT('Ctrl Pts',(5.23051517800192,138.201452046782,12.0735119395835));
#79724=CARTESIAN_POINT('Ctrl Pts',(5.23151122929005,138.21697366425,12.0635703664218));
#79725=CARTESIAN_POINT('Ctrl Pts',(5.23191953131606,138.223319102512,12.0595745634491));
#79726=CARTESIAN_POINT('Ctrl Pts',(5.23278959702834,138.236797106945,12.0512312615137));
#79727=CARTESIAN_POINT('Ctrl Pts',(5.23325203873197,138.243936530905,12.0468958375753));
#79728=CARTESIAN_POINT('Ctrl Pts',(5.23456188055164,138.264104774722,12.0348837422996));
#79729=CARTESIAN_POINT('Ctrl Pts',(5.23541741902444,138.277215704362,12.0273477483613));
#79730=CARTESIAN_POINT('Ctrl Pts',(5.23740732974182,138.307633005543,12.0104859013627));
#79731=CARTESIAN_POINT('Ctrl Pts',(5.23854815078499,138.325015101979,12.0013029643975));
#79732=CARTESIAN_POINT('Ctrl Pts',(5.242593073207,138.386651087998,11.9703124169934));
#79733=CARTESIAN_POINT('Ctrl Pts',(5.24555540226669,138.431816565312,11.9503951956846));
#79734=CARTESIAN_POINT('Ctrl Pts',(5.25510285665952,138.579914644636,11.893840210316));
#79735=CARTESIAN_POINT('Ctrl Pts',(5.26166103881786,138.685985989613,11.8664173976163));
#79736=CARTESIAN_POINT('Ctrl Pts',(5.2691492785385,138.817003073326,11.8478023457227));
#79737=CARTESIAN_POINT('Ctrl Pts',(5.27044022770045,138.839948867676,11.8450946343882));
#79738=CARTESIAN_POINT('Ctrl Pts',(5.27249505040638,138.8770443951,11.8416054801674));
#79739=CARTESIAN_POINT('Ctrl Pts',(5.27326935387441,138.891157501101,11.8404843315371));
#79740=CARTESIAN_POINT('Ctrl Pts',(5.27475165734572,138.918427133229,11.8387157842537));
#79741=CARTESIAN_POINT('Ctrl Pts',(5.27546044684804,138.93158044096,11.8380408790497));
#79742=CARTESIAN_POINT('Ctrl Pts',(5.27711649088458,138.962567728502,11.8368700304699));
#79743=CARTESIAN_POINT('Ctrl Pts',(5.2780590542116,138.980405391547,11.8365224392377));
#79744=CARTESIAN_POINT('Ctrl Pts',(5.28133794221558,139.043094612097,11.8364472844683));
#79745=CARTESIAN_POINT('Ctrl Pts',(5.28362124549377,139.087924597964,11.8384551228243));
#79746=CARTESIAN_POINT('Ctrl Pts',(5.28967052909967,139.208511052563,11.8494254871192));
#79747=CARTESIAN_POINT('Ctrl Pts',(5.29334217554952,139.283773927069,11.8622531415987));
#79748=CARTESIAN_POINT('Ctrl Pts',(5.30027948630146,139.421859560158,11.897058279467));
#79749=CARTESIAN_POINT('Ctrl Pts',(5.30352943641082,139.484848413172,11.9175632208407));
#79750=CARTESIAN_POINT('Ctrl Pts',(5.30781295347927,139.56132804225,11.9483314008382));
#79751=CARTESIAN_POINT('Ctrl Pts',(5.30866988649024,139.576325316098,11.9546575676899));
#79752=CARTESIAN_POINT('Ctrl Pts',(5.31000524925259,139.599158556797,11.9647409573135));
#79753=CARTESIAN_POINT('Ctrl Pts',(5.31047380481253,139.607072174531,11.9683202132259));
#79754=CARTESIAN_POINT('Ctrl Pts',(5.31134972829718,139.621671607149,11.975080577099));
#79755=CARTESIAN_POINT('Ctrl Pts',(5.31175596911822,139.62836583279,11.9782422929549));
#79756=CARTESIAN_POINT('Ctrl Pts',(5.31273302653917,139.644288424333,11.9859109056203));
#79757=CARTESIAN_POINT('Ctrl Pts',(5.3133065569548,139.653493730939,11.9904643369108));
#79758=CARTESIAN_POINT('Ctrl Pts',(5.31535867608064,139.685967685746,12.0069553337115));
#79759=CARTESIAN_POINT('Ctrl Pts',(5.31686475778166,139.708962377867,12.0194187415709));
#79760=CARTESIAN_POINT('Ctrl Pts',(5.32089736269073,139.768730419634,12.0539169971704));
#79761=CARTESIAN_POINT('Ctrl Pts',(5.32345860558771,139.804890608806,12.0769627669271));
#79762=CARTESIAN_POINT('Ctrl Pts',(5.33281180597075,139.932296393498,12.1662614260395));
#79763=CARTESIAN_POINT('Ctrl Pts',(5.33962666596036,140.016837633374,12.2414217710385));
#79764=CARTESIAN_POINT('Ctrl Pts',(5.34753799592571,140.109333988725,12.3450682312167));
#79765=CARTESIAN_POINT('Ctrl Pts',(5.34900743183869,140.126226327528,12.365050287922));
#79766=CARTESIAN_POINT('Ctrl Pts',(5.35128076508101,140.151894358731,12.3971190189345));
#79767=CARTESIAN_POINT('Ctrl Pts',(5.35209907743536,140.161035696619,12.408904711036));
#79768=CARTESIAN_POINT('Ctrl Pts',(5.35361041140312,140.177727815262,12.4311184677967));
#79769=CARTESIAN_POINT('Ctrl Pts',(5.35430517345941,140.185324176356,12.4415103172189));
#79770=CARTESIAN_POINT('Ctrl Pts',(5.35586828005345,140.202231417226,12.4652917951563));
#79771=CARTESIAN_POINT('Ctrl Pts',(5.3567333503536,140.211457651472,12.4787396545397));
#79772=CARTESIAN_POINT('Ctrl Pts',(5.3594060230579,140.239523420335,12.5211498845817));
#79773=CARTESIAN_POINT('Ctrl Pts',(5.36118445407896,140.257564041181,12.5506277776409));
#79774=CARTESIAN_POINT('Ctrl Pts',(5.36543710875225,140.29885030092,12.6237857619784));
#79775=CARTESIAN_POINT('Ctrl Pts',(5.36787707630344,140.320957619038,12.6680592058672));
#79776=CARTESIAN_POINT('Ctrl Pts',(5.37540776842262,140.382756508672,12.8093043572145));
#79777=CARTESIAN_POINT('Ctrl Pts',(5.38037692756727,140.414308946801,12.9094574267174));
#79778=CARTESIAN_POINT('Ctrl Pts',(5.38673295043903,140.438477576492,13.0299175922779));
#79779=CARTESIAN_POINT('Ctrl Pts',(5.38768614720088,140.441718983239,13.0477926243908));
#79780=CARTESIAN_POINT('Ctrl Pts',(5.38913466340411,140.446060253086,13.0745622270729));
#79781=CARTESIAN_POINT('Ctrl Pts',(5.38961708346854,140.447412596039,13.0834146507383));
#79782=CARTESIAN_POINT('Ctrl Pts',(5.39050443496787,140.449728652993,13.0995672244277));
#79783=CARTESIAN_POINT('Ctrl Pts',(5.39090793898311,140.450718642334,13.1068630575315));
#79784=CARTESIAN_POINT('Ctrl Pts',(5.39185898253675,140.452905636494,13.1239468995723));
#79785=CARTESIAN_POINT('Ctrl Pts',(5.39240881864613,140.454058816827,13.1337398759583));
#79786=CARTESIAN_POINT('Ctrl Pts',(5.39428038542812,140.457616102224,13.1668241583656));
#79787=CARTESIAN_POINT('Ctrl Pts',(5.3956238698896,140.459560081497,13.1901603255108));
#79788=CARTESIAN_POINT('Ctrl Pts',(5.39909354875647,140.463083174909,13.2496855062319));
#79789=CARTESIAN_POINT('Ctrl Pts',(5.40124463207642,140.463880114815,13.2859045974367));
#79790=CARTESIAN_POINT('Ctrl Pts',(5.41039807306712,140.461570852026,13.438713625626));
#79791=CARTESIAN_POINT('Ctrl Pts',(5.41749376015007,140.445878051767,13.55470449641));
#79792=CARTESIAN_POINT('Ctrl Pts',(5.42590183501994,140.40903585322,13.6966763473822));
#79793=CARTESIAN_POINT('Ctrl Pts',(5.42759736254931,140.40059902728,13.7255075908075));
#79794=CARTESIAN_POINT('Ctrl Pts',(5.43013576229703,140.386411919014,13.7689781273738));
#79795=CARTESIAN_POINT('Ctrl Pts',(5.43099903710802,140.381303591431,13.78381701962));
#79796=CARTESIAN_POINT('Ctrl Pts',(5.43256105048977,140.371541719345,13.8107578412828));
#79797=CARTESIAN_POINT('Ctrl Pts',(5.43326221014194,140.366964190116,13.8228854351483));
#79798=CARTESIAN_POINT('Ctrl Pts',(5.43478797649018,140.356575142137,13.8493406329289));
#79799=CARTESIAN_POINT('Ctrl Pts',(5.43561024045213,140.350696453762,13.8636402767373));
#79800=CARTESIAN_POINT('Ctrl Pts',(5.43799394653683,140.332842243807,13.9051854183788));
#79801=CARTESIAN_POINT('Ctrl Pts',(5.43953496512592,140.320260708261,13.9321626807603));
#79802=CARTESIAN_POINT('Ctrl Pts',(5.44308278099412,140.288950723886,13.9942782170509));
#79803=CARTESIAN_POINT('Ctrl Pts',(5.44506958116845,140.269593805768,14.0290734125879));
#79804=CARTESIAN_POINT('Ctrl Pts',(5.44993688475439,140.218108598054,14.1133377608396));
#79805=CARTESIAN_POINT('Ctrl Pts',(5.452781759856,140.184364210054,14.1617356846067));
#79806=CARTESIAN_POINT('Ctrl Pts',(5.45884913286976,140.107110750787,14.2593945744269));
#79807=CARTESIAN_POINT('Ctrl Pts',(5.46207162515903,140.063021218632,14.3080260697235));
#79808=CARTESIAN_POINT('Ctrl Pts',(5.46632215634683,140.004141926804,14.3647979244937));
#79809=CARTESIAN_POINT('Ctrl Pts',(5.46717667803751,139.992273047967,14.3758669922274));
#79810=CARTESIAN_POINT('Ctrl Pts',(5.46850904790812,139.973780999331,14.3925466026891));
#79811=CARTESIAN_POINT('Ctrl Pts',(5.46897708982476,139.967287572472,14.3982997123756));
#79812=CARTESIAN_POINT('Ctrl Pts',(5.46985261650331,139.95515708649,14.4088561825648));
#79813=CARTESIAN_POINT('Ctrl Pts',(5.47025898548705,139.949534151391,14.4136749886845));
#79814=CARTESIAN_POINT('Ctrl Pts',(5.47123712863113,139.936013512736,14.4250852285997));
#79815=CARTESIAN_POINT('Ctrl Pts',(5.47181163378226,139.928082551652,14.4316363516975));
#79816=CARTESIAN_POINT('Ctrl Pts',(5.47387153977532,139.899653743742,14.4546192206599));
#79817=CARTESIAN_POINT('Ctrl Pts',(5.47538469689689,139.878784219547,14.470581280652));
#79818=CARTESIAN_POINT('Ctrl Pts',(5.47944277972557,139.822517498149,14.5112640164428));
#79819=CARTESIAN_POINT('Ctrl Pts',(5.48202290309546,139.786436904842,14.5349948181222));
#79820=CARTESIAN_POINT('Ctrl Pts',(5.49147178306497,139.651445039794,14.6154643078039));
#79821=CARTESIAN_POINT('Ctrl Pts',(5.49836017198872,139.547026788292,14.6622026166579));
#79822=CARTESIAN_POINT('Ctrl Pts',(5.50627447615158,139.414197161587,14.7038901524748));
#79823=CARTESIAN_POINT('Ctrl Pts',(5.50768755231191,139.389970111386,14.7108119192568));
#79824=CARTESIAN_POINT('Ctrl Pts',(5.50989419562295,139.351329389669,14.7207801952475));
#79825=CARTESIAN_POINT('Ctrl Pts',(5.51070082119714,139.337028486189,14.7242403326006));
#79826=CARTESIAN_POINT('Ctrl Pts',(5.51220845294001,139.309974703634,14.7303557382969));
#79827=CARTESIAN_POINT('Ctrl Pts',(5.51291088256839,139.297233917155,14.733057524532));
#79828=CARTESIAN_POINT('Ctrl Pts',(5.51450111961948,139.268090259283,14.738832269715));
#79829=CARTESIAN_POINT('Ctrl Pts',(5.51538537814265,139.251667355918,14.741795498651));
#79830=CARTESIAN_POINT('Ctrl Pts',(5.51819652395127,139.198805570433,14.7504027146267));
#79831=CARTESIAN_POINT('Ctrl Pts',(5.52008946916763,139.162201739746,14.7549510518571));
#79832=CARTESIAN_POINT('Ctrl Pts',(5.52470719752459,139.071023163151,14.762796504619));
#79833=CARTESIAN_POINT('Ctrl Pts',(5.5273884606941,139.016361605603,14.7644284427876));
#79834=CARTESIAN_POINT('Ctrl Pts',(5.53432614235396,138.873959285715,14.7607038785996));
#79835=CARTESIAN_POINT('Ctrl Pts',(5.5385315852486,138.786575426571,14.7505135816117));
#79836=CARTESIAN_POINT('Ctrl Pts',(5.54420187072996,138.677942678452,14.7278126554631));
#79837=CARTESIAN_POINT('Ctrl Pts',(5.54540589547608,138.655362804147,14.7225311910118));
#79838=CARTESIAN_POINT('Ctrl Pts',(5.54712332221838,138.624044309751,14.7144163528826));
#79839=CARTESIAN_POINT('Ctrl Pts',(5.54761413656486,138.615191515355,14.7120335413478));
#79840=CARTESIAN_POINT('Ctrl Pts',(5.54851459195195,138.599143147112,14.7075518491842));
#79841=CARTESIAN_POINT('Ctrl Pts',(5.54892271245598,138.591940090674,14.7054805348877));
#79842=CARTESIAN_POINT('Ctrl Pts',(5.5497931973991,138.576733620486,14.700981001567));
#79843=CARTESIAN_POINT('Ctrl Pts',(5.55025625224375,138.568734718494,14.6985393969137));
#79844=CARTESIAN_POINT('Ctrl Pts',(5.55156957570382,138.546284493274,14.6914757237726));
#79845=CARTESIAN_POINT('Ctrl Pts',(5.55242804740352,138.531883856106,14.6866974038771));
#79846=CARTESIAN_POINT('Ctrl Pts',(5.5544260721784,138.498919713078,14.6751874950941));
#79847=CARTESIAN_POINT('Ctrl Pts',(5.55557214298547,138.480413086165,14.6683024066775));
#79848=CARTESIAN_POINT('Ctrl Pts',(5.55964517484957,138.415819653272,14.642772107222));
#79849=CARTESIAN_POINT('Ctrl Pts',(5.56263108570559,138.370550094219,14.6221558188611));
#79850=CARTESIAN_POINT('Ctrl Pts',(5.57215968650534,138.23009500097,14.5493400900722));
#79851=CARTESIAN_POINT('Ctrl Pts',(5.57867365104861,138.139607601796,14.4888380779715));
#79852=CARTESIAN_POINT('Ctrl Pts',(5.58612738079609,138.038916969706,14.4039423329906));
#79853=CARTESIAN_POINT('Ctrl Pts',(5.58742254039263,138.02155684579,14.3885854794396));
#79854=CARTESIAN_POINT('Ctrl Pts',(5.58948234907378,137.994179661264,14.363183203355));
#79855=CARTESIAN_POINT('Ctrl Pts',(5.59025751949347,137.983931613357,14.3533936259726));
#79856=CARTESIAN_POINT('Ctrl Pts',(5.59174043650857,137.96444098823,14.3342258396538));
#79857=CARTESIAN_POINT('Ctrl Pts',(5.59244899041773,137.955179639167,14.3248687640099));
#79858=CARTESIAN_POINT('Ctrl Pts',(5.59410289900716,137.933694258032,14.3025673215696));
#79859=CARTESIAN_POINT('Ctrl Pts',(5.59504359985574,137.921577546443,14.289522216996));
#79860=CARTESIAN_POINT('Ctrl Pts',(5.59830609660957,137.879972863463,14.2430575713872));
#79861=CARTESIAN_POINT('Ctrl Pts',(5.60057562209633,137.851774883274,14.2085141217825));
#79862=CARTESIAN_POINT('Ctrl Pts',(5.60656756534489,137.780275511439,14.1122675611804));
#79863=CARTESIAN_POINT('Ctrl Pts',(5.6101981834469,137.74008974083,14.0484203184192));
#79864=CARTESIAN_POINT('Ctrl Pts',(5.61741422150682,137.671059893276,13.9172988771268));
#79865=CARTESIAN_POINT('Ctrl Pts',(5.62098958648454,137.641986236878,13.8503963785111));
#79866=CARTESIAN_POINT('Ctrl Pts',(5.62551107200565,137.613610244128,13.7689722501961));
#79867=CARTESIAN_POINT('Ctrl Pts',(5.62622130129798,137.609377860415,13.7562691819363));
#79868=CARTESIAN_POINT('Ctrl Pts',(5.62737058769988,137.602899557178,13.7358972606584));
#79869=CARTESIAN_POINT('Ctrl Pts',(5.62780346399546,137.600541036462,13.7282647223738));
#79870=CARTESIAN_POINT('Ctrl Pts',(5.628660657519,137.596033157479,13.7132415669794));
#79871=CARTESIAN_POINT('Ctrl Pts',(5.62908472411609,137.59387940404,13.7058526198756));
#79872=CARTESIAN_POINT('Ctrl Pts',(5.63017827883031,137.588516195094,13.686897649915));
#79873=CARTESIAN_POINT('Ctrl Pts',(5.63085226363257,137.585390608779,13.6753086384701));
#79874=CARTESIAN_POINT('Ctrl Pts',(5.6339236577602,137.571930507609,13.622842789949));
#79875=CARTESIAN_POINT('Ctrl Pts',(5.63639408510215,137.563223535799,13.5815719847109));
#79876=CARTESIAN_POINT('Ctrl Pts',(5.64365701630666,137.543196703086,13.4610963525993));
#79877=CARTESIAN_POINT('Ctrl Pts',(5.64852536850634,137.536571038055,13.381264277037));
#79878=CARTESIAN_POINT('Ctrl Pts',(5.65328945758633,137.536500568152,13.3012895659352));
#79879=CARTESIAN_POINT('Ctrl Pts',(5.65328947433155,137.536500567904,13.3012892848334));
#79880=CARTESIAN_POINT('Ctrl Pts',(5.6533150753595,137.536500189299,13.3008595206364));
#79881=CARTESIAN_POINT('Ctrl Pts',(5.65334067327062,137.5365,13.3004297589952));
#79882=CARTESIAN_POINT('Ctrl Pts',(5.6533662680412,137.5365,13.3000000000336));
#79883=CARTESIAN_POINT('Origin',(4.2,139.,13.3));
#79884=CARTESIAN_POINT('',(6.22415553577981,137.536500247676,13.2991485609046));
#79885=CARTESIAN_POINT('',(6.1539436045687,137.5365,13.30000001305));
#79886=CARTESIAN_POINT('',(4.2,137.5365,13.3));
#79887=CARTESIAN_POINT('Ctrl Pts',(6.22273965880574,137.536500296291,13.2990687414511));
#79888=CARTESIAN_POINT('Ctrl Pts',(6.222044214228,137.536492446524,13.3114048768242));
#79889=CARTESIAN_POINT('Ctrl Pts',(6.2213535867996,137.53664057234,13.323740935255));
#79890=CARTESIAN_POINT('Ctrl Pts',(6.22001613084792,137.537233710625,13.3477968911271));
#79891=CARTESIAN_POINT('Ctrl Pts',(6.21936887733289,137.537663649918,13.3595161414469));
#79892=CARTESIAN_POINT('Ctrl Pts',(6.21807604716484,137.538811751986,13.383077486202));
#79893=CARTESIAN_POINT('Ctrl Pts',(6.2174306252796,137.539533140684,13.3949185428767));
#79894=CARTESIAN_POINT('Ctrl Pts',(6.21607770235265,137.541360165099,13.4198996497014));
#79895=CARTESIAN_POINT('Ctrl Pts',(6.21537136504241,137.542499579291,13.4330362125317));
#79896=CARTESIAN_POINT('Ctrl Pts',(6.21362057472982,137.5457900118,13.4658195203661));
#79897=CARTESIAN_POINT('Ctrl Pts',(6.21258341250646,137.548161781306,13.4854417471171));
#79898=CARTESIAN_POINT('Ctrl Pts',(6.20826591339485,137.559821838086,13.5678581426207));
#79899=CARTESIAN_POINT('Ctrl Pts',(6.20510621794372,137.572792873788,13.6300637899079));
#79900=CARTESIAN_POINT('Ctrl Pts',(6.19722307775851,137.616026451684,13.7859021479421));
#79901=CARTESIAN_POINT('Ctrl Pts',(6.19262035113756,137.651752558102,13.8776767969723));
#79902=CARTESIAN_POINT('Ctrl Pts',(6.18588796045833,137.713321831012,13.9983392664641));
#79903=CARTESIAN_POINT('Ctrl Pts',(6.18399774454713,137.731502086943,14.0308427064663));
#79904=CARTESIAN_POINT('Ctrl Pts',(6.18144287536967,137.756771656705,14.0722321539532));
#79905=CARTESIAN_POINT('Ctrl Pts',(6.18084280882312,137.762753870045,14.0817807944641));
#79906=CARTESIAN_POINT('Ctrl Pts',(6.17983686065803,137.772843056661,14.0974789989223));
#79907=CARTESIAN_POINT('Ctrl Pts',(6.17943512195257,137.77688736565,14.103668089127));
#79908=CARTESIAN_POINT('Ctrl Pts',(6.1785912915681,137.785411422791,14.1164992431133));
#79909=CARTESIAN_POINT('Ctrl Pts',(6.17814875790932,137.789898901364,14.123135317369));
#79910=CARTESIAN_POINT('Ctrl Pts',(6.17695534727235,137.802053652023,14.1407955240577));
#79911=CARTESIAN_POINT('Ctrl Pts',(6.17619840006465,137.80981838798,14.1517512958659));
#79912=CARTESIAN_POINT('Ctrl Pts',(6.17122124626072,137.861314030513,14.2223306466869));
#79913=CARTESIAN_POINT('Ctrl Pts',(6.16677943139859,137.909356331349,14.2786695943109));
#79914=CARTESIAN_POINT('Ctrl Pts',(6.15779942961889,138.014340880967,14.3844099122492));
#79915=CARTESIAN_POINT('Ctrl Pts',(6.15327552512922,138.071262475373,14.4335417597504));
#79916=CARTESIAN_POINT('Ctrl Pts',(6.14627893816397,138.167690663832,14.5046126808137));
#79917=CARTESIAN_POINT('Ctrl Pts',(6.14371871499775,138.204873696299,14.5294735811563));
#79918=CARTESIAN_POINT('Ctrl Pts',(6.14021488458455,138.258534348764,14.561897170226));
#79919=CARTESIAN_POINT('Ctrl Pts',(6.13921978228206,138.274099826181,14.5709149295976));
#79920=CARTESIAN_POINT('Ctrl Pts',(6.13750349103926,138.30150762835,14.5861256092759));
#79921=CARTESIAN_POINT('Ctrl Pts',(6.13677780642107,138.313275611648,14.5924474097258));
#79922=CARTESIAN_POINT('Ctrl Pts',(6.13527897273767,138.337947308381,14.6052690051632));
#79923=CARTESIAN_POINT('Ctrl Pts',(6.13450685801153,138.350864065961,14.6117406380377));
#79924=CARTESIAN_POINT('Ctrl Pts',(6.13247775877977,138.385339650733,14.6283798275873));
#79925=CARTESIAN_POINT('Ctrl Pts',(6.13123207788039,138.407055026696,14.6382139784917));
#79926=CARTESIAN_POINT('Ctrl Pts',(6.12491170941017,138.5198148705,14.6859950683551));
#79927=CARTESIAN_POINT('Ctrl Pts',(6.12012611455855,138.614285280199,14.7151981792919));
#79928=CARTESIAN_POINT('Ctrl Pts',(6.11273338811958,138.762712527666,14.745099194244));
#79929=CARTESIAN_POINT('Ctrl Pts',(6.11014859626989,138.814967612255,14.7527145284675));
#79930=CARTESIAN_POINT('Ctrl Pts',(6.10597138077205,138.897130728009,14.7601829995804));
#79931=CARTESIAN_POINT('Ctrl Pts',(6.10443893358022,138.926818050694,14.7619715003115));
#79932=CARTESIAN_POINT('Ctrl Pts',(6.10228719388142,138.967424482485,14.763177952371));
#79933=CARTESIAN_POINT('Ctrl Pts',(6.10170465908702,138.978314583121,14.7633798595471));
#79934=CARTESIAN_POINT('Ctrl Pts',(6.10070364707831,138.996826051883,14.7635163991386));
#79935=CARTESIAN_POINT('Ctrl Pts',(6.10028843238366,139.004446705273,14.7635130850595));
#79936=CARTESIAN_POINT('Ctrl Pts',(6.09939381986166,139.020733633276,14.7633787894919));
#79937=CARTESIAN_POINT('Ctrl Pts',(6.09891355985767,139.029399208304,14.7632303454761));
#79938=CARTESIAN_POINT('Ctrl Pts',(6.09751943514681,139.054349834836,14.7625812096661));
#79939=CARTESIAN_POINT('Ctrl Pts',(6.09659599328652,139.070628062481,14.7618855398829));
#79940=CARTESIAN_POINT('Ctrl Pts',(6.09213875034915,139.148217445811,14.7572707806052));
#79941=CARTESIAN_POINT('Ctrl Pts',(6.08846890548091,139.209249526039,14.749765524995));
#79942=CARTESIAN_POINT('Ctrl Pts',(6.07999781812186,139.347738764418,14.7238069538988));
#79943=CARTESIAN_POINT('Ctrl Pts',(6.07519974503492,139.424536506281,14.7028253306703));
#79944=CARTESIAN_POINT('Ctrl Pts',(6.06787074379707,139.542373624631,14.6600615069225));
#79945=CARTESIAN_POINT('Ctrl Pts',(6.06524085514309,139.58473675776,14.6423933847799));
#79946=CARTESIAN_POINT('Ctrl Pts',(6.0616640244784,139.642556275291,14.6150213066711));
#79947=CARTESIAN_POINT('Ctrl Pts',(6.06066260232415,139.658764811965,14.6069768810432));
#79948=CARTESIAN_POINT('Ctrl Pts',(6.05894116113815,139.686652140228,14.5924855414837));
#79949=CARTESIAN_POINT('Ctrl Pts',(6.05821649783322,139.698399424661,14.5861758420241));
#79950=CARTESIAN_POINT('Ctrl Pts',(6.05672524454002,139.72258029141,14.5727588224701));
#79951=CARTESIAN_POINT('Ctrl Pts',(6.05595959704273,139.734999109348,14.5656277598967));
#79952=CARTESIAN_POINT('Ctrl Pts',(6.05396171736826,139.7673938598,14.5463885676313));
#79953=CARTESIAN_POINT('Ctrl Pts',(6.0527402946741,139.787188403661,14.5339822905692));
#79954=CARTESIAN_POINT('Ctrl Pts',(6.04547812510897,139.904533117828,14.4564629364915));
#79955=CARTESIAN_POINT('Ctrl Pts',(6.03987724374481,139.994260212743,14.3802937459376));
#79956=CARTESIAN_POINT('Ctrl Pts',(6.03200053668788,140.103737340647,14.2620396483392));
#79957=CARTESIAN_POINT('Ctrl Pts',(6.02983677567864,140.132073434613,14.2285288100749));
#79958=CARTESIAN_POINT('Ctrl Pts',(6.02625469943177,140.175102436962,14.1727392465524));
#79959=CARTESIAN_POINT('Ctrl Pts',(6.02487879924249,140.190766589596,14.1512427953628));
#79960=CARTESIAN_POINT('Ctrl Pts',(6.02291658663522,140.21172554076,14.1207688460803));
#79961=CARTESIAN_POINT('Ctrl Pts',(6.02235987760694,140.21752400669,14.1121425770545));
#79962=CARTESIAN_POINT('Ctrl Pts',(6.02139311240099,140.227328075581,14.097216261855));
#79963=CARTESIAN_POINT('Ctrl Pts',(6.02098592347601,140.23137832815,14.0909458799062));
#79964=CARTESIAN_POINT('Ctrl Pts',(6.02009687029709,140.240047345375,14.0772969830976));
#79965=CARTESIAN_POINT('Ctrl Pts',(6.0196139719613,140.244648443965,14.0699079566835));
#79966=CARTESIAN_POINT('Ctrl Pts',(6.01821519839237,140.257679458185,14.0485589953317));
#79967=CARTESIAN_POINT('Ctrl Pts',(6.01728969379064,140.265942081212,14.0344990069006));
#79968=CARTESIAN_POINT('Ctrl Pts',(6.01255006059004,140.306565857409,13.9626497021191));
#79969=CARTESIAN_POINT('Ctrl Pts',(6.00857620792415,140.335210320654,13.9028524787359));
#79970=CARTESIAN_POINT('Ctrl Pts',(6.00000225040313,140.387852260403,13.7706262959092));
#79971=CARTESIAN_POINT('Ctrl Pts',(5.99541303730799,140.410444327656,13.6978333688117));
#79972=CARTESIAN_POINT('Ctrl Pts',(5.98834762946852,140.437181098722,13.5799115068666));
#79973=CARTESIAN_POINT('Ctrl Pts',(5.98578032340018,140.445077543099,13.5357783877591));
#79974=CARTESIAN_POINT('Ctrl Pts',(5.98227807868768,140.453270160398,13.4736564454145));
#79975=CARTESIAN_POINT('Ctrl Pts',(5.98129068485707,140.455279708766,13.4559221900238));
#79976=CARTESIAN_POINT('Ctrl Pts',(5.9795916161321,140.458208913983,13.425031185483));
#79977=CARTESIAN_POINT('Ctrl Pts',(5.97887539529392,140.459276016412,13.4118908310042));
#79978=CARTESIAN_POINT('Ctrl Pts',(5.97740040596324,140.461121995369,13.3845918454692));
#79979=CARTESIAN_POINT('Ctrl Pts',(5.97664258622784,140.461872950412,13.3704326757375));
#79980=CARTESIAN_POINT('Ctrl Pts',(5.97466377355011,140.463308148105,13.3331292281276));
#79981=CARTESIAN_POINT('Ctrl Pts',(5.97345353028372,140.463649156035,13.3099753526027));
#79982=CARTESIAN_POINT('Ctrl Pts',(5.96618680777581,140.4623814455,13.1691911392114));
#79983=CARTESIAN_POINT('Ctrl Pts',(5.96057870747964,140.447144646371,13.0521207858882));
#79984=CARTESIAN_POINT('Ctrl Pts',(5.95268614726718,140.407153658407,12.8954074642292));
#79985=CARTESIAN_POINT('Ctrl Pts',(5.95051439063421,140.394326073208,12.8531992158087));
#79986=CARTESIAN_POINT('Ctrl Pts',(5.94692175253812,140.370722674627,12.7865202126219));
#79987=CARTESIAN_POINT('Ctrl Pts',(5.94554434879728,140.361148027467,12.7616525051066));
#79988=CARTESIAN_POINT('Ctrl Pts',(5.94358314219853,140.346922785979,12.7275157622443));
#79989=CARTESIAN_POINT('Ctrl Pts',(5.94302944851173,140.342844005569,12.7180127508745));
#79990=CARTESIAN_POINT('Ctrl Pts',(5.94206783464265,140.335663267261,12.7017600353641));
#79991=CARTESIAN_POINT('Ctrl Pts',(5.94166278428657,140.332610072855,12.6949894130177));
#79992=CARTESIAN_POINT('Ctrl Pts',(5.94077624273421,140.325868394609,12.6803380352376));
#79993=CARTESIAN_POINT('Ctrl Pts',(5.94029370723431,140.32216113687,12.6724668369694));
#79994=CARTESIAN_POINT('Ctrl Pts',(5.93890173164414,140.31135175035,12.6500375308205));
#79995=CARTESIAN_POINT('Ctrl Pts',(5.9379828610423,140.304078004894,12.6355640454456));
#79996=CARTESIAN_POINT('Ctrl Pts',(5.93334773284171,140.26662035635,12.5640151742937));
#79997=CARTESIAN_POINT('Ctrl Pts',(5.92947981772648,140.232924584106,12.5088637569139));
#79998=CARTESIAN_POINT('Ctrl Pts',(5.92203714569948,140.161646071081,12.4078684184591));
#79999=CARTESIAN_POINT('Ctrl Pts',(5.91847208025445,140.124699950273,12.3617191890794));
#80000=CARTESIAN_POINT('Ctrl Pts',(5.91258293853601,140.057991392317,12.2880147026651));
#80001=CARTESIAN_POINT('Ctrl Pts',(5.91022534492137,140.029690866555,12.2592324348137));
#80002=CARTESIAN_POINT('Ctrl Pts',(5.90618938801653,139.978268926778,12.2110887822059));
#80003=CARTESIAN_POINT('Ctrl Pts',(5.90449151586008,139.95567243821,12.1912042071751));
#80004=CARTESIAN_POINT('Ctrl Pts',(5.90195692376185,139.920459404514,12.1620940792194));
#80005=CARTESIAN_POINT('Ctrl Pts',(5.90109959087046,139.908282801352,12.1523511951962));
#80006=CARTESIAN_POINT('Ctrl Pts',(5.89953829921091,139.885623926212,12.1348076814118));
#80007=CARTESIAN_POINT('Ctrl Pts',(5.89883210526393,139.875188560566,12.1269493289893));
#80008=CARTESIAN_POINT('Ctrl Pts',(5.89728328217412,139.851896388601,12.1098930156426));
#80009=CARTESIAN_POINT('Ctrl Pts',(5.89644325606804,139.838992869227,12.1007614571737));
#80010=CARTESIAN_POINT('Ctrl Pts',(5.89401723797274,139.800963415186,12.0747630821864));
#80011=CARTESIAN_POINT('Ctrl Pts',(5.8924521932004,139.775458630695,12.0584638664878));
#80012=CARTESIAN_POINT('Ctrl Pts',(5.88500388482994,139.649864501263,11.9835824309555));
#80013=CARTESIAN_POINT('Ctrl Pts',(5.87950877405515,139.543564051749,11.9362489200195));
#80014=CARTESIAN_POINT('Ctrl Pts',(5.87118770458335,139.382060112064,11.8862522972906));
#80015=CARTESIAN_POINT('Ctrl Pts',(5.86852864505822,139.330516332581,11.8733218755028));
#80016=CARTESIAN_POINT('Ctrl Pts',(5.86506664663542,139.265844331865,11.8607910787119));
#80017=CARTESIAN_POINT('Ctrl Pts',(5.86438761144379,139.253268745226,11.8585249053419));
#80018=CARTESIAN_POINT('Ctrl Pts',(5.86327447989685,139.232871245547,11.8551243401695));
#80019=CARTESIAN_POINT('Ctrl Pts',(5.86284580432276,139.225066750608,11.8538880952062));
#80020=CARTESIAN_POINT('Ctrl Pts',(5.86203363893271,139.210386569871,11.8516844443037));
#80021=CARTESIAN_POINT('Ctrl Pts',(5.86165098199122,139.203513232919,11.8507026470455));
#80022=CARTESIAN_POINT('Ctrl Pts',(5.86060846822576,139.184895108791,11.848178259011));
#80023=CARTESIAN_POINT('Ctrl Pts',(5.85994371603298,139.173138379242,11.8467293259645));
#80024=CARTESIAN_POINT('Ctrl Pts',(5.85720491314605,139.125101023145,11.8414002262686));
#80025=CARTESIAN_POINT('Ctrl Pts',(5.85507721592598,139.08870099091,11.8387350276837));
#80026=CARTESIAN_POINT('Ctrl Pts',(5.84669517950804,138.947196026553,11.8336805326472));
#80027=CARTESIAN_POINT('Ctrl Pts',(5.84025725618538,138.842049281319,11.8412556799315));
#80028=CARTESIAN_POINT('Ctrl Pts',(5.83101251125895,138.68746545757,11.8693159357432));
#80029=CARTESIAN_POINT('Ctrl Pts',(5.82801624564579,138.636843277737,11.8813200415955));
#80030=CARTESIAN_POINT('Ctrl Pts',(5.82405237315119,138.568964275335,11.9012890073804));
#80031=CARTESIAN_POINT('Ctrl Pts',(5.82301232399686,138.551068577809,11.9069296998691));
#80032=CARTESIAN_POINT('Ctrl Pts',(5.82124931482719,138.52059744695,11.917182347678));
#80033=CARTESIAN_POINT('Ctrl Pts',(5.82052095254888,138.50796811122,11.9216255572136));
#80034=CARTESIAN_POINT('Ctrl Pts',(5.81904329849012,138.48227281332,11.9310637637119));
#80035=CARTESIAN_POINT('Ctrl Pts',(5.81829460477804,138.469213916878,11.9360740447966));
#80036=CARTESIAN_POINT('Ctrl Pts',(5.81638724512933,138.435862584686,11.9494214461254));
#80037=CARTESIAN_POINT('Ctrl Pts',(5.81523771369553,138.415681825091,11.9580291395752));
#80038=CARTESIAN_POINT('Ctrl Pts',(5.80798446849508,138.288089788978,12.015875160176));
#80039=CARTESIAN_POINT('Ctrl Pts',(5.80233787926683,138.186785184517,12.0775124080618));
#80040=CARTESIAN_POINT('Ctrl Pts',(5.79437664164933,138.058724127397,12.1784615884725));
#80041=CARTESIAN_POINT('Ctrl Pts',(5.79216520176852,138.024758791509,12.2078677498098));
#80042=CARTESIAN_POINT('Ctrl Pts',(5.78851500752631,137.972645537959,12.2573579937815));
#80043=CARTESIAN_POINT('Ctrl Pts',(5.78712095805331,137.953608394412,12.2764649578319));
#80044=CARTESIAN_POINT('Ctrl Pts',(5.78513817249175,137.927960755744,12.3036703544242));
#80045=CARTESIAN_POINT('Ctrl Pts',(5.78458007238846,137.920891861777,12.3113309364265));
#80046=CARTESIAN_POINT('Ctrl Pts',(5.78361218002465,137.908904649935,12.3246032315321));
#80047=CARTESIAN_POINT('Ctrl Pts',(5.78320531060899,137.903946411247,12.330178136015));
#80048=CARTESIAN_POINT('Ctrl Pts',(5.78231719941338,137.893301895956,12.3423324337592));
#80049=CARTESIAN_POINT('Ctrl Pts',(5.7818349476132,137.887631562945,12.348924654229));
#80050=CARTESIAN_POINT('Ctrl Pts',(5.78044402150243,137.871576333891,12.3679301469697));
#80051=CARTESIAN_POINT('Ctrl Pts',(5.77952592971365,137.86133843644,12.3804653454155));
#80052=CARTESIAN_POINT('Ctrl Pts',(5.77490422749186,137.811441086024,12.4436705353262));
#80053=CARTESIAN_POINT('Ctrl Pts',(5.77104989921061,137.774948046035,12.4967447758345));
#80054=CARTESIAN_POINT('Ctrl Pts',(5.76372100027898,137.712736949158,12.6013728939457));
#80055=CARTESIAN_POINT('Ctrl Pts',(5.76025635280797,137.686331842526,12.6523871454748));
#80056=CARTESIAN_POINT('Ctrl Pts',(5.75320684658108,137.637995404598,12.760970174725));
#80057=CARTESIAN_POINT('Ctrl Pts',(5.74963844029193,137.616560165947,12.8186421958136));
#80058=CARTESIAN_POINT('Ctrl Pts',(5.74508335810925,137.593140617498,12.8963106942074));
#80059=CARTESIAN_POINT('Ctrl Pts',(5.74399201146777,137.587847054098,12.9152371014115));
#80060=CARTESIAN_POINT('Ctrl Pts',(5.74216973223066,137.579553863482,12.9473696099917));
#80061=CARTESIAN_POINT('Ctrl Pts',(5.74143244174944,137.576353529733,12.9605207463537));
#80062=CARTESIAN_POINT('Ctrl Pts',(5.73995852077226,137.570273212558,12.9871065891242));
#80063=CARTESIAN_POINT('Ctrl Pts',(5.73922214162866,137.567399065723,13.0005412315861));
#80064=CARTESIAN_POINT('Ctrl Pts',(5.73738955708814,137.560664290573,13.034341306802));
#80065=CARTESIAN_POINT('Ctrl Pts',(5.73630108586578,137.557046276954,13.0547522980622));
#80066=CARTESIAN_POINT('Ctrl Pts',(5.73131828483472,137.542305501869,13.1495939443217));
#80067=CARTESIAN_POINT('Ctrl Pts',(5.72759032558515,137.536500000002,13.2247384293328));
#80068=CARTESIAN_POINT('Ctrl Pts',(5.72391728548022,137.5365,13.299999999962));
#80069=CARTESIAN_POINT('Ctrl Pts',(5.6533662680412,137.5365,13.3000000000336));
#80070=CARTESIAN_POINT('Ctrl Pts',(5.65697576249153,137.536499999999,13.2393933779925));
#80071=CARTESIAN_POINT('Ctrl Pts',(5.66051905483574,137.540264715002,13.1788398257535));
#80072=CARTESIAN_POINT('Ctrl Pts',(5.66493101344803,137.549915832198,13.1015388318754));
#80073=CARTESIAN_POINT('Ctrl Pts',(5.66590078546337,137.552360588956,13.0844284336989));
#80074=CARTESIAN_POINT('Ctrl Pts',(5.66757947452231,137.557162490758,13.0546039247781));
#80075=CARTESIAN_POINT('Ctrl Pts',(5.6682924378738,137.559386067369,13.0418705285407));
#80076=CARTESIAN_POINT('Ctrl Pts',(5.66972008679681,137.564211833059,13.0162438632421));
#80077=CARTESIAN_POINT('Ctrl Pts',(5.67043451871115,137.566819723821,13.0033528742392));
#80078=CARTESIAN_POINT('Ctrl Pts',(5.67190907110246,137.57260468111,12.9766169900121));
#80079=CARTESIAN_POINT('Ctrl Pts',(5.67266819879496,137.575810260272,12.9627796387201));
#80080=CARTESIAN_POINT('Ctrl Pts',(5.67465794725342,137.584813131011,12.9263386360229));
#80081=CARTESIAN_POINT('Ctrl Pts',(5.67587763759821,137.590950535077,12.9038228006479));
#80082=CARTESIAN_POINT('Ctrl Pts',(5.68297053624817,137.630250783349,12.7721411094394));
#80083=CARTESIAN_POINT('Ctrl Pts',(5.68842942902264,137.675546905034,12.6670123508193));
#80084=CARTESIAN_POINT('Ctrl Pts',(5.69622892650164,137.7554690448,12.5285939362078));
#80085=CARTESIAN_POINT('Ctrl Pts',(5.69847955861117,137.780185076684,12.4900767073825));
#80086=CARTESIAN_POINT('Ctrl Pts',(5.70218479769977,137.822438041925,12.43056185106));
#80087=CARTESIAN_POINT('Ctrl Pts',(5.70359287116361,137.838830172965,12.4087877251487));
#80088=CARTESIAN_POINT('Ctrl Pts',(5.70559029422991,137.862318361711,12.3793364475598));
#80089=CARTESIAN_POINT('Ctrl Pts',(5.70614826520265,137.868903880071,12.3712576020478));
#80090=CARTESIAN_POINT('Ctrl Pts',(5.70711386780697,137.88032586865,12.3575472518085));
#80091=CARTESIAN_POINT('Ctrl Pts',(5.70751854574648,137.885119830445,12.3518810469976));
#80092=CARTESIAN_POINT('Ctrl Pts',(5.70839898750365,137.895560418243,12.3397295209064));
#80093=CARTESIAN_POINT('Ctrl Pts',(5.7088757020187,137.901221147062,12.3332574243764));
#80094=CARTESIAN_POINT('Ctrl Pts',(5.71024272975254,137.917486988537,12.314987572934));
#80095=CARTESIAN_POINT('Ctrl Pts',(5.71114204658586,137.928227066828,12.3033121653655));
#80096=CARTESIAN_POINT('Ctrl Pts',(5.71673256266189,137.995382236531,12.2326493314217));
#80097=CARTESIAN_POINT('Ctrl Pts',(5.72167012102453,138.056457438729,12.1782959172463));
#80098=CARTESIAN_POINT('Ctrl Pts',(5.73056645239369,138.174619641106,12.0896489629321));
#80099=CARTESIAN_POINT('Ctrl Pts',(5.73452429668179,138.230130455645,12.0536034102975));
#80100=CARTESIAN_POINT('Ctrl Pts',(5.74078273043686,138.324086738216,12.0012737112748));
#80101=CARTESIAN_POINT('Ctrl Pts',(5.74314875636077,138.361123529924,11.9826594833613));
#80102=CARTESIAN_POINT('Ctrl Pts',(5.7464311898699,138.414743363113,11.9585050307912));
#80103=CARTESIAN_POINT('Ctrl Pts',(5.74739137224624,138.430709932742,11.9516517736723));
#80104=CARTESIAN_POINT('Ctrl Pts',(5.74905892724868,138.458927140236,11.940130841145));
#80105=CARTESIAN_POINT('Ctrl Pts',(5.74977036242739,138.47112527388,11.9353405155711));
#80106=CARTESIAN_POINT('Ctrl Pts',(5.75124961530128,138.496815553994,11.925647906543));
#80107=CARTESIAN_POINT('Ctrl Pts',(5.75201626322393,138.510318837146,11.9207789727201));
#80108=CARTESIAN_POINT('Ctrl Pts',(5.75405179314551,138.546657799159,11.9082770642428));
#80109=CARTESIAN_POINT('Ctrl Pts',(5.75530877724265,138.569614267595,11.9010074738027));
#80110=CARTESIAN_POINT('Ctrl Pts',(5.76165962002447,138.687977340127,11.866715142009));
#80111=CARTESIAN_POINT('Ctrl Pts',(5.76645666101301,138.785771727214,11.84887228459));
#80112=CARTESIAN_POINT('Ctrl Pts',(5.77395428176452,138.939499799882,11.8367153341214));
#80113=CARTESIAN_POINT('Ctrl Pts',(5.77663737081935,138.994572709531,11.8354754283577));
#80114=CARTESIAN_POINT('Ctrl Pts',(5.78095528113385,139.080040614718,11.8383726249417));
#80115=CARTESIAN_POINT('Ctrl Pts',(5.7825227818539,139.110458335318,11.8403562744335));
#80116=CARTESIAN_POINT('Ctrl Pts',(5.78470946486359,139.151580241848,11.8443306698612));
#80117=CARTESIAN_POINT('Ctrl Pts',(5.78528892739312,139.162358312024,11.8454933713165));
#80118=CARTESIAN_POINT('Ctrl Pts',(5.78627937891608,139.180554097086,11.8476610292999));
#80119=CARTESIAN_POINT('Ctrl Pts',(5.78668700117038,139.187979010471,11.8486033766396));
#80120=CARTESIAN_POINT('Ctrl Pts',(5.787558896572,139.203718181919,11.8507237458842));
#80121=CARTESIAN_POINT('Ctrl Pts',(5.78802389826536,139.212029921588,11.8519164169021));
#80122=CARTESIAN_POINT('Ctrl Pts',(5.78934811970957,139.235485320512,11.8554883518329));
#80123=CARTESIAN_POINT('Ctrl Pts',(5.79021574391387,139.250602122528,11.8580340585846));
#80124=CARTESIAN_POINT('Ctrl Pts',(5.79727733072901,139.371908243837,11.8804273599112));
#80125=CARTESIAN_POINT('Ctrl Pts',(5.80390257703309,139.475638444459,11.9117388218285));
#80126=CARTESIAN_POINT('Ctrl Pts',(5.8133645079529,139.621144096273,11.9739031131033));
#80127=CARTESIAN_POINT('Ctrl Pts',(5.81632986685041,139.666270649019,11.9959919421423));
#80128=CARTESIAN_POINT('Ctrl Pts',(5.82124112551004,139.740687077363,12.0372915602315));
#80129=CARTESIAN_POINT('Ctrl Pts',(5.82322093362158,139.770584946117,12.055311654391));
#80130=CARTESIAN_POINT('Ctrl Pts',(5.82607342195843,139.813518275877,12.0833290766765));
#80131=CARTESIAN_POINT('Ctrl Pts',(5.82697559271159,139.827074062998,12.0925031487259));
#80132=CARTESIAN_POINT('Ctrl Pts',(5.82857240202151,139.851016516525,12.1092989483834));
#80133=CARTESIAN_POINT('Ctrl Pts',(5.82927021660863,139.86146166295,12.1168339407565));
#80134=CARTESIAN_POINT('Ctrl Pts',(5.83076286949335,139.883756579928,12.1333689868138));
#80135=CARTESIAN_POINT('Ctrl Pts',(5.83155586106612,139.895571362298,12.1424139036313));
#80136=CARTESIAN_POINT('Ctrl Pts',(5.83371479382208,139.927631320412,12.1677423930271));
#80137=CARTESIAN_POINT('Ctrl Pts',(5.83506635647265,139.947584462736,12.1843876357522));
#80138=CARTESIAN_POINT('Ctrl Pts',(5.84219773149226,140.051889601134,12.2762192644865));
#80139=CARTESIAN_POINT('Ctrl Pts',(5.84758776100299,140.127760627587,12.3604492426307));
#80140=CARTESIAN_POINT('Ctrl Pts',(5.85521029515537,140.218040440163,12.4875642707814));
#80141=CARTESIAN_POINT('Ctrl Pts',(5.8573289085875,140.241340057753,12.523631005899));
#80142=CARTESIAN_POINT('Ctrl Pts',(5.86084302808322,140.276243026866,12.5832565921059));
#80143=CARTESIAN_POINT('Ctrl Pts',(5.86219769897589,140.288856966002,12.6061953146103));
#80144=CARTESIAN_POINT('Ctrl Pts',(5.86413144545184,140.3055553693,12.6385901644603));
#80145=CARTESIAN_POINT('Ctrl Pts',(5.86468172313351,140.310165985271,12.6477708441284));
#80146=CARTESIAN_POINT('Ctrl Pts',(5.8656385614609,140.31793176553,12.6636487543553));
#80147=CARTESIAN_POINT('Ctrl Pts',(5.86604232001495,140.321133403085,12.6703226413633));
#80148=CARTESIAN_POINT('Ctrl Pts',(5.86692632877688,140.327978043523,12.684872487048));
#80149=CARTESIAN_POINT('Ctrl Pts',(5.86740762163779,140.331601675158,12.6927566285216));
#80150=CARTESIAN_POINT('Ctrl Pts',(5.86880146119969,140.341810418521,12.7154992016563));
#80151=CARTESIAN_POINT('Ctrl Pts',(5.86972354831471,140.348218232883,12.7304353112508));
#80152=CARTESIAN_POINT('Ctrl Pts',(5.87444010108554,140.379350713558,12.8064734133424));
#80153=CARTESIAN_POINT('Ctrl Pts',(5.87839261959991,140.40017448443,12.8690857994544));
#80154=CARTESIAN_POINT('Ctrl Pts',(5.88593417453586,140.43158689687,12.9903064563344));
#80155=CARTESIAN_POINT('Ctrl Pts',(5.88951340184243,140.442962802065,13.0485839523468));
#80156=CARTESIAN_POINT('Ctrl Pts',(5.89535748610721,140.455959657195,13.1464797876939));
#80157=CARTESIAN_POINT('Ctrl Pts',(5.89765902870917,140.459567455845,13.1857626298503));
#80158=CARTESIAN_POINT('Ctrl Pts',(5.90160904877756,140.463096435683,13.254668406482));
#80159=CARTESIAN_POINT('Ctrl Pts',(5.90327601833361,140.463713656544,13.2842316146644));
#80160=CARTESIAN_POINT('Ctrl Pts',(5.90577059080835,140.463289659303,13.3292117398176));
#80161=CARTESIAN_POINT('Ctrl Pts',(5.90661803458687,140.462900719914,13.3446258007389));
#80162=CARTESIAN_POINT('Ctrl Pts',(5.90816360619895,140.461736870412,13.3729753634333));
#80163=CARTESIAN_POINT('Ctrl Pts',(5.90886389101222,140.461033609066,13.3859121071203));
#80164=CARTESIAN_POINT('Ctrl Pts',(5.91040205680386,140.459097131236,13.4145201511361));
#80165=CARTESIAN_POINT('Ctrl Pts',(5.91123733109681,140.457783020476,13.430184462665));
#80166=CARTESIAN_POINT('Ctrl Pts',(5.91365503742473,140.45320842033,13.4758666851387));
#80167=CARTESIAN_POINT('Ctrl Pts',(5.91521651274233,140.449271028005,13.5058092617556));
#80168=CARTESIAN_POINT('Ctrl Pts',(5.92320795417005,140.424011930144,13.6606604578252));
#80169=CARTESIAN_POINT('Ctrl Pts',(5.92915707016481,140.387463903187,13.782522653517));
#80170=CARTESIAN_POINT('Ctrl Pts',(5.93763254924681,140.317623140847,13.9384775904453));
#80171=CARTESIAN_POINT('Ctrl Pts',(5.93986629223164,140.297749527945,13.9779601173162));
#80172=CARTESIAN_POINT('Ctrl Pts',(5.94283266149028,140.270171550407,14.0270792535848));
#80173=CARTESIAN_POINT('Ctrl Pts',(5.94347967245631,140.264088954362,14.0376036229821));
#80174=CARTESIAN_POINT('Ctrl Pts',(5.94455098484331,140.253927321835,14.0546908019192));
#80175=CARTESIAN_POINT('Ctrl Pts',(5.94497051413286,140.2499260164,14.0612994712912));
#80176=CARTESIAN_POINT('Ctrl Pts',(5.94582876313332,140.241702163078,14.0746426060735));
#80177=CARTESIAN_POINT('Ctrl Pts',(5.94626763921887,140.237476741196,14.0813749022207));
#80178=CARTESIAN_POINT('Ctrl Pts',(5.94744401771789,140.226090987063,14.0991916378737));
#80179=CARTESIAN_POINT('Ctrl Pts',(5.94818731514329,140.218835366291,14.1102139887132));
#80180=CARTESIAN_POINT('Ctrl Pts',(5.95261557662548,140.175181980069,14.1746163373711));
#80181=CARTESIAN_POINT('Ctrl Pts',(5.95647032850294,140.135433269071,14.2256329228595));
#80182=CARTESIAN_POINT('Ctrl Pts',(5.96660487842762,140.023307145018,14.3514138633291));
#80183=CARTESIAN_POINT('Ctrl Pts',(5.97288412030695,139.946092433288,14.4214021463712));
#80184=CARTESIAN_POINT('Ctrl Pts',(5.98061089440359,139.837237049878,14.5007554754419));
#80185=CARTESIAN_POINT('Ctrl Pts',(5.9823490665748,139.811798316072,14.5180982235904));
#80186=CARTESIAN_POINT('Ctrl Pts',(5.98492633364281,139.772625888458,14.5430311633009));
#80187=CARTESIAN_POINT('Ctrl Pts',(5.98578729338112,139.759287312848,14.5512234172284));
#80188=CARTESIAN_POINT('Ctrl Pts',(5.98734728210769,139.734662029811,14.5658088773062));
#80189=CARTESIAN_POINT('Ctrl Pts',(5.98804868636133,139.723416975461,14.5722689599892));
#80190=CARTESIAN_POINT('Ctrl Pts',(5.9895774872314,139.698534343617,14.5861270066639));
#80191=CARTESIAN_POINT('Ctrl Pts',(5.99040249398316,139.684861915198,14.5934593493193));
#80192=CARTESIAN_POINT('Ctrl Pts',(5.99275371047503,139.645218577311,14.6139146836974));
#80193=CARTESIAN_POINT('Ctrl Pts',(5.99426080569329,139.618968931615,14.6264827237329));
#80194=CARTESIAN_POINT('Ctrl Pts',(5.99774695640422,139.55650277023,14.6541324303148));
#80195=CARTESIAN_POINT('Ctrl Pts',(5.99970622901512,139.52001994584,14.6685574454841));
#80196=CARTESIAN_POINT('Ctrl Pts',(6.0045889324306,139.426584480367,14.701224360436));
#80197=CARTESIAN_POINT('Ctrl Pts',(6.00747351366385,139.36901276103,14.717474417418));
#80198=CARTESIAN_POINT('Ctrl Pts',(6.01359016967776,139.246345875599,14.7441158223409));
#80199=CARTESIAN_POINT('Ctrl Pts',(6.01682155523195,139.181220397575,14.753724342107));
#80200=CARTESIAN_POINT('Ctrl Pts',(6.02108275488072,139.09947871777,14.7602055484217));
#80201=CARTESIAN_POINT('Ctrl Pts',(6.02193827720658,139.083261583861,14.7612199440886));
#80202=CARTESIAN_POINT('Ctrl Pts',(6.02327211548137,139.058356607022,14.7623618464705));
#80203=CARTESIAN_POINT('Ctrl Pts',(6.02374061167786,139.049678472142,14.7626823665254));
#80204=CARTESIAN_POINT('Ctrl Pts',(6.02461742149734,139.033580154739,14.7631335189008));
#80205=CARTESIAN_POINT('Ctrl Pts',(6.02502462531589,139.026161067507,14.7632849725592));
#80206=CARTESIAN_POINT('Ctrl Pts',(6.02600531581143,139.008424122384,14.7635121267794));
#80207=CARTESIAN_POINT('Ctrl Pts',(6.02658155015462,138.99810616258,14.7635351420108));
#80208=CARTESIAN_POINT('Ctrl Pts',(6.02865032523758,138.96139198578,14.7632288027181));
#80209=CARTESIAN_POINT('Ctrl Pts',(6.03017080556315,138.935007142182,14.762294385749));
#80210=CARTESIAN_POINT('Ctrl Pts',(6.03425517211736,138.865257064081,14.7579328145923));
#80211=CARTESIAN_POINT('Ctrl Pts',(6.03685460391053,138.821994932134,14.7532851057885));
#80212=CARTESIAN_POINT('Ctrl Pts',(6.04641928212429,138.664694571314,14.729256652979));
#80213=CARTESIAN_POINT('Ctrl Pts',(6.05339910789472,138.552835589036,14.6983047196228));
#80214=CARTESIAN_POINT('Ctrl Pts',(6.06131903926754,138.423527407056,14.6453957206966));
#80215=CARTESIAN_POINT('Ctrl Pts',(6.06266448652038,138.401502376958,14.635743608258));
#80216=CARTESIAN_POINT('Ctrl Pts',(6.06478431823162,138.366719099659,14.619467209964));
#80217=CARTESIAN_POINT('Ctrl Pts',(6.06557031596723,138.353803951958,14.613190429847));
#80218=CARTESIAN_POINT('Ctrl Pts',(6.06706229219365,138.329262805641,14.6008136549379));
#80219=CARTESIAN_POINT('Ctrl Pts',(6.06776927869749,138.317622478903,14.5947453351638));
#80220=CARTESIAN_POINT('Ctrl Pts',(6.06940245757921,138.290718831501,14.5802563368812));
#80221=CARTESIAN_POINT('Ctrl Pts',(6.0703243842096,138.275521031118,14.5717178626686));
#80222=CARTESIAN_POINT('Ctrl Pts',(6.0734228321803,138.224465170957,14.5418211215038));
#80223=CARTESIAN_POINT('Ctrl Pts',(6.07555433134893,138.189368282953,14.5192007934152));
#80224=CARTESIAN_POINT('Ctrl Pts',(6.08100162206062,138.100656327443,14.4564982730705));
#80225=CARTESIAN_POINT('Ctrl Pts',(6.08424755849882,138.048738442852,14.4141854724613));
#80226=CARTESIAN_POINT('Ctrl Pts',(6.09141875441242,137.941001027503,14.3133415492535));
#80227=CARTESIAN_POINT('Ctrl Pts',(6.09533386832001,137.886770008277,14.2534444714429));
#80228=CARTESIAN_POINT('Ctrl Pts',(6.10035156963313,137.828166169026,14.1768618397456));
#80229=CARTESIAN_POINT('Ctrl Pts',(6.1011832123673,137.81878092496,14.1641774533306));
#80230=CARTESIAN_POINT('Ctrl Pts',(6.10248718083329,137.804611665318,14.1443652056503));
#80231=CARTESIAN_POINT('Ctrl Pts',(6.10295033497054,137.799681960186,14.137342502853));
#80232=CARTESIAN_POINT('Ctrl Pts',(6.10382039045731,137.79062011418,14.1241888135682));
#80233=CARTESIAN_POINT('Ctrl Pts',(6.10422625624439,137.786472267466,14.1180692774802));
#80234=CARTESIAN_POINT('Ctrl Pts',(6.10520919734878,137.776613695097,14.1032844423948));
#80235=CARTESIAN_POINT('Ctrl Pts',(6.10578912543287,137.770948544979,14.0945894880172));
#80236=CARTESIAN_POINT('Ctrl Pts',(6.10790681526746,137.750782483832,14.0629066492488));
#80237=CARTESIAN_POINT('Ctrl Pts',(6.10947463367642,137.736830872648,14.0395772661838));
#80238=CARTESIAN_POINT('Ctrl Pts',(6.1137346422948,137.701240172514,13.9761161658724));
#80239=CARTESIAN_POINT('Ctrl Pts',(6.11646629783227,137.680813312742,13.9353394864149));
#80240=CARTESIAN_POINT('Ctrl Pts',(6.12629454618935,137.614609778026,13.7861696165259));
#80241=CARTESIAN_POINT('Ctrl Pts',(6.13338760801281,137.580022259446,13.6732811597668));
#80242=CARTESIAN_POINT('Ctrl Pts',(6.14127450084188,137.555452133638,13.5357925116783));
#80243=CARTESIAN_POINT('Ctrl Pts',(6.14250239594808,137.552069405187,13.5140413837613));
#80244=CARTESIAN_POINT('Ctrl Pts',(6.14448003346254,137.547354132912,13.4784521085903));
#80245=CARTESIAN_POINT('Ctrl Pts',(6.14523895209424,137.54572589518,13.4646572715126));
#80246=CARTESIAN_POINT('Ctrl Pts',(6.1467063820322,137.542935031073,13.4377237655496));
#80247=CARTESIAN_POINT('Ctrl Pts',(6.14741543291234,137.541753146379,13.4245884781647));
#80248=CARTESIAN_POINT('Ctrl Pts',(6.1490947416746,137.539356311365,13.3932027575419));
#80249=CARTESIAN_POINT('Ctrl Pts',(6.15005978637313,137.538305604865,13.3749418047271));
#80250=CARTESIAN_POINT('Ctrl Pts',(6.15200166140935,137.536865783236,13.337783340469));
#80251=CARTESIAN_POINT('Ctrl Pts',(6.15297747730672,137.536500000168,13.3188913700656));
#80252=CARTESIAN_POINT('Ctrl Pts',(6.1539436045687,137.5365,13.30000001305));
#80253=CARTESIAN_POINT('Origin',(1.13913288526384,139.,13.3));
#80254=CARTESIAN_POINT('',(2.4607468847319,137.88614821265,13.6826607614027));
#80255=CARTESIAN_POINT('',(2.36281348338426,137.886148197203,13.6826607164382));
#80256=CARTESIAN_POINT('',(1.13913288526384,137.88614821265,13.6826607614027));
#80257=CARTESIAN_POINT('',(2.06349999999998,138.327116518419,12.3333962121348));
#80258=CARTESIAN_POINT('Ctrl Pts',(2.46074688473191,137.88614821265,13.6826607614027));
#80259=CARTESIAN_POINT('Ctrl Pts',(2.45928397525449,137.89272897163,13.701816083534));
#80260=CARTESIAN_POINT('Ctrl Pts',(2.45783385173158,137.899805886111,13.7208075478205));
#80261=CARTESIAN_POINT('Ctrl Pts',(2.45549200100449,137.91219985181,13.7516116641803));
#80262=CARTESIAN_POINT('Ctrl Pts',(2.45458867175444,137.917223828975,13.7635278372366));
#80263=CARTESIAN_POINT('Ctrl Pts',(2.45315465607098,137.92560881407,13.7825351313431));
#80264=CARTESIAN_POINT('Ctrl Pts',(2.45261724523232,137.92884607051,13.7896793272959));
#80265=CARTESIAN_POINT('Ctrl Pts',(2.45154083877098,137.935527919108,13.8040418697068));
#80266=CARTESIAN_POINT('Ctrl Pts',(2.45100202155896,137.938975128628,13.8112584954435));
#80267=CARTESIAN_POINT('Ctrl Pts',(2.44955373087507,137.948511270729,13.8307101520025));
#80268=CARTESIAN_POINT('Ctrl Pts',(2.44865230826454,137.954740264935,13.8428756203764));
#80269=CARTESIAN_POINT('Ctrl Pts',(2.44661626077223,137.969445941233,13.870404383881));
#80270=CARTESIAN_POINT('Ctrl Pts',(2.44548826582058,137.978057098827,13.8856924102223));
#80271=CARTESIAN_POINT('Ctrl Pts',(2.44158744149147,138.009328372448,13.9384195598443));
#80272=CARTESIAN_POINT('Ctrl Pts',(2.4388772983383,138.033731260977,13.9747851473174));
#80273=CARTESIAN_POINT('Ctrl Pts',(2.43142808267214,138.106345354465,14.0709508714327));
#80274=CARTESIAN_POINT('Ctrl Pts',(2.42670574502547,138.158457623931,14.1275197170264));
#80275=CARTESIAN_POINT('Ctrl Pts',(2.42038367873486,138.23155745979,14.1927726647626));
#80276=CARTESIAN_POINT('Ctrl Pts',(2.41899696075887,138.247795763608,14.2064963677247));
#80277=CARTESIAN_POINT('Ctrl Pts',(2.41668526924672,138.275120239638,14.2283495983067));
#80278=CARTESIAN_POINT('Ctrl Pts',(2.41577079766173,138.285993514856,14.2367381469551));
#80279=CARTESIAN_POINT('Ctrl Pts',(2.41394526472066,138.307806678174,14.2529661761489));
#80280=CARTESIAN_POINT('Ctrl Pts',(2.41303464185118,138.318739201053,14.26081206558));
#80281=CARTESIAN_POINT('Ctrl Pts',(2.41077065550203,138.3460298843,14.2796976784835));
#80282=CARTESIAN_POINT('Ctrl Pts',(2.40940928043307,138.362535135864,14.2905164907587));
#80283=CARTESIAN_POINT('Ctrl Pts',(2.40291109855419,138.441712771649,14.3396168407627));
#80284=CARTESIAN_POINT('Ctrl Pts',(2.39758344690424,138.507595105554,14.3723907901521));
#80285=CARTESIAN_POINT('Ctrl Pts',(2.38723026835388,138.639206968591,14.4231653422949));
#80286=CARTESIAN_POINT('Ctrl Pts',(2.38223621736652,138.704310978394,14.4420338633483));
#80287=CARTESIAN_POINT('Ctrl Pts',(2.37648601230282,138.784121255699,14.4578770429948));
#80288=CARTESIAN_POINT('Ctrl Pts',(2.37552695144948,138.797609866748,14.4603108004324));
#80289=CARTESIAN_POINT('Ctrl Pts',(2.37402629816139,138.819043497177,14.4637929125631));
#80290=CARTESIAN_POINT('Ctrl Pts',(2.37347693170749,138.826961589692,14.4649965310344));
#80291=CARTESIAN_POINT('Ctrl Pts',(2.37239730849052,138.842676950449,14.4672216356913));
#80292=CARTESIAN_POINT('Ctrl Pts',(2.37186693858509,138.850473348529,14.4682459830209));
#80293=CARTESIAN_POINT('Ctrl Pts',(2.37047294911137,138.871147787263,14.4707519768697));
#80294=CARTESIAN_POINT('Ctrl Pts',(2.36961633097778,138.884041448505,14.4720992845166));
#80295=CARTESIAN_POINT('Ctrl Pts',(2.36481160582904,138.957245402524,14.478528758298));
#80296=CARTESIAN_POINT('Ctrl Pts',(2.36105569286795,139.017861469534,14.4791694998175));
#80297=CARTESIAN_POINT('Ctrl Pts',(2.35243766820181,139.156865156438,14.4699119157188));
#80298=CARTESIAN_POINT('Ctrl Pts',(2.34759513308405,139.234734817817,14.4568053851832));
#80299=CARTESIAN_POINT('Ctrl Pts',(2.34115013904538,139.331043419698,14.4304643649378));
#80300=CARTESIAN_POINT('Ctrl Pts',(2.33977452344838,139.351222484418,14.4243585300967));
#80301=CARTESIAN_POINT('Ctrl Pts',(2.33747566698884,139.384234683821,14.4133942098578));
#80302=CARTESIAN_POINT('Ctrl Pts',(2.3365626471314,139.397166569647,14.408846990365));
#80303=CARTESIAN_POINT('Ctrl Pts',(2.33473554987574,139.422669961128,14.3993759050918));
#80304=CARTESIAN_POINT('Ctrl Pts',(2.3338218382357,139.435242012673,14.3944595199405));
#80305=CARTESIAN_POINT('Ctrl Pts',(2.33154125650734,139.466155997043,14.3817535201762));
#80306=CARTESIAN_POINT('Ctrl Pts',(2.33016612931047,139.484389400856,14.3737126785111));
#80307=CARTESIAN_POINT('Ctrl Pts',(2.32376092596492,139.567412600211,14.3345546976335));
#80308=CARTESIAN_POINT('Ctrl Pts',(2.31854969547642,139.629463176611,14.2980148119132));
#80309=CARTESIAN_POINT('Ctrl Pts',(2.30820956986678,139.743847341394,14.2157266188255));
#80310=CARTESIAN_POINT('Ctrl Pts',(2.30310767114884,139.796254528154,14.1705424760453));
#80311=CARTESIAN_POINT('Ctrl Pts',(2.29726318606867,139.853912515423,14.1112426106492));
#80312=CARTESIAN_POINT('Ctrl Pts',(2.29630860946709,139.863252149824,14.1012970256901));
#80313=CARTESIAN_POINT('Ctrl Pts',(2.29481358382522,139.877785594431,14.0852715259833));
#80314=CARTESIAN_POINT('Ctrl Pts',(2.29426543952778,139.883093650073,14.0792974618079));
#80315=CARTESIAN_POINT('Ctrl Pts',(2.29319136909778,139.893461453587,14.0673868145198));
#80316=CARTESIAN_POINT('Ctrl Pts',(2.29266530742886,139.8985237803,14.0614531596122));
#80317=CARTESIAN_POINT('Ctrl Pts',(2.29128354858555,139.91176582025,14.0456159358502));
#80318=CARTESIAN_POINT('Ctrl Pts',(2.29043477776658,139.919843404728,14.0356277450894));
#80319=CARTESIAN_POINT('Ctrl Pts',(2.28853886649562,139.937707459874,14.0127837924098));
#80320=CARTESIAN_POINT('Ctrl Pts',(2.28749714922217,139.947396187672,13.9998546496914));
#80321=CARTESIAN_POINT('Ctrl Pts',(2.28405353974228,139.978854665698,13.9560237398922));
#80322=CARTESIAN_POINT('Ctrl Pts',(2.28170046311129,139.999403565874,13.9242727565533));
#80323=CARTESIAN_POINT('Ctrl Pts',(2.27388012267663,140.062867599536,13.81502216255));
#80324=CARTESIAN_POINT('Ctrl Pts',(2.26847548926846,140.098564180645,13.7336941031766));
#80325=CARTESIAN_POINT('Ctrl Pts',(2.26145351050725,140.130757100884,13.6299785591863));
#80326=CARTESIAN_POINT('Ctrl Pts',(2.26014254050079,140.13621304909,13.6106723356718));
#80327=CARTESIAN_POINT('Ctrl Pts',(2.25801419572744,140.144169297777,13.5794968534091));
#80328=CARTESIAN_POINT('Ctrl Pts',(2.25720705160607,140.146984056923,13.5677114633326));
#80329=CARTESIAN_POINT('Ctrl Pts',(2.25550066819096,140.152508754552,13.5428906244995));
#80330=CARTESIAN_POINT('Ctrl Pts',(2.25460033050362,140.155180468557,13.5298485249686));
#80331=CARTESIAN_POINT('Ctrl Pts',(2.25238244960284,140.161168304665,13.4978704807504));
#80332=CARTESIAN_POINT('Ctrl Pts',(2.2510574696775,140.164242878733,13.4788938286223));
#80333=CARTESIAN_POINT('Ctrl Pts',(2.24453588561216,140.176946797534,13.3861602685533));
#80334=CARTESIAN_POINT('Ctrl Pts',(2.2391399945279,140.180036989101,13.3116904380777));
#80335=CARTESIAN_POINT('Ctrl Pts',(2.22870469908476,140.172486848981,13.1697553418608));
#80336=CARTESIAN_POINT('Ctrl Pts',(2.22369890502352,140.163050232008,13.1025042048074));
#80337=CARTESIAN_POINT('Ctrl Pts',(2.21794038478802,140.144819201995,13.0231045165625));
#80338=CARTESIAN_POINT('Ctrl Pts',(2.21698306898224,140.141526405918,13.0098282935504));
#80339=CARTESIAN_POINT('Ctrl Pts',(2.21548604850883,140.135947360223,12.9889014113496));
#80340=CARTESIAN_POINT('Ctrl Pts',(2.21493855734802,140.133813423178,12.9812118760396));
#80341=CARTESIAN_POINT('Ctrl Pts',(2.21386072339937,140.129422060607,12.9659899860858));
#80342=CARTESIAN_POINT('Ctrl Pts',(2.2133302739426,140.127167033051,12.9584573687298));
#80343=CARTESIAN_POINT('Ctrl Pts',(2.21193853135526,140.121006181999,12.9386037546601));
#80344=CARTESIAN_POINT('Ctrl Pts',(2.21108417134733,140.116972579735,12.9263231390681));
#80345=CARTESIAN_POINT('Ctrl Pts',(2.20917584803252,140.107412486386,12.898755967871));
#80346=CARTESIAN_POINT('Ctrl Pts',(2.20812730575607,140.101770020611,12.8835122302565));
#80347=CARTESIAN_POINT('Ctrl Pts',(2.20465874539275,140.08186684179,12.8329801642291));
#80348=CARTESIAN_POINT('Ctrl Pts',(2.20228749641355,140.066211124872,12.7982654231828));
#80349=CARTESIAN_POINT('Ctrl Pts',(2.19450105713038,140.009062155612,12.68635352426));
#80350=CARTESIAN_POINT('Ctrl Pts',(2.18914401530618,139.960648532175,12.6130347060686));
#80351=CARTESIAN_POINT('Ctrl Pts',(2.18216845580539,139.891592326052,12.5302156380824));
#80352=CARTESIAN_POINT('Ctrl Pts',(2.1808450237708,139.878230628679,12.5150059084846));
#80353=CARTESIAN_POINT('Ctrl Pts',(2.17869562473881,139.85617144352,12.4911642030252));
#80354=CARTESIAN_POINT('Ctrl Pts',(2.17787995294451,139.847719351996,12.4823101025167));
#80355=CARTESIAN_POINT('Ctrl Pts',(2.17615414929313,139.829679767511,12.4639928404264));
#80356=CARTESIAN_POINT('Ctrl Pts',(2.17524288943651,139.820064896154,12.4545592702435));
#80357=CARTESIAN_POINT('Ctrl Pts',(2.1729936275348,139.796128752399,12.4318670091998));
#80358=CARTESIAN_POINT('Ctrl Pts',(2.17164800729215,139.781636098753,12.4187958179911));
#80359=CARTESIAN_POINT('Ctrl Pts',(2.16497177872032,139.708936910061,12.3564319094249));
#80360=CARTESIAN_POINT('Ctrl Pts',(2.15943391124451,139.646369881718,12.3125210332979));
#80361=CARTESIAN_POINT('Ctrl Pts',(2.14910595607752,139.523863190429,12.2432009689591));
#80362=CARTESIAN_POINT('Ctrl Pts',(2.14435391962411,139.465197206728,12.2160951855371));
#80363=CARTESIAN_POINT('Ctrl Pts',(2.13879798874671,139.391393542256,12.1890976716974));
#80364=CARTESIAN_POINT('Ctrl Pts',(2.13781337941443,139.378098282155,12.1845025233635));
#80365=CARTESIAN_POINT('Ctrl Pts',(2.13627988467631,139.357002187677,12.1776317726565));
#80366=CARTESIAN_POINT('Ctrl Pts',(2.1357227967925,139.349255097007,12.1751969564406));
#80367=CARTESIAN_POINT('Ctrl Pts',(2.13462845607441,139.333858820776,12.1705325076397));
#80368=CARTESIAN_POINT('Ctrl Pts',(2.13409105683266,139.326210966168,12.1682999764697));
#80369=CARTESIAN_POINT('Ctrl Pts',(2.13268129110015,139.305936539197,12.1626041578633));
#80370=CARTESIAN_POINT('Ctrl Pts',(2.13181592933848,139.293273497132,12.1592734077159));
#80371=CARTESIAN_POINT('Ctrl Pts',(2.12728516373587,139.225994317005,12.1427714965815));
#80372=CARTESIAN_POINT('Ctrl Pts',(2.12378034255749,139.170537653335,12.1333082816886));
#80373=CARTESIAN_POINT('Ctrl Pts',(2.11525682551867,139.033868034591,12.1199449508485));
#80374=CARTESIAN_POINT('Ctrl Pts',(2.11026701857196,138.952532233442,12.1204143121773));
#80375=CARTESIAN_POINT('Ctrl Pts',(2.10368943184909,138.851417175468,12.1314785018599));
#80376=CARTESIAN_POINT('Ctrl Pts',(2.10234335522298,138.831004583655,12.1342556820317));
#80377=CARTESIAN_POINT('Ctrl Pts',(2.10007501371621,138.797160654769,12.1397677908201));
#80378=CARTESIAN_POINT('Ctrl Pts',(2.09916210251997,138.78368498598,12.1422045226007));
#80379=CARTESIAN_POINT('Ctrl Pts',(2.0973191559252,138.756792773886,12.1475531606829));
#80380=CARTESIAN_POINT('Ctrl Pts',(2.09638922911049,138.743378577313,12.150465794256));
#80381=CARTESIAN_POINT('Ctrl Pts',(2.09403383361451,138.709809894335,12.1583714189739));
#80382=CARTESIAN_POINT('Ctrl Pts',(2.09259909307004,138.689731540893,12.1636640008672));
#80383=CARTESIAN_POINT('Ctrl Pts',(2.08941622219356,138.646019822059,12.1764311005241));
#80384=CARTESIAN_POINT('Ctrl Pts',(2.08766193247673,138.622461733889,12.1841264637165));
#80385=CARTESIAN_POINT('Ctrl Pts',(2.07854696123358,138.502726554575,12.2274642197546));
#80386=CARTESIAN_POINT('Ctrl Pts',(2.07086395863705,138.41127481782,12.2748109570225));
#80387=CARTESIAN_POINT('Ctrl Pts',(2.06349999999998,138.327116518419,12.3333962121349));
#80388=CARTESIAN_POINT('',(2.0635,139.684664424539,12.3417048010816));
#80389=CARTESIAN_POINT('Origin',(2.0635,139.,13.3));
#80390=CARTESIAN_POINT('Ctrl Pts',(2.06349999999976,139.684664424539,12.3417048010814));
#80391=CARTESIAN_POINT('Ctrl Pts',(2.06413207243538,139.692276025771,12.3471429923432));
#80392=CARTESIAN_POINT('Ctrl Pts',(2.06475846007851,139.699814794663,12.3526659312376));
#80393=CARTESIAN_POINT('Ctrl Pts',(2.06626808273718,139.717950082849,12.3662868168646));
#80394=CARTESIAN_POINT('Ctrl Pts',(2.06714603508711,139.728468797957,12.374469952678));
#80395=CARTESIAN_POINT('Ctrl Pts',(2.0715132138531,139.780513105435,12.4163954144151));
#80396=CARTESIAN_POINT('Ctrl Pts',(2.07489099690678,139.819847070126,12.4527636475568));
#80397=CARTESIAN_POINT('Ctrl Pts',(2.08230577647004,139.900562164323,12.5382974931292));
#80398=CARTESIAN_POINT('Ctrl Pts',(2.08633185582837,139.940669195938,12.588421714189));
#80399=CARTESIAN_POINT('Ctrl Pts',(2.09201028102551,139.989650974106,12.6610637734024));
#80400=CARTESIAN_POINT('Ctrl Pts',(2.09355018068357,140.002215711147,12.6809587124619));
#80401=CARTESIAN_POINT('Ctrl Pts',(2.09611575615856,140.021896338493,12.7142922723833));
#80402=CARTESIAN_POINT('Ctrl Pts',(2.09712994397898,140.029363050064,12.7275165091744));
#80403=CARTESIAN_POINT('Ctrl Pts',(2.09916946998459,140.043740119151,12.754170696032));
#80404=CARTESIAN_POINT('Ctrl Pts',(2.10019451974577,140.050651981217,12.767596538696));
#80405=CARTESIAN_POINT('Ctrl Pts',(2.10279087435359,140.067360811613,12.8016455744444));
#80406=CARTESIAN_POINT('Ctrl Pts',(2.10437266492368,140.076819414721,12.8224269023685));
#80407=CARTESIAN_POINT('Ctrl Pts',(2.11222247014196,140.120210322204,12.9256139468685));
#80408=CARTESIAN_POINT('Ctrl Pts',(2.11876461733174,140.145312735583,13.011400775157));
#80409=CARTESIAN_POINT('Ctrl Pts',(2.13001082082233,140.171256861151,13.1613263014646));
#80410=CARTESIAN_POINT('Ctrl Pts',(2.13466710424179,140.177002791467,13.2242435825927));
#80411=CARTESIAN_POINT('Ctrl Pts',(2.14005074624944,140.177822454712,13.300392861075));
#80412=CARTESIAN_POINT('Ctrl Pts',(2.1409657211342,140.177745574321,13.3134643170549));
#80413=CARTESIAN_POINT('Ctrl Pts',(2.14241951757392,140.177271994475,13.3344807262676));
#80414=CARTESIAN_POINT('Ctrl Pts',(2.14296523071435,140.177012406725,13.3424272709685));
#80415=CARTESIAN_POINT('Ctrl Pts',(2.14403999052804,140.176337051815,13.3582036799551));
#80416=CARTESIAN_POINT('Ctrl Pts',(2.14456903170626,140.175923540063,13.3660330204332));
#80417=CARTESIAN_POINT('Ctrl Pts',(2.14598272575006,140.174599359911,13.3871070701734));
#80418=CARTESIAN_POINT('Ctrl Pts',(2.1468596103102,140.17354284871,13.4003420054723));
#80419=CARTESIAN_POINT('Ctrl Pts',(2.15231803634139,140.165485612026,13.4835178808387));
#80420=CARTESIAN_POINT('Ctrl Pts',(2.15663328603,140.152458270382,13.5527409858127));
#80421=CARTESIAN_POINT('Ctrl Pts',(2.16529624695658,140.114293047057,13.68774228311));
#80422=CARTESIAN_POINT('Ctrl Pts',(2.16962937644036,140.089291502112,13.7532500846333));
#80423=CARTESIAN_POINT('Ctrl Pts',(2.17539110814622,140.050281864033,13.8332592998947));
#80424=CARTESIAN_POINT('Ctrl Pts',(2.17663621255472,140.041525625264,13.8501652284155));
#80425=CARTESIAN_POINT('Ctrl Pts',(2.1787566843611,140.026104282296,13.8782509944093));
#80426=CARTESIAN_POINT('Ctrl Pts',(2.17962407072749,140.019656467382,13.889546330235));
#80427=CARTESIAN_POINT('Ctrl Pts',(2.18138981032915,140.006261303003,13.9121347843412));
#80428=CARTESIAN_POINT('Ctrl Pts',(2.18228830853187,139.999307683292,13.9234219536115));
#80429=CARTESIAN_POINT('Ctrl Pts',(2.18458701174971,139.981182154403,13.951760802839));
#80430=CARTESIAN_POINT('Ctrl Pts',(2.18599685241096,139.969755755006,13.9686435862105));
#80431=CARTESIAN_POINT('Ctrl Pts',(2.19368597685254,139.905832308907,14.0580047812989));
#80432=CARTESIAN_POINT('Ctrl Pts',(2.20027555257896,139.845649928336,14.1246052346611));
#80433=CARTESIAN_POINT('Ctrl Pts',(2.21122798441851,139.7344934079,14.2225279832514));
#80434=CARTESIAN_POINT('Ctrl Pts',(2.21555282743687,139.687619651618,14.2579765791127));
#80435=CARTESIAN_POINT('Ctrl Pts',(2.22053519540554,139.628252999963,14.2962609999035));
#80436=CARTESIAN_POINT('Ctrl Pts',(2.22136977755323,139.618113556419,14.3025833995454));
#80437=CARTESIAN_POINT('Ctrl Pts',(2.22271079299268,139.601473834201,14.3126105943606));
#80438=CARTESIAN_POINT('Ctrl Pts',(2.22322308167965,139.595031759257,14.3164094682078));
#80439=CARTESIAN_POINT('Ctrl Pts',(2.22427832534028,139.581579256063,14.3241706199419));
#80440=CARTESIAN_POINT('Ctrl Pts',(2.22482070539569,139.574563810906,14.3281227196552));
#80441=CARTESIAN_POINT('Ctrl Pts',(2.22628572417675,139.555356986974,14.3386847352448));
#80442=CARTESIAN_POINT('Ctrl Pts',(2.22719998283471,139.543088118983,14.3451519979256));
#80443=CARTESIAN_POINT('Ctrl Pts',(2.23238903180733,139.472031978979,14.3810184213317));
#80444=CARTESIAN_POINT('Ctrl Pts',(2.23644148188335,139.410973121126,14.4056754410378));
#80445=CARTESIAN_POINT('Ctrl Pts',(2.24510756763881,139.276929959089,14.4471555727982));
#80446=CARTESIAN_POINT('Ctrl Pts',(2.24971002566705,139.203765534783,14.4623829840665));
#80447=CARTESIAN_POINT('Ctrl Pts',(2.25585498591522,139.109273320645,14.4728490839006));
#80448=CARTESIAN_POINT('Ctrl Pts',(2.25719482552104,139.088835756897,14.4745738625621));
#80449=CARTESIAN_POINT('Ctrl Pts',(2.25945995909053,139.054645455405,14.476561849671));
#80450=CARTESIAN_POINT('Ctrl Pts',(2.2603760186917,139.040913980292,14.4771193360399));
#80451=CARTESIAN_POINT('Ctrl Pts',(2.26223090317901,139.013323248518,14.4777561567112));
#80452=CARTESIAN_POINT('Ctrl Pts',(2.26316970638875,138.999466102471,14.4778313802513));
#80453=CARTESIAN_POINT('Ctrl Pts',(2.26556139801454,138.96445252382,14.4774035850751));
#80454=CARTESIAN_POINT('Ctrl Pts',(2.26702400649114,138.943305768658,14.4765748978057));
#80455=CARTESIAN_POINT('Ctrl Pts',(2.2737518499631,138.847279805774,14.4702172154917));
#80456=CARTESIAN_POINT('Ctrl Pts',(2.27920927473163,138.773022258433,14.4581060911347));
#80457=CARTESIAN_POINT('Ctrl Pts',(2.28784152407662,138.65902399702,14.428124024552));
#80458=CARTESIAN_POINT('Ctrl Pts',(2.29097993590114,138.618237303402,14.4149825016667));
#80459=CARTESIAN_POINT('Ctrl Pts',(2.29531233963049,138.562037334715,14.3934283182496));
#80460=CARTESIAN_POINT('Ctrl Pts',(2.2965526426546,138.54595786279,14.3868498430392));
#80461=CARTESIAN_POINT('Ctrl Pts',(2.29873849430818,138.51755119602,14.3744875049502));
#80462=CARTESIAN_POINT('Ctrl Pts',(2.29968952716099,138.505167731833,14.3688411070798));
#80463=CARTESIAN_POINT('Ctrl Pts',(2.3011885533406,138.485569742248,14.3594915062799));
#80464=CARTESIAN_POINT('Ctrl Pts',(2.30174392208495,138.478291139038,14.3559264254956));
#80465=CARTESIAN_POINT('Ctrl Pts',(2.30284396359321,138.463827158832,14.3486558501001));
#80466=CARTESIAN_POINT('Ctrl Pts',(2.30338859513916,138.456642025645,14.3449509686713));
#80467=CARTESIAN_POINT('Ctrl Pts',(2.30484681387049,138.437359100049,14.3347554041012));
#80468=CARTESIAN_POINT('Ctrl Pts',(2.3057524089987,138.4253352836,14.3281264670286));
#80469=CARTESIAN_POINT('Ctrl Pts',(2.31113667315481,138.35377327029,14.2870252821611));
#80470=CARTESIAN_POINT('Ctrl Pts',(2.31537294259488,138.297226435663,14.2475966902402));
#80471=CARTESIAN_POINT('Ctrl Pts',(2.32266531069903,138.206778066183,14.1719544603465));
#80472=CARTESIAN_POINT('Ctrl Pts',(2.32570361507321,138.171123362906,14.1381340913705));
#80473=CARTESIAN_POINT('Ctrl Pts',(2.33027701625526,138.121939579175,14.0852638658834));
#80474=CARTESIAN_POINT('Ctrl Pts',(2.33175537515584,138.106696874624,14.0678794635745));
#80475=CARTESIAN_POINT('Ctrl Pts',(2.33453026448093,138.079415915783,14.0348530302698));
#80476=CARTESIAN_POINT('Ctrl Pts',(2.3358211561055,138.067240177319,14.0193351597679));
#80477=CARTESIAN_POINT('Ctrl Pts',(2.33802583763286,138.047355667512,13.9926383796948));
#80478=CARTESIAN_POINT('Ctrl Pts',(2.3389314363825,138.039439950873,13.9816183061784));
#80479=CARTESIAN_POINT('Ctrl Pts',(2.3406725046085,138.0247108208,13.9603465233313));
#80480=CARTESIAN_POINT('Ctrl Pts',(2.34150656079126,138.017864251657,13.9501198857444));
#80481=CARTESIAN_POINT('Ctrl Pts',(2.34373310838499,138.000146681057,13.9227366056069));
#80482=CARTESIAN_POINT('Ctrl Pts',(2.34513565670164,137.989557499316,13.9054035044915));
#80483=CARTESIAN_POINT('Ctrl Pts',(2.35181427384127,137.941826054495,13.8225298473835));
#80484=CARTESIAN_POINT('Ctrl Pts',(2.35728795971268,137.910598130773,13.7538297741315));
#80485=CARTESIAN_POINT('Ctrl Pts',(2.36281347991194,137.88614819712,13.6826607161973));
#80486=CARTESIAN_POINT('Origin',(1.13913288526384,139.,13.3));
#80487=CARTESIAN_POINT('',(2.96251705962155,137.886148212658,13.6826607614251));
#80488=CARTESIAN_POINT('',(2.86376176824067,137.886148209742,13.6826607529367));
#80489=CARTESIAN_POINT('',(1.13913288526384,137.88614821265,13.6826607614027));
#80490=CARTESIAN_POINT('Ctrl Pts',(2.96251705962155,137.886148212665,13.6826607614475));
#80491=CARTESIAN_POINT('Ctrl Pts',(2.95646427638088,137.914303066403,13.7646141188798));
#80492=CARTESIAN_POINT('Ctrl Pts',(2.95012116491658,137.951412599125,13.8431978452712));
#80493=CARTESIAN_POINT('Ctrl Pts',(2.94094865633092,138.016846374047,13.9495915135337));
#80494=CARTESIAN_POINT('Ctrl Pts',(2.93814404898771,138.038477049007,13.9812004767065));
#80495=CARTESIAN_POINT('Ctrl Pts',(2.93421783410981,138.071450872807,14.0246770331796));
#80496=CARTESIAN_POINT('Ctrl Pts',(2.93305563758885,138.081560683279,14.0374480041505));
#80497=CARTESIAN_POINT('Ctrl Pts',(2.93099474864767,138.10016896321,14.059977926502));
#80498=CARTESIAN_POINT('Ctrl Pts',(2.93009120527257,138.108569459425,14.0698142436267));
#80499=CARTESIAN_POINT('Ctrl Pts',(2.92865679132281,138.122323516098,14.0853920087352));
#80500=CARTESIAN_POINT('Ctrl Pts',(2.92811919652302,138.127575181228,14.0912215644773));
#80501=CARTESIAN_POINT('Ctrl Pts',(2.92704265943291,138.138296328096,14.1028859131977));
#80502=CARTESIAN_POINT('Ctrl Pts',(2.92650389367022,138.143767735551,14.1087183233468));
#80503=CARTESIAN_POINT('Ctrl Pts',(2.9250555123353,138.158750749254,14.1243673801587));
#80504=CARTESIAN_POINT('Ctrl Pts',(2.92415395412031,138.168374824719,14.1340752285838));
#80505=CARTESIAN_POINT('Ctrl Pts',(2.91879091357252,138.227262727787,14.1914427888018));
#80506=CARTESIAN_POINT('Ctrl Pts',(2.91457257147433,138.280447035369,14.2349005065517));
#80507=CARTESIAN_POINT('Ctrl Pts',(2.90727758395957,138.378028587346,14.3013473983221));
#80508=CARTESIAN_POINT('Ctrl Pts',(2.90421788048289,138.420655381496,14.3265984975157));
#80509=CARTESIAN_POINT('Ctrl Pts',(2.89961986449765,138.485371650327,14.3596174241781));
#80510=CARTESIAN_POINT('Ctrl Pts',(2.89813975559793,138.506306109645,14.3695315181162));
#80511=CARTESIAN_POINT('Ctrl Pts',(2.89536475165503,138.545568622493,14.3867269639389));
#80512=CARTESIAN_POINT('Ctrl Pts',(2.89407561786099,138.563813584067,14.3941776400951));
#80513=CARTESIAN_POINT('Ctrl Pts',(2.89188108521518,138.594808206175,14.4059364728599));
#80514=CARTESIAN_POINT('Ctrl Pts',(2.89098401695126,138.607460677712,14.410490309218));
#80515=CARTESIAN_POINT('Ctrl Pts',(2.88915629679668,138.633183899496,14.4192539973092));
#80516=CARTESIAN_POINT('Ctrl Pts',(2.88822547886479,138.6462558124,14.4234538637689));
#80517=CARTESIAN_POINT('Ctrl Pts',(2.88583351993616,138.679756063075,14.4335745119744));
#80518=CARTESIAN_POINT('Ctrl Pts',(2.88436222385205,138.700276055443,14.4391719835894));
#80519=CARTESIAN_POINT('Ctrl Pts',(2.87752814097923,138.795141304597,14.4623089394183));
#80520=CARTESIAN_POINT('Ctrl Pts',(2.87196243263017,138.870920950121,14.4731429258473));
#80521=CARTESIAN_POINT('Ctrl Pts',(2.86312578182455,138.991108701895,14.478536211947));
#80522=CARTESIAN_POINT('Ctrl Pts',(2.85989427780272,139.035092070729,14.4780473327829));
#80523=CARTESIAN_POINT('Ctrl Pts',(2.85545500363692,139.096489825624,14.4739224532959));
#80524=CARTESIAN_POINT('Ctrl Pts',(2.85419700888376,139.114005294646,14.4723510863785));
#80525=CARTESIAN_POINT('Ctrl Pts',(2.85198700728598,139.14508170287,14.4688600030221));
#80526=CARTESIAN_POINT('Ctrl Pts',(2.85102913643867,139.158656616601,14.4670949086401));
#80527=CARTESIAN_POINT('Ctrl Pts',(2.8495301914702,139.180113010494,14.4639236983597));
#80528=CARTESIAN_POINT('Ctrl Pts',(2.84898135787315,139.188015807698,14.4626732721216));
#80529=CARTESIAN_POINT('Ctrl Pts',(2.84790362175273,139.203639071181,14.4600378013745));
#80530=CARTESIAN_POINT('Ctrl Pts',(2.84737459876056,139.211359604073,14.458655987293));
#80531=CARTESIAN_POINT('Ctrl Pts',(2.84598491146719,139.231758263538,14.4547943699576));
#80532=CARTESIAN_POINT('Ctrl Pts',(2.84513121119135,139.244410804899,14.4521828510139));
#80533=CARTESIAN_POINT('Ctrl Pts',(2.83930804671342,139.331323913121,14.4327475100138));
#80534=CARTESIAN_POINT('Ctrl Pts',(2.83464826567873,139.403852941535,14.4089627125076));
#80535=CARTESIAN_POINT('Ctrl Pts',(2.82711638647817,139.515392998031,14.3599764965389));
#80536=CARTESIAN_POINT('Ctrl Pts',(2.82428398209048,139.556095966834,14.3392001837738));
#80537=CARTESIAN_POINT('Ctrl Pts',(2.81998207717441,139.614619769986,14.3049026469251));
#80538=CARTESIAN_POINT('Ctrl Pts',(2.81856210774795,139.633430018696,14.2931531174113));
#80539=CARTESIAN_POINT('Ctrl Pts',(2.8158869145189,139.667792776651,14.270315500188));
#80540=CARTESIAN_POINT('Ctrl Pts',(2.81463670508925,139.683428989856,14.259366515478));
#80541=CARTESIAN_POINT('Ctrl Pts',(2.8124882130804,139.709530642263,14.240127286651));
#80542=CARTESIAN_POINT('Ctrl Pts',(2.81159743286672,139.720134041103,14.2320300346127));
#80543=CARTESIAN_POINT('Ctrl Pts',(2.80976504738042,139.741486455576,14.215142417727));
#80544=CARTESIAN_POINT('Ctrl Pts',(2.80882299533033,139.752222102584,14.2063386167127));
#80545=CARTESIAN_POINT('Ctrl Pts',(2.80636219022813,139.779627715741,14.1830421986584));
#80546=CARTESIAN_POINT('Ctrl Pts',(2.80483207943284,139.796049399458,14.1682673201443));
#80547=CARTESIAN_POINT('Ctrl Pts',(2.79596435802696,139.887663566981,14.0810559285882));
#80548=CARTESIAN_POINT('Ctrl Pts',(2.78821814302433,139.953365569953,13.9993436884224));
#80549=CARTESIAN_POINT('Ctrl Pts',(2.77876875349182,140.020489283649,13.8885002619602));
#80550=CARTESIAN_POINT('Ctrl Pts',(2.77694338091867,140.032856017517,13.8665152494277));
#80551=CARTESIAN_POINT('Ctrl Pts',(2.77388139473684,140.052696169122,13.8284315674735));
#80552=CARTESIAN_POINT('Ctrl Pts',(2.77263146660674,140.060529080949,13.8125302875807));
#80553=CARTESIAN_POINT('Ctrl Pts',(2.77079016566074,140.071704948047,13.7884882744695));
#80554=CARTESIAN_POINT('Ctrl Pts',(2.77018456005063,140.07532015996,13.7804777369926));
#80555=CARTESIAN_POINT('Ctrl Pts',(2.76907479188195,140.081838118129,13.7655931784909));
#80556=CARTESIAN_POINT('Ctrl Pts',(2.76856931279198,140.084765579221,13.7587312538943));
#80557=CARTESIAN_POINT('Ctrl Pts',(2.76734605272378,140.091744339827,13.7419326728629));
#80558=CARTESIAN_POINT('Ctrl Pts',(2.76663230603118,140.095725385821,13.7319676960192));
#80559=CARTESIAN_POINT('Ctrl Pts',(2.763837912919,140.110918673227,13.6923750661017));
#80560=CARTESIAN_POINT('Ctrl Pts',(2.76180972217653,140.121070782741,13.6623522576163));
#80561=CARTESIAN_POINT('Ctrl Pts',(2.7555091423141,140.149233394899,13.5664842484062));
#80562=CARTESIAN_POINT('Ctrl Pts',(2.75135332240071,140.162740684014,13.4994646764901));
#80563=CARTESIAN_POINT('Ctrl Pts',(2.74606215449591,140.172244708905,13.4149739945561));
#80564=CARTESIAN_POINT('Ctrl Pts',(2.74501340583822,140.173763873846,13.3982599705989));
#80565=CARTESIAN_POINT('Ctrl Pts',(2.74161964085247,140.1774976719,13.3444454654854));
#80566=CARTESIAN_POINT('Ctrl Pts',(2.73924862467719,140.178313569384,13.3072735012378));
#80567=CARTESIAN_POINT('Ctrl Pts',(2.73573465045298,140.176947063702,13.2534150163207));
#80568=CARTESIAN_POINT('Ctrl Pts',(2.73463417971304,140.176167251754,13.2367141328168));
#80569=CARTESIAN_POINT('Ctrl Pts',(2.73265520278804,140.174146518575,13.207020373354));
#80570=CARTESIAN_POINT('Ctrl Pts',(2.73178116875128,140.173044591831,13.1940206614416));
#80571=CARTESIAN_POINT('Ctrl Pts',(2.72990781827039,140.170242429182,13.166419492816));
#80572=CARTESIAN_POINT('Ctrl Pts',(2.72890682441286,140.168484323683,13.151826297632));
#80573=CARTESIAN_POINT('Ctrl Pts',(2.7260808992278,140.162800178642,13.11108207491));
#80574=CARTESIAN_POINT('Ctrl Pts',(2.72423742540446,140.158266078932,13.0850261977428));
#80575=CARTESIAN_POINT('Ctrl Pts',(2.71554413255922,140.133109548212,12.9646129095003));
#80576=CARTESIAN_POINT('Ctrl Pts',(2.70837759843094,140.101808294031,12.8728758460773));
#80577=CARTESIAN_POINT('Ctrl Pts',(2.69870720917318,140.043930321278,12.7535516889008));
#80578=CARTESIAN_POINT('Ctrl Pts',(2.69610461206466,140.026703374677,12.7218331269415));
#80579=CARTESIAN_POINT('Ctrl Pts',(2.69276029577135,140.00207914963,12.681077085518));
#80580=CARTESIAN_POINT('Ctrl Pts',(2.6919571582432,139.995967247938,12.6712890467248));
#80581=CARTESIAN_POINT('Ctrl Pts',(2.6906458910845,139.985642919904,12.6552834317038));
#80582=CARTESIAN_POINT('Ctrl Pts',(2.69013278603232,139.9815132273,12.6490136586495));
#80583=CARTESIAN_POINT('Ctrl Pts',(2.68905528701246,139.972644951077,12.6358259588382));
#80584=CARTESIAN_POINT('Ctrl Pts',(2.68849183153208,139.967891984953,12.6289184297513));
#80585=CARTESIAN_POINT('Ctrl Pts',(2.68689328005565,139.95408979238,12.6093113049842));
#80586=CARTESIAN_POINT('Ctrl Pts',(2.68586930428567,139.944861241485,12.5967393823012));
#80587=CARTESIAN_POINT('Ctrl Pts',(2.68349261644428,139.92260433705,12.5676485030669));
#80588=CARTESIAN_POINT('Ctrl Pts',(2.68215023481727,139.909377519702,12.5512877034403));
#80589=CARTESIAN_POINT('Ctrl Pts',(2.67684015034007,139.854776040291,12.4873320624687));
#80590=CARTESIAN_POINT('Ctrl Pts',(2.67298891306041,139.810046183845,12.4427385488402));
#80591=CARTESIAN_POINT('Ctrl Pts',(2.66557615801517,139.718945518702,12.3654442474519));
#80592=CARTESIAN_POINT('Ctrl Pts',(2.66203676676584,139.673370213679,12.3320905920249));
#80593=CARTESIAN_POINT('Ctrl Pts',(2.65717130904673,139.609879379389,12.2922868569744));
#80594=CARTESIAN_POINT('Ctrl Pts',(2.65595576476691,139.593945200348,12.2828138454466));
#80595=CARTESIAN_POINT('Ctrl Pts',(2.65384787932054,139.566246960718,12.267219740887));
#80596=CARTESIAN_POINT('Ctrl Pts',(2.65296232148721,139.554590618507,12.2609139084754));
#80597=CARTESIAN_POINT('Ctrl Pts',(2.65112351693161,139.530364629532,12.2483319230294));
#80598=CARTESIAN_POINT('Ctrl Pts',(2.65016954817143,139.517784172462,12.2420813333175));
#80599=CARTESIAN_POINT('Ctrl Pts',(2.6476358947917,139.484359447224,12.2262133007545));
#80600=CARTESIAN_POINT('Ctrl Pts',(2.64604353078672,139.463341503351,12.2169780827989));
#80601=CARTESIAN_POINT('Ctrl Pts',(2.63904814699702,139.371015738573,12.1795899085017));
#80602=CARTESIAN_POINT('Ctrl Pts',(2.63344720661547,139.297333456835,12.1578262082442));
#80603=CARTESIAN_POINT('Ctrl Pts',(2.6233513268985,139.162357044138,12.131910712448));
#80604=CARTESIAN_POINT('Ctrl Pts',(2.61888690131824,139.101838166796,12.1250860651044));
#80605=CARTESIAN_POINT('Ctrl Pts',(2.61374785087651,139.028862343082,12.1225404692164));
#80606=CARTESIAN_POINT('Ctrl Pts',(2.61289690439158,139.016660029395,12.1223046002309));
#80607=CARTESIAN_POINT('Ctrl Pts',(2.6115768950797,138.997511803851,12.1222321581758));
#80608=CARTESIAN_POINT('Ctrl Pts',(2.61110134948665,138.990567612995,12.122267298177));
#80609=CARTESIAN_POINT('Ctrl Pts',(2.61009009270014,138.975693367215,12.1224741379759));
#80610=CARTESIAN_POINT('Ctrl Pts',(2.60955545845676,138.967763852686,12.1226645303241));
#80611=CARTESIAN_POINT('Ctrl Pts',(2.60813233657684,138.946500278861,12.1233900789607));
#80612=CARTESIAN_POINT('Ctrl Pts',(2.60725142571311,138.933171975335,12.1240717799075));
#80613=CARTESIAN_POINT('Ctrl Pts',(2.60527078173857,138.902910402694,12.1261357782268));
#80614=CARTESIAN_POINT('Ctrl Pts',(2.60417715766075,138.885989467951,12.1276582161223));
#80615=CARTESIAN_POINT('Ctrl Pts',(2.60046542407353,138.828100590766,12.13413200809));
#80616=CARTESIAN_POINT('Ctrl Pts',(2.59790383431498,138.787361331258,12.140869810963));
#80617=CARTESIAN_POINT('Ctrl Pts',(2.59034158179797,138.667967260764,12.1671244168521));
#80618=CARTESIAN_POINT('Ctrl Pts',(2.58537165666007,138.590889263896,12.1926248313139));
#80619=CARTESIAN_POINT('Ctrl Pts',(2.5787934169404,138.497965454653,12.2344045145641));
#80620=CARTESIAN_POINT('Ctrl Pts',(2.57742838146803,138.47912434219,12.2434864478856));
#80621=CARTESIAN_POINT('Ctrl Pts',(2.57514297570203,138.448388001399,12.2593242492612));
#80622=CARTESIAN_POINT('Ctrl Pts',(2.57423261405881,138.436350451406,12.2657945199197));
#80623=CARTESIAN_POINT('Ctrl Pts',(2.57240777441562,138.412647480277,12.2790717825479));
#80624=CARTESIAN_POINT('Ctrl Pts',(2.57149361126972,138.400981153039,12.2858728865739));
#80625=CARTESIAN_POINT('Ctrl Pts',(2.56920604004584,138.372316469135,12.3032506919806));
#80626=CARTESIAN_POINT('Ctrl Pts',(2.56782422807919,138.355466542002,12.3140627129904));
#80627=CARTESIAN_POINT('Ctrl Pts',(2.56104135236056,138.275038526765,12.3686136249284));
#80628=CARTESIAN_POINT('Ctrl Pts',(2.5554277968484,138.215597506304,12.4180936589112));
#80629=CARTESIAN_POINT('Ctrl Pts',(2.54516716506433,138.117493759442,12.517572295702));
#80630=CARTESIAN_POINT('Ctrl Pts',(2.54055902904284,138.077174286213,12.5655585181767));
#80631=CARTESIAN_POINT('Ctrl Pts',(2.53513126941458,138.032653893176,12.6280354518401));
#80632=CARTESIAN_POINT('Ctrl Pts',(2.53414114286161,138.024658780827,12.6396937113549));
#80633=CARTESIAN_POINT('Ctrl Pts',(2.53260395005526,138.012419215598,12.6582486921008));
#80634=CARTESIAN_POINT('Ctrl Pts',(2.53204848415557,138.008032940814,12.665049678961));
#80635=CARTESIAN_POINT('Ctrl Pts',(2.53096927703127,137.999576441104,12.6784631610406));
#80636=CARTESIAN_POINT('Ctrl Pts',(2.53044525326067,137.995500885975,12.6850716507389));
#80637=CARTESIAN_POINT('Ctrl Pts',(2.52908539718374,137.985015539958,12.7024560283014));
#80638=CARTESIAN_POINT('Ctrl Pts',(2.5282559990971,137.978711719937,12.7132951911438));
#80639=CARTESIAN_POINT('Ctrl Pts',(2.52641263751658,137.964945637128,12.7378598759104));
#80640=CARTESIAN_POINT('Ctrl Pts',(2.52540359728806,137.957580854063,12.7516375058554));
#80641=CARTESIAN_POINT('Ctrl Pts',(2.5221279857152,137.934337645941,12.7972812673542));
#80642=CARTESIAN_POINT('Ctrl Pts',(2.51990488982002,137.919628879312,12.8297224923258));
#80643=CARTESIAN_POINT('Ctrl Pts',(2.51194043115319,137.871957632597,12.9489598685272));
#80644=CARTESIAN_POINT('Ctrl Pts',(2.50628575698445,137.847813491294,13.0388994043874));
#80645=CARTESIAN_POINT('Ctrl Pts',(2.49901509361655,137.831683349772,13.1499701873584));
#80646=CARTESIAN_POINT('Ctrl Pts',(2.4977430908007,137.829366964721,13.169267579232));
#80647=CARTESIAN_POINT('Ctrl Pts',(2.49557808838465,137.826275003925,13.2018137492617));
#80648=CARTESIAN_POINT('Ctrl Pts',(2.49469319961711,137.825243950473,13.2150346778205));
#80649=CARTESIAN_POINT('Ctrl Pts',(2.49287625974316,137.823598863839,13.241995465887));
#80650=CARTESIAN_POINT('Ctrl Pts',(2.4919438184932,137.823001837056,13.255734261437));
#80651=CARTESIAN_POINT('Ctrl Pts',(2.489539971741,137.822090615859,13.2908858258664));
#80652=CARTESIAN_POINT('Ctrl Pts',(2.48805818800391,137.822119636331,13.3123016249424));
#80653=CARTESIAN_POINT('Ctrl Pts',(2.48214734766849,137.824535676554,13.3966940542107));
#80654=CARTESIAN_POINT('Ctrl Pts',(2.47758840895213,137.831391287714,13.459429453727));
#80655=CARTESIAN_POINT('Ctrl Pts',(2.46888627835354,137.853704825262,13.5760620385627));
#80656=CARTESIAN_POINT('Ctrl Pts',(2.46477007283849,137.868050284058,13.6299811763935));
#80657=CARTESIAN_POINT('Ctrl Pts',(2.46074688473191,137.88614821265,13.6826607614027));
#80658=CARTESIAN_POINT('Ctrl Pts',(2.36281347991194,137.88614819712,13.6826607161973));
#80659=CARTESIAN_POINT('Ctrl Pts',(2.36370494271238,137.882203553803,13.6711786176069));
#80660=CARTESIAN_POINT('Ctrl Pts',(2.36459733014602,137.878435320883,13.6596322255798));
#80661=CARTESIAN_POINT('Ctrl Pts',(2.36828519000139,137.863595032016,13.6116540706226));
#80662=CARTESIAN_POINT('Ctrl Pts',(2.37107428274278,137.854114502947,13.5747566644989));
#80663=CARTESIAN_POINT('Ctrl Pts',(2.37498502668362,137.843155181419,13.521517850011));
#80664=CARTESIAN_POINT('Ctrl Pts',(2.37614673066806,137.840203586683,13.5055052918271));
#80665=CARTESIAN_POINT('Ctrl Pts',(2.37820869752349,137.83550089769,13.4766486884019));
#80666=CARTESIAN_POINT('Ctrl Pts',(2.37911376202389,137.833628026566,13.4638272654617));
#80667=CARTESIAN_POINT('Ctrl Pts',(2.3805534315095,137.830954285057,13.443141860933));
#80668=CARTESIAN_POINT('Ctrl Pts',(2.38109472504524,137.83002036977,13.4352965275862));
#80669=CARTESIAN_POINT('Ctrl Pts',(2.38217850131203,137.828294316822,13.4194389535477));
#80670=CARTESIAN_POINT('Ctrl Pts',(2.38272078806668,137.827505244843,13.4114267938098));
#80671=CARTESIAN_POINT('Ctrl Pts',(2.38418591104725,137.825580522056,13.3895898716165));
#80672=CARTESIAN_POINT('Ctrl Pts',(2.38510036017024,137.824606797752,13.3757516794376));
#80673=CARTESIAN_POINT('Ctrl Pts',(2.39026989169334,137.820439133956,13.2965630087617));
#80674=CARTESIAN_POINT('Ctrl Pts',(2.39430478192049,137.822450397756,13.2310462106728));
#80675=CARTESIAN_POINT('Ctrl Pts',(2.40151098035598,137.83572054376,13.1151443196098));
#80676=CARTESIAN_POINT('Ctrl Pts',(2.40467113387298,137.844859456328,13.0646954947855));
#80677=CARTESIAN_POINT('Ctrl Pts',(2.40939932616093,137.862959193525,12.9921210168449));
#80678=CARTESIAN_POINT('Ctrl Pts',(2.41090490556354,137.86935186253,12.9694157444935));
#80679=CARTESIAN_POINT('Ctrl Pts',(2.41372229769881,137.882409200919,12.9278645682477));
#80680=CARTESIAN_POINT('Ctrl Pts',(2.41502799622043,137.888880306906,12.908966849498));
#80681=CARTESIAN_POINT('Ctrl Pts',(2.41724298798655,137.900526983021,12.8775825192685));
#80682=CARTESIAN_POINT('Ctrl Pts',(2.41814356103877,137.905442759992,12.8650036027267));
#80683=CARTESIAN_POINT('Ctrl Pts',(2.41997204211476,137.915775907125,12.839847142172));
#80684=CARTESIAN_POINT('Ctrl Pts',(2.42090001345591,137.921198502948,12.8272740345724));
#80685=CARTESIAN_POINT('Ctrl Pts',(2.42327065143957,137.93549166057,12.7956606332028));
#80686=CARTESIAN_POINT('Ctrl Pts',(2.42472313582341,137.94465433273,12.7767585403582));
#80687=CARTESIAN_POINT('Ctrl Pts',(2.43184752135921,137.991510012431,12.6863408938383));
#80688=CARTESIAN_POINT('Ctrl Pts',(2.43775288960991,138.035987712953,12.6186001107558));
#80689=CARTESIAN_POINT('Ctrl Pts',(2.44807394619868,138.124690481633,12.5097594508452));
#80690=CARTESIAN_POINT('Ctrl Pts',(2.45245277928582,138.1657966472,12.466481603452));
#80691=CARTESIAN_POINT('Ctrl Pts',(2.45757202356835,138.21961343685,12.4178097268812));
#80692=CARTESIAN_POINT('Ctrl Pts',(2.45847719720754,138.22936416045,12.4092793344997));
#80693=CARTESIAN_POINT('Ctrl Pts',(2.4599137108304,138.245248935978,12.3958387531089));
#80694=CARTESIAN_POINT('Ctrl Pts',(2.46045184443412,138.251294597947,12.3908262201031));
#80695=CARTESIAN_POINT('Ctrl Pts',(2.46153208348657,138.263633059035,12.3808028049711));
#80696=CARTESIAN_POINT('Ctrl Pts',(2.46207398446655,138.269927887874,12.3757952197848));
#80697=CARTESIAN_POINT('Ctrl Pts',(2.4635304760307,138.287116566024,12.3624067155546));
#80698=CARTESIAN_POINT('Ctrl Pts',(2.46443692383154,138.298106963837,12.3541510883681));
#80699=CARTESIAN_POINT('Ctrl Pts',(2.46974089713571,138.363971711688,12.306456122906));
#80700=CARTESIAN_POINT('Ctrl Pts',(2.47390281228041,138.422019827442,12.2716019509782));
#80701=CARTESIAN_POINT('Ctrl Pts',(2.48255144186157,138.547765708745,12.2101295802508));
#80702=CARTESIAN_POINT('Ctrl Pts',(2.48702651210484,138.615572691124,12.1844070781383));
#80703=CARTESIAN_POINT('Ctrl Pts',(2.49302055325611,138.704911492484,12.1596352822596));
#80704=CARTESIAN_POINT('Ctrl Pts',(2.49434993994169,138.724651767359,12.1547086889104));
#80705=CARTESIAN_POINT('Ctrl Pts',(2.49659746925259,138.757818684663,12.14733822211));
#80706=CARTESIAN_POINT('Ctrl Pts',(2.49750648697719,138.771178423432,12.1446119165284));
#80707=CARTESIAN_POINT('Ctrl Pts',(2.49934647970019,138.798089224461,12.1396052996263));
#80708=CARTESIAN_POINT('Ctrl Pts',(2.5002774253177,138.811638842421,12.1373289938924));
#80709=CARTESIAN_POINT('Ctrl Pts',(2.50264515492876,138.84591527995,12.1321855020265));
#80710=CARTESIAN_POINT('Ctrl Pts',(2.5040915052838,138.866683689059,12.1296327642032));
#80711=CARTESIAN_POINT('Ctrl Pts',(2.51122721403268,138.968265985038,12.1198856326596));
#80712=CARTESIAN_POINT('Ctrl Pts',(2.51715038312931,139.049596363856,12.1205030222231));
#80713=CARTESIAN_POINT('Ctrl Pts',(2.52738559354353,139.188131821146,12.1359129221112));
#80714=CARTESIAN_POINT('Ctrl Pts',(2.53166186741653,139.245507379856,12.1466485243347));
#80715=CARTESIAN_POINT('Ctrl Pts',(2.53670134925441,139.314551830955,12.1649560724034));
#80716=CARTESIAN_POINT('Ctrl Pts',(2.53761915624092,139.327190877144,12.1685346942726));
#80717=CARTESIAN_POINT('Ctrl Pts',(2.53907341540822,139.347360371918,12.1746117511051));
#80718=CARTESIAN_POINT('Ctrl Pts',(2.5396168056144,139.354929709527,12.176976024111));
#80719=CARTESIAN_POINT('Ctrl Pts',(2.54070249699927,139.370131193591,12.1818932455645));
#80720=CARTESIAN_POINT('Ctrl Pts',(2.54124465009739,139.377762188072,12.1844483187086));
#80721=CARTESIAN_POINT('Ctrl Pts',(2.54270111718668,139.398349993115,12.1915771911104));
#80722=CARTESIAN_POINT('Ctrl Pts',(2.54360730825848,139.41125434383,12.1962999749666));
#80723=CARTESIAN_POINT('Ctrl Pts',(2.54892245681042,139.487276639879,12.2256414952513));
#80724=CARTESIAN_POINT('Ctrl Pts',(2.55309476832289,139.548264799519,12.2554461967351));
#80725=CARTESIAN_POINT('Ctrl Pts',(2.56177207600366,139.668640266625,12.3277379455101));
#80726=CARTESIAN_POINT('Ctrl Pts',(2.56626547947886,139.727322110554,12.3708205972148));
#80727=CARTESIAN_POINT('Ctrl Pts',(2.57226350223519,139.79667163363,12.4323524860332));
#80728=CARTESIAN_POINT('Ctrl Pts',(2.57357577401968,139.811341058487,12.4460541528802));
#80729=CARTESIAN_POINT('Ctrl Pts',(2.57580232370098,139.835334820325,12.4696415572273));
#80730=CARTESIAN_POINT('Ctrl Pts',(2.57670784220026,139.844851383168,12.4793261794082));
#80731=CARTESIAN_POINT('Ctrl Pts',(2.5785471687522,139.863683246502,12.4991653532434));
#80732=CARTESIAN_POINT('Ctrl Pts',(2.57948105188919,139.87299198058,12.5093231662068));
#80733=CARTESIAN_POINT('Ctrl Pts',(2.58186968724454,139.896151278757,12.5355025224336));
#80734=CARTESIAN_POINT('Ctrl Pts',(2.58333439004339,139.909751326121,12.5517380596833));
#80735=CARTESIAN_POINT('Ctrl Pts',(2.59032458202646,139.971814861545,12.6300231117368));
#80736=CARTESIAN_POINT('Ctrl Pts',(2.59606788310749,140.014407679925,12.6964550673818));
#80737=CARTESIAN_POINT('Ctrl Pts',(2.60641231920528,140.078182210739,12.8220076299135));
#80738=CARTESIAN_POINT('Ctrl Pts',(2.61097741341454,140.101890564828,12.8795333896135));
#80739=CARTESIAN_POINT('Ctrl Pts',(2.61622089572783,140.124739890963,12.9504178079355));
#80740=CARTESIAN_POINT('Ctrl Pts',(2.61708219075277,140.128343351051,12.9622295983991));
#80741=CARTESIAN_POINT('Ctrl Pts',(2.61846891045585,140.133908733837,12.9815564231586));
#80742=CARTESIAN_POINT('Ctrl Pts',(2.61900025170515,140.135983215132,12.9890378220453));
#80743=CARTESIAN_POINT('Ctrl Pts',(2.62008566264482,140.140103423939,13.0044887030572));
#80744=CARTESIAN_POINT('Ctrl Pts',(2.62063923220957,140.142139900528,13.0124600867968));
#80745=CARTESIAN_POINT('Ctrl Pts',(2.62216691417989,140.147571698341,13.034690582458));
#80746=CARTESIAN_POINT('Ctrl Pts',(2.62313146678731,140.150784746255,13.0489932158116));
#80747=CARTESIAN_POINT('Ctrl Pts',(2.62780971386251,140.165234984486,13.119442734379));
#80748=CARTESIAN_POINT('Ctrl Pts',(2.63136248784062,140.172635508967,13.1763032675171));
#80749=CARTESIAN_POINT('Ctrl Pts',(2.63834502554683,140.179012900032,13.2890392135396));
#80750=CARTESIAN_POINT('Ctrl Pts',(2.64176753553828,140.178214243876,13.344748063664));
#80751=CARTESIAN_POINT('Ctrl Pts',(2.64683311795144,140.171385549814,13.4247301074581));
#80752=CARTESIAN_POINT('Ctrl Pts',(2.64840284579948,140.168521104795,13.4491979201679));
#80753=CARTESIAN_POINT('Ctrl Pts',(2.65132723971652,140.161850757156,13.4939684569883));
#80754=CARTESIAN_POINT('Ctrl Pts',(2.65267497205706,140.158273842006,13.5142955145468));
#80755=CARTESIAN_POINT('Ctrl Pts',(2.65494318086267,140.151443266099,13.5479118654387));
#80756=CARTESIAN_POINT('Ctrl Pts',(2.65585408809344,140.148488699442,13.5612576673292));
#80757=CARTESIAN_POINT('Ctrl Pts',(2.65768956496284,140.142121125143,13.5878205437596));
#80758=CARTESIAN_POINT('Ctrl Pts',(2.65861397038254,140.138709272596,13.6010357040442));
#80759=CARTESIAN_POINT('Ctrl Pts',(2.66094726208514,140.129593504645,13.6339682748677));
#80760=CARTESIAN_POINT('Ctrl Pts',(2.66236519682339,140.123602553707,13.6536007685401));
#80761=CARTESIAN_POINT('Ctrl Pts',(2.669743135192,140.090154788374,13.7537562324198));
#80762=CARTESIAN_POINT('Ctrl Pts',(2.6759660382059,140.054548305496,13.8312771278612));
#80763=CARTESIAN_POINT('Ctrl Pts',(2.68508805045857,139.990827878354,13.9378776161496));
#80764=CARTESIAN_POINT('Ctrl Pts',(2.68795849905837,139.969077288269,13.9704604696807));
#80765=CARTESIAN_POINT('Ctrl Pts',(2.69196624158601,139.935899495469,14.0151643297314));
#80766=CARTESIAN_POINT('Ctrl Pts',(2.69314556178104,139.925777267946,14.0282200144966));
#80767=CARTESIAN_POINT('Ctrl Pts',(2.69523417996089,139.907150796955,14.0512281124043));
#80768=CARTESIAN_POINT('Ctrl Pts',(2.69614849047403,139.898749012578,14.061259806929));
#80769=CARTESIAN_POINT('Ctrl Pts',(2.6975976009109,139.885005722024,14.0771244539462));
#80770=CARTESIAN_POINT('Ctrl Pts',(2.69813930780114,139.87976983265,14.0830469956334));
#80771=CARTESIAN_POINT('Ctrl Pts',(2.69922270416607,139.869090664656,14.0948843173224));
#80772=CARTESIAN_POINT('Ctrl Pts',(2.69976423547238,139.863645701496,14.1007969612631));
#80773=CARTESIAN_POINT('Ctrl Pts',(2.70121841231904,139.848747508035,14.116646071639));
#80774=CARTESIAN_POINT('Ctrl Pts',(2.70212296075423,139.839180261047,14.1264742393575));
#80775=CARTESIAN_POINT('Ctrl Pts',(2.70747480747601,139.780931870744,14.1842565399776));
#80776=CARTESIAN_POINT('Ctrl Pts',(2.7116807756843,139.728318596275,14.2280724683605));
#80777=CARTESIAN_POINT('Ctrl Pts',(2.71896711854889,139.631494000551,14.2953730326502));
#80778=CARTESIAN_POINT('Ctrl Pts',(2.72203098029131,139.589047695657,14.321065410084));
#80779=CARTESIAN_POINT('Ctrl Pts',(2.72663659360722,139.524533514388,14.3547504607225));
#80780=CARTESIAN_POINT('Ctrl Pts',(2.72812006565005,139.503643737149,14.3648834815391));
#80781=CARTESIAN_POINT('Ctrl Pts',(2.7309023439459,139.464438134442,14.3824892423539));
#80782=CARTESIAN_POINT('Ctrl Pts',(2.73219538132343,139.446207106281,14.3901306732219));
#80783=CARTESIAN_POINT('Ctrl Pts',(2.734398854613,139.415195769642,14.4022206459882));
#80784=CARTESIAN_POINT('Ctrl Pts',(2.73530094314328,139.402515097274,14.4069143825244));
#80785=CARTESIAN_POINT('Ctrl Pts',(2.73703174222824,139.37823355822,14.4154297626416));
#80786=CARTESIAN_POINT('Ctrl Pts',(2.73785899297669,139.366648494687,14.4192913122783));
#80787=CARTESIAN_POINT('Ctrl Pts',(2.74005812356436,139.335919381437,14.4290057271924));
#80788=CARTESIAN_POINT('Ctrl Pts',(2.74143974328702,139.316683275063,14.4345516209504));
#80789=CARTESIAN_POINT('Ctrl Pts',(2.74904499861801,139.211237336399,14.4620618552608));
#80790=CARTESIAN_POINT('Ctrl Pts',(2.75556162124577,139.122904598153,14.4746906426126));
#80791=CARTESIAN_POINT('Ctrl Pts',(2.76482496490398,138.996786747674,14.4783342369882));
#80792=CARTESIAN_POINT('Ctrl Pts',(2.76755157684444,138.959530033395,14.4776435622599));
#80793=CARTESIAN_POINT('Ctrl Pts',(2.77138473949638,138.906344529368,14.4741301275034));
#80794=CARTESIAN_POINT('Ctrl Pts',(2.77253005615581,138.890344523968,14.4727440605465));
#80795=CARTESIAN_POINT('Ctrl Pts',(2.77456557616334,138.861635890586,14.4696643289929));
#80796=CARTESIAN_POINT('Ctrl Pts',(2.77546043949872,138.848917158788,14.468089584899));
#80797=CARTESIAN_POINT('Ctrl Pts',(2.77688682533256,138.828447362137,14.4652151971332));
#80798=CARTESIAN_POINT('Ctrl Pts',(2.7774248808188,138.820679458299,14.4640450670873));
#80799=CARTESIAN_POINT('Ctrl Pts',(2.77850912859651,138.804920066812,14.4615096188324));
#80800=CARTESIAN_POINT('Ctrl Pts',(2.77905504088709,138.796929871471,14.4601393483755));
#80801=CARTESIAN_POINT('Ctrl Pts',(2.78053546697373,138.775132086452,14.4561690499583));
#80802=CARTESIAN_POINT('Ctrl Pts',(2.78146137786792,138.761355407105,14.453404201376));
#80803=CARTESIAN_POINT('Ctrl Pts',(2.78657798172832,138.684661493557,14.4365793613153));
#80804=CARTESIAN_POINT('Ctrl Pts',(2.7905574157926,138.62292506064,14.4176168633181));
#80805=CARTESIAN_POINT('Ctrl Pts',(2.79773282293255,138.515097844997,14.3745375203155));
#80806=CARTESIAN_POINT('Ctrl Pts',(2.8009187210109,138.468463586943,14.3522497975832));
#80807=CARTESIAN_POINT('Ctrl Pts',(2.80568176338657,138.402766683406,14.3153668060605));
#80808=CARTESIAN_POINT('Ctrl Pts',(2.80719570560732,138.382445466318,14.3031369193902));
#80809=CARTESIAN_POINT('Ctrl Pts',(2.81002831548545,138.345627946676,14.2794362133505));
#80810=CARTESIAN_POINT('Ctrl Pts',(2.81134081580199,138.329029241261,14.268140611536));
#80811=CARTESIAN_POINT('Ctrl Pts',(2.81356733303682,138.301705141275,14.2485059820357));
#80812=CARTESIAN_POINT('Ctrl Pts',(2.81447257598025,138.290820386679,14.2403954262185));
#80813=CARTESIAN_POINT('Ctrl Pts',(2.81631096095968,138.269182197627,14.2236828261546));
#80814=CARTESIAN_POINT('Ctrl Pts',(2.81724417199555,138.258434625036,14.2150767127517));
#80815=CARTESIAN_POINT('Ctrl Pts',(2.81963021074647,138.23156623608,14.1927776365519));
#80816=CARTESIAN_POINT('Ctrl Pts',(2.82109295833759,138.215659456017,14.178835689056));
#80817=CARTESIAN_POINT('Ctrl Pts',(2.82809624855325,138.142188946103,14.1108564104354));
#80818=CARTESIAN_POINT('Ctrl Pts',(2.83385615181188,138.089787170954,14.0515562314469));
#80819=CARTESIAN_POINT('Ctrl Pts',(2.84410799879032,138.008321553379,13.9382366290328));
#80820=CARTESIAN_POINT('Ctrl Pts',(2.8485637062218,137.976777856709,13.8863359681887));
#80821=CARTESIAN_POINT('Ctrl Pts',(2.85375788054518,137.943499476499,13.8206442738174));
#80822=CARTESIAN_POINT('Ctrl Pts',(2.85466545471157,137.937820798617,13.8089589329466));
#80823=CARTESIAN_POINT('Ctrl Pts',(2.85610679578974,137.929006096192,13.7900299528661));
#80824=CARTESIAN_POINT('Ctrl Pts',(2.85664733617375,137.925747639733,13.7828448759772));
#80825=CARTESIAN_POINT('Ctrl Pts',(2.85773109774786,137.919306156813,13.7682529841614));
#80826=CARTESIAN_POINT('Ctrl Pts',(2.85827411959659,137.91612650171,13.7608451900794));
#80827=CARTESIAN_POINT('Ctrl Pts',(2.85973740429669,137.907698472623,13.7406401366959));
#80828=CARTESIAN_POINT('Ctrl Pts',(2.86064939361364,137.902598889426,13.7277817204549));
#80829=CARTESIAN_POINT('Ctrl Pts',(2.86229480890035,137.893710802472,13.7041649034555));
#80830=CARTESIAN_POINT('Ctrl Pts',(2.86303115989592,137.889850956811,13.6934387371489));
#80831=CARTESIAN_POINT('Ctrl Pts',(2.86376176824068,137.886148206833,13.6826607444707));
#80832=CARTESIAN_POINT('Origin',(1.13913288526384,139.,13.3));
#80833=CARTESIAN_POINT('',(3.46173780540502,137.886148220981,13.6826607856522));
#80834=CARTESIAN_POINT('',(3.36195598355709,137.886148212417,13.6826607607244));
#80835=CARTESIAN_POINT('',(1.13913288526384,137.88614821265,13.6826607614027));
#80836=CARTESIAN_POINT('Ctrl Pts',(3.46173780698925,137.886148221013,13.6826607857451));
#80837=CARTESIAN_POINT('Ctrl Pts',(3.45836838296447,137.903798630072,13.7340377239194));
#80838=CARTESIAN_POINT('Ctrl Pts',(3.4549629707539,137.924986636544,13.7841441124887));
#80839=CARTESIAN_POINT('Ctrl Pts',(3.45016111005712,137.958539568967,13.8503170867777));
#80840=CARTESIAN_POINT('Ctrl Pts',(3.44886346368914,137.967957637348,13.867782715661));
#80841=CARTESIAN_POINT('Ctrl Pts',(3.44665880860375,137.984502739928,13.8966924042346));
#80842=CARTESIAN_POINT('Ctrl Pts',(3.44576031457575,137.991393398323,13.9082673820296));
#80843=CARTESIAN_POINT('Ctrl Pts',(3.44393330418159,138.005689426144,13.9313709083526));
#80844=CARTESIAN_POINT('Ctrl Pts',(3.44300467975767,138.013100458757,13.9428934663466));
#80845=CARTESIAN_POINT('Ctrl Pts',(3.44062623712217,138.03243567786,13.9718331692168));
#80846=CARTESIAN_POINT('Ctrl Pts',(3.43916649497018,138.044629745427,13.9890632057143));
#80847=CARTESIAN_POINT('Ctrl Pts',(3.43375299313194,138.091009244744,14.0509975789069));
#80848=CARTESIAN_POINT('Ctrl Pts',(3.42969913269336,138.127919275501,14.0935586035251));
#80849=CARTESIAN_POINT('Ctrl Pts',(3.41950168214345,138.226636605513,14.1921528536077));
#80850=CARTESIAN_POINT('Ctrl Pts',(3.41330701396937,138.291623602701,14.2445802319252));
#80851=CARTESIAN_POINT('Ctrl Pts',(3.40651566562879,138.372527379974,14.2967659164351));
#80852=CARTESIAN_POINT('Ctrl Pts',(3.40560701895227,138.383572286705,14.3036339425661));
#80853=CARTESIAN_POINT('Ctrl Pts',(3.40416654812882,138.401471968,14.3143574513776));
#80854=CARTESIAN_POINT('Ctrl Pts',(3.40362790460698,138.408255242592,14.3183295128722));
#80855=CARTESIAN_POINT('Ctrl Pts',(3.40255137636818,138.422004684899,14.3261969425864));
#80856=CARTESIAN_POINT('Ctrl Pts',(3.4020136377026,138.428971667734,14.3300899972183));
#80857=CARTESIAN_POINT('Ctrl Pts',(3.40057142001163,138.447907618626,14.3404199801074));
#80858=CARTESIAN_POINT('Ctrl Pts',(3.39967488138512,138.459949676213,14.3467212711553));
#80859=CARTESIAN_POINT('Ctrl Pts',(3.39423534859957,138.53447122782,14.3840878500927));
#80860=CARTESIAN_POINT('Ctrl Pts',(3.38994529973612,138.599507540974,14.4097619971875));
#80861=CARTESIAN_POINT('Ctrl Pts',(3.38121794782789,138.734956449527,14.4497611357717));
#80862=CARTESIAN_POINT('Ctrl Pts',(3.37679391651474,138.805162748747,14.463716334325));
#80863=CARTESIAN_POINT('Ctrl Pts',(3.37088986772326,138.895867876636,14.4733042413624));
#80864=CARTESIAN_POINT('Ctrl Pts',(3.36959600343743,138.915587325411,14.4748875554781));
#80865=CARTESIAN_POINT('Ctrl Pts',(3.3673958482543,138.948775783991,14.4767124990439));
#80866=CARTESIAN_POINT('Ctrl Pts',(3.36649799012021,138.962226354736,14.4772210293705));
#80867=CARTESIAN_POINT('Ctrl Pts',(3.36467067810907,138.989392028937,14.4777820563403));
#80868=CARTESIAN_POINT('Ctrl Pts',(3.36374109055478,139.003105197759,14.4778257219704));
#80869=CARTESIAN_POINT('Ctrl Pts',(3.36135670714543,139.037990177743,14.4773275953248));
#80870=CARTESIAN_POINT('Ctrl Pts',(3.35989188592125,139.059151554218,14.4764542120358));
#80871=CARTESIAN_POINT('Ctrl Pts',(3.3529626225683,139.1579462292,14.4697045597161));
#80872=CARTESIAN_POINT('Ctrl Pts',(3.34728588692791,139.234886570133,14.4567110490137));
#80873=CARTESIAN_POINT('Ctrl Pts',(3.33840595325053,139.351515204987,14.4248940301977));
#80874=CARTESIAN_POINT('Ctrl Pts',(3.33524118673407,139.392409245801,14.4112897078416));
#80875=CARTESIAN_POINT('Ctrl Pts',(3.33088142890843,139.448642233739,14.3890902605491));
#80876=CARTESIAN_POINT('Ctrl Pts',(3.32963773032751,139.464674203836,14.3823471699356));
#80877=CARTESIAN_POINT('Ctrl Pts',(3.32744987806223,139.492946540754,14.3697116842225));
#80878=CARTESIAN_POINT('Ctrl Pts',(3.32650001641606,139.50524530785,14.3639579869557));
#80879=CARTESIAN_POINT('Ctrl Pts',(3.32501058194549,139.524608995583,14.3544876046362));
#80880=CARTESIAN_POINT('Ctrl Pts',(3.32446340574519,139.531739989095,14.3509097487427));
#80881=CARTESIAN_POINT('Ctrl Pts',(3.32338603398,139.545825820355,14.3436623291972));
#80882=CARTESIAN_POINT('Ctrl Pts',(3.32285575840621,139.55278132278,14.339995048269));
#80883=CARTESIAN_POINT('Ctrl Pts',(3.32145837865224,139.571152442221,14.3300725105765));
#80884=CARTESIAN_POINT('Ctrl Pts',(3.32059838025901,139.582502349165,14.3236969948901));
#80885=CARTESIAN_POINT('Ctrl Pts',(3.31482710664153,139.658755003209,14.2791850590484));
#80886=CARTESIAN_POINT('Ctrl Pts',(3.31021736387331,139.719985865332,14.2350854680397));
#80887=CARTESIAN_POINT('Ctrl Pts',(3.30163879361943,139.824311371667,14.1435842883494));
#80888=CARTESIAN_POINT('Ctrl Pts',(3.29769709531925,139.868563508873,14.0979473592663));
#80889=CARTESIAN_POINT('Ctrl Pts',(3.29221966239704,139.922578631638,14.0323967098507));
#80890=CARTESIAN_POINT('Ctrl Pts',(3.29081932656742,139.935779178061,14.0154533589605));
#80891=CARTESIAN_POINT('Ctrl Pts',(3.28849154127559,139.956670325095,13.9870709718419));
#80892=CARTESIAN_POINT('Ctrl Pts',(3.28757492063597,139.964636728147,13.9758406520039));
#80893=CARTESIAN_POINT('Ctrl Pts',(3.28576043245001,139.979886476013,13.953523863034));
#80894=CARTESIAN_POINT('Ctrl Pts',(3.28486324619194,139.987183036697,13.9424488870522));
#80895=CARTESIAN_POINT('Ctrl Pts',(3.28263558342335,140.004693778336,13.9148676214361));
#80896=CARTESIAN_POINT('Ctrl Pts',(3.28129737408778,140.014689558669,13.8982280514226));
#80897=CARTESIAN_POINT('Ctrl Pts',(3.27346485324006,140.070162278796,13.8004917436436));
#80898=CARTESIAN_POINT('Ctrl Pts',(3.26664388542069,140.10631187933,13.7144963522789));
#80899=CARTESIAN_POINT('Ctrl Pts',(3.25721729603795,140.14177476633,13.5910429590802));
#80900=CARTESIAN_POINT('Ctrl Pts',(3.25462110955812,140.150029680615,13.5564909711158));
#80901=CARTESIAN_POINT('Ctrl Pts',(3.2509494330637,140.159646245647,13.5062981698378));
#80902=CARTESIAN_POINT('Ctrl Pts',(3.24983796188384,140.162276798773,13.49092155693));
#80903=CARTESIAN_POINT('Ctrl Pts',(3.24785670157042,140.166467640818,13.4631109749276));
#80904=CARTESIAN_POINT('Ctrl Pts',(3.24698256610957,140.16813644254,13.4506958219219));
#80905=CARTESIAN_POINT('Ctrl Pts',(3.24558296370976,140.170518381318,13.4305452587776));
#80906=CARTESIAN_POINT('Ctrl Pts',(3.24505131614193,140.171353596489,13.4228255251882));
#80907=CARTESIAN_POINT('Ctrl Pts',(3.24397408217778,140.172903856802,13.4070382469128));
#80908=CARTESIAN_POINT('Ctrl Pts',(3.24342885740922,140.173612152311,13.3989705475416));
#80909=CARTESIAN_POINT('Ctrl Pts',(3.24194163928365,140.175330390584,13.3767735112108));
#80910=CARTESIAN_POINT('Ctrl Pts',(3.24100845544324,140.176168781239,13.3626317880328));
#80911=CARTESIAN_POINT('Ctrl Pts',(3.23593604413233,140.179373999623,13.2848279198774));
#80912=CARTESIAN_POINT('Ctrl Pts',(3.23200192620154,140.176827942798,13.221062715401));
#80913=CARTESIAN_POINT('Ctrl Pts',(3.22485021694789,140.16285605262,13.1061807304899));
#80914=CARTESIAN_POINT('Ctrl Pts',(3.22164194641489,140.153164000722,13.0550254956201));
#80915=CARTESIAN_POINT('Ctrl Pts',(3.21685223766466,140.1341637527,12.9816722612954));
#80916=CARTESIAN_POINT('Ctrl Pts',(3.21533502313076,140.127509213828,12.9588507142722));
#80917=CARTESIAN_POINT('Ctrl Pts',(3.2124986664702,140.113966252323,12.9171454586621));
#80918=CARTESIAN_POINT('Ctrl Pts',(3.21118576990382,140.10727611206,12.8982065887315));
#80919=CARTESIAN_POINT('Ctrl Pts',(3.20896293948137,140.095280046206,12.8668264881014));
#80920=CARTESIAN_POINT('Ctrl Pts',(3.20806185296122,140.090238021495,12.8542885442418));
#80921=CARTESIAN_POINT('Ctrl Pts',(3.20623587025286,140.079671968242,12.8292667465182));
#80922=CARTESIAN_POINT('Ctrl Pts',(3.20531096720339,140.074144406381,12.8167866704284));
#80923=CARTESIAN_POINT('Ctrl Pts',(3.20295553797155,140.059635614489,12.7855086262486));
#80924=CARTESIAN_POINT('Ctrl Pts',(3.20151547786178,140.050370522561,12.7668483533693));
#80925=CARTESIAN_POINT('Ctrl Pts',(3.19433579516952,140.002284031912,12.6761238902412));
#80926=CARTESIAN_POINT('Ctrl Pts',(3.18835678133591,139.956523142738,12.6080072330928));
#80927=CARTESIAN_POINT('Ctrl Pts',(3.17808917411832,139.866939104729,12.5007062524346));
#80928=CARTESIAN_POINT('Ctrl Pts',(3.17383654351491,139.826559592481,12.4590158547615));
#80929=CARTESIAN_POINT('Ctrl Pts',(3.16881717108323,139.773444214679,12.4117138599098));
#80930=CARTESIAN_POINT('Ctrl Pts',(3.16789740098424,139.763470720846,12.4031272583048));
#80931=CARTESIAN_POINT('Ctrl Pts',(3.16644372228409,139.747288857042,12.3896612139027));
#80932=CARTESIAN_POINT('Ctrl Pts',(3.16590278581643,139.741171992806,12.384674140957));
#80933=CARTESIAN_POINT('Ctrl Pts',(3.16482619341234,139.728796278721,12.3747896508646));
#80934=CARTESIAN_POINT('Ctrl Pts',(3.1642906185319,139.722537077851,12.3698933467504));
#80935=CARTESIAN_POINT('Ctrl Pts',(3.16286136406658,139.705572319966,12.3568971630647));
#80936=CARTESIAN_POINT('Ctrl Pts',(3.1619753812029,139.694776717644,12.3489160866601));
#80937=CARTESIAN_POINT('Ctrl Pts',(3.156425623832,139.625563384154,12.2995550209397));
#80938=CARTESIAN_POINT('Ctrl Pts',(3.15203005996752,139.563604428024,12.2633841995888));
#80939=CARTESIAN_POINT('Ctrl Pts',(3.14333910096303,139.436206454115,12.2038323834162));
#80940=CARTESIAN_POINT('Ctrl Pts',(3.13906025550019,139.371234114205,12.1801592256757));
#80941=CARTESIAN_POINT('Ctrl Pts',(3.13329083730982,139.285051533183,12.1570875697915));
#80942=CARTESIAN_POINT('Ctrl Pts',(3.13197047012983,139.265406149983,12.1523664798762));
#80943=CARTESIAN_POINT('Ctrl Pts',(3.1297387185587,139.232413100441,12.1453301782094));
#80944=CARTESIAN_POINT('Ctrl Pts',(3.12883634579817,139.219129036005,12.142735688635));
#80945=CARTESIAN_POINT('Ctrl Pts',(3.127010759545,139.192387944015,12.1379898486125));
#80946=CARTESIAN_POINT('Ctrl Pts',(3.12608758758131,139.178932431487,12.1358419906512));
#80947=CARTESIAN_POINT('Ctrl Pts',(3.12374290479611,139.144945382887,12.1310198824146));
#80948=CARTESIAN_POINT('Ctrl Pts',(3.12231204065755,139.124375696271,12.1286527965437));
#80949=CARTESIAN_POINT('Ctrl Pts',(3.11505855702339,139.021014221465,12.1195114928741));
#80950=CARTESIAN_POINT('Ctrl Pts',(3.1089878774016,138.937743712085,12.1209688224316));
#80951=CARTESIAN_POINT('Ctrl Pts',(3.09869023911081,138.798610077406,12.138189292158));
#80952=CARTESIAN_POINT('Ctrl Pts',(3.09449856238143,138.742466710349,12.1493307189832));
#80953=CARTESIAN_POINT('Ctrl Pts',(3.08954210526601,138.67473893858,12.1679790599948));
#80954=CARTESIAN_POINT('Ctrl Pts',(3.08862797395389,138.662185632882,12.1716615507934));
#80955=CARTESIAN_POINT('Ctrl Pts',(3.08718099203487,138.642176414888,12.1778951160327));
#80956=CARTESIAN_POINT('Ctrl Pts',(3.08664121942925,138.634680558193,12.180313077565));
#80957=CARTESIAN_POINT('Ctrl Pts',(3.08556467203787,138.61965526003,12.185326793539));
#80958=CARTESIAN_POINT('Ctrl Pts',(3.08502801103589,138.612126783704,12.1879240782118));
#80959=CARTESIAN_POINT('Ctrl Pts',(3.08359225929201,138.591902064861,12.1951318769706));
#80960=CARTESIAN_POINT('Ctrl Pts',(3.08270098694365,138.579257439121,12.1998849015177));
#80961=CARTESIAN_POINT('Ctrl Pts',(3.07720264407398,138.500920871212,12.2308794096361));
#80962=CARTESIAN_POINT('Ctrl Pts',(3.07285651860873,138.43761494184,12.2627804745131));
#80963=CARTESIAN_POINT('Ctrl Pts',(3.06411762173651,138.317566322302,12.3375179041533));
#80964=CARTESIAN_POINT('Ctrl Pts',(3.05973944968749,138.261071989804,12.3801785864653));
#80965=CARTESIAN_POINT('Ctrl Pts',(3.05388674823547,138.194102149079,12.4409223129584));
#80966=CARTESIAN_POINT('Ctrl Pts',(3.05259371580389,138.179797767602,12.4545687240624));
#80967=CARTESIAN_POINT('Ctrl Pts',(3.05039454783694,138.156343957378,12.4780993698694));
#80968=CARTESIAN_POINT('Ctrl Pts',(3.04949682700704,138.147008125544,12.4877925137365));
#80969=CARTESIAN_POINT('Ctrl Pts',(3.04766943956062,138.12849675394,12.5076836015772));
#80970=CARTESIAN_POINT('Ctrl Pts',(3.04673963356958,138.11932922425,12.5178861079576));
#80971=CARTESIAN_POINT('Ctrl Pts',(3.04435391411528,138.096455146639,12.5442547438014));
#80972=CARTESIAN_POINT('Ctrl Pts',(3.04288795252716,138.083003477047,12.5606344138111));
#80973=CARTESIAN_POINT('Ctrl Pts',(3.03738147642545,138.03472191734,12.622770764814));
#80974=CARTESIAN_POINT('Ctrl Pts',(3.03323581444742,138.002819103006,12.6706909550478));
#80975=CARTESIAN_POINT('Ctrl Pts',(3.02303387021577,137.93420670332,12.7921548859122));
#80976=CARTESIAN_POINT('Ctrl Pts',(3.01693586612402,137.901435833194,12.8675880044185));
#80977=CARTESIAN_POINT('Ctrl Pts',(3.01023981030961,137.872882901291,12.9581388769779));
#80978=CARTESIAN_POINT('Ctrl Pts',(3.00933727578236,137.869200383165,12.9705242908488));
#80979=CARTESIAN_POINT('Ctrl Pts',(3.00790405585608,137.863611049326,12.9905218478332));
#80980=CARTESIAN_POINT('Ctrl Pts',(3.00736666509325,137.861575270655,12.9980965050352));
#80981=CARTESIAN_POINT('Ctrl Pts',(3.0062901193871,137.857616142088,13.0134372999262));
#80982=CARTESIAN_POINT('Ctrl Pts',(3.00575114704534,137.855695957887,13.021203786753));
#80983=CARTESIAN_POINT('Ctrl Pts',(3.00430151962512,137.850706174465,13.0423063484932));
#80984=CARTESIAN_POINT('Ctrl Pts',(3.00339894570211,137.847789517265,13.0556777562563));
#80985=CARTESIAN_POINT('Ctrl Pts',(2.9980588046626,137.831739586346,13.1359539549935));
#80986=CARTESIAN_POINT('Ctrl Pts',(2.99386158844297,137.824201746464,13.2038531112635));
#80987=CARTESIAN_POINT('Ctrl Pts',(2.98507619683986,137.820825215976,13.3459900454161));
#80988=CARTESIAN_POINT('Ctrl Pts',(2.98049928156362,137.826040736481,13.4199428737051));
#80989=CARTESIAN_POINT('Ctrl Pts',(2.9744562608184,137.841314131111,13.5119283728539));
#80990=CARTESIAN_POINT('Ctrl Pts',(2.97319422149151,137.84493744974,13.5308614603078));
#80991=CARTESIAN_POINT('Ctrl Pts',(2.97103179804789,137.851858618572,13.5627646291086));
#80992=CARTESIAN_POINT('Ctrl Pts',(2.97013916613176,137.854915965702,13.5757832689906));
#80993=CARTESIAN_POINT('Ctrl Pts',(2.96841900833703,137.861183027981,13.6005654422242));
#80994=CARTESIAN_POINT('Ctrl Pts',(2.96759280119882,137.864355071985,13.6123367714931));
#80995=CARTESIAN_POINT('Ctrl Pts',(2.96537867397912,137.873279503437,13.6435197784572));
#80996=CARTESIAN_POINT('Ctrl Pts',(2.96398063800157,137.879350437252,13.6628352031284));
#80997=CARTESIAN_POINT('Ctrl Pts',(2.96255039632898,137.88599320387,13.6822093374455));
#80998=CARTESIAN_POINT('Ctrl Pts',(2.96253372896323,137.886070674307,13.6824350622175));
#80999=CARTESIAN_POINT('Ctrl Pts',(2.96251705962155,137.886148212665,13.6826607614475));
#81000=CARTESIAN_POINT('Ctrl Pts',(2.86376176824068,137.886148206833,13.6826607444707));
#81001=CARTESIAN_POINT('Ctrl Pts',(2.86725567767849,137.868440945227,13.6311183132772));
#81002=CARTESIAN_POINT('Ctrl Pts',(2.87062046861302,137.854326414844,13.5783907776995));
#81003=CARTESIAN_POINT('Ctrl Pts',(2.87713906771859,137.834185868406,13.4748394318849));
#81004=CARTESIAN_POINT('Ctrl Pts',(2.88028484405678,137.82771416093,13.4242454806967));
#81005=CARTESIAN_POINT('Ctrl Pts',(2.88499619080121,137.823071471942,13.3498891616564));
#81006=CARTESIAN_POINT('Ctrl Pts',(2.88650018847356,137.822309281961,13.3263468935304));
#81007=CARTESIAN_POINT('Ctrl Pts',(2.88931634634091,137.822205861884,13.2828247150978));
#81008=CARTESIAN_POINT('Ctrl Pts',(2.89062246892688,137.822666525777,13.2628538517397));
#81009=CARTESIAN_POINT('Ctrl Pts',(2.892841326005,137.824291837794,13.2293663373899));
#81010=CARTESIAN_POINT('Ctrl Pts',(2.89374542417892,137.825182605914,13.2158402617338));
#81011=CARTESIAN_POINT('Ctrl Pts',(2.89558407723261,137.82744997144,13.1885926453274));
#81012=CARTESIAN_POINT('Ctrl Pts',(2.89651874310581,137.828834509547,13.1748739277128));
#81013=CARTESIAN_POINT('Ctrl Pts',(2.8989141149303,137.832965523065,13.1400698801915));
#81014=CARTESIAN_POINT('Ctrl Pts',(2.90038490369175,137.836042643655,13.1190296045035));
#81015=CARTESIAN_POINT('Ctrl Pts',(2.90728800563884,137.852953535013,13.0218503576638));
#81016=CARTESIAN_POINT('Ctrl Pts',(2.91292945815507,137.87369859987,12.9471198244522));
#81017=CARTESIAN_POINT('Ctrl Pts',(2.9230931726133,137.923632998348,12.8180751906311));
#81018=CARTESIAN_POINT('Ctrl Pts',(2.92757963674675,137.950040652123,12.7629673611171));
#81019=CARTESIAN_POINT('Ctrl Pts',(2.93284330922091,137.987363313571,12.6984650745539));
#81020=CARTESIAN_POINT('Ctrl Pts',(2.93378764430336,137.994325513776,12.6868962631589));
#81021=CARTESIAN_POINT('Ctrl Pts',(2.93527260690719,138.005724024588,12.6686726417028));
#81022=CARTESIAN_POINT('Ctrl Pts',(2.93582070534413,138.010031613605,12.6619392254268));
#81023=CARTESIAN_POINT('Ctrl Pts',(2.93683893748925,138.018229610334,12.6494074182241));
#81024=CARTESIAN_POINT('Ctrl Pts',(2.93731013035026,138.022103634643,12.6435988192708));
#81025=CARTESIAN_POINT('Ctrl Pts',(2.93859937393458,138.032918134826,12.6276921408359));
#81026=CARTESIAN_POINT('Ctrl Pts',(2.9394106703059,138.039965112964,12.6176670631507));
#81027=CARTESIAN_POINT('Ctrl Pts',(2.94423117158354,138.083200826815,12.5581559250762));
#81028=CARTESIAN_POINT('Ctrl Pts',(2.94803691158806,138.123056303952,12.5114411958815));
#81029=CARTESIAN_POINT('Ctrl Pts',(2.95528846212442,138.205882640744,12.4284490964462));
#81030=CARTESIAN_POINT('Ctrl Pts',(2.95872792589386,138.248161375517,12.3917259884215));
#81031=CARTESIAN_POINT('Ctrl Pts',(2.96381525364608,138.312636962533,12.3433197910511));
#81032=CARTESIAN_POINT('Ctrl Pts',(2.96538906575527,138.332847143474,12.3291179687968));
#81033=CARTESIAN_POINT('Ctrl Pts',(2.96832033726247,138.370773429674,12.3042105425882));
#81034=CARTESIAN_POINT('Ctrl Pts',(2.96967081299137,138.388354052668,12.2933163995666));
#81035=CARTESIAN_POINT('Ctrl Pts',(2.97194270105114,138.418027383992,12.2759930980345));
#81036=CARTESIAN_POINT('Ctrl Pts',(2.97285449386152,138.429962113949,12.2693016722268));
#81037=CARTESIAN_POINT('Ctrl Pts',(2.97469106963597,138.454032240892,12.2563522498827));
#81038=CARTESIAN_POINT('Ctrl Pts',(2.97561567689895,138.466165267372,12.2500943512662));
#81039=CARTESIAN_POINT('Ctrl Pts',(2.97794818804247,138.496792909123,12.2349655636982));
#81040=CARTESIAN_POINT('Ctrl Pts',(2.97936510920751,138.515414985312,12.2263645877426));
#81041=CARTESIAN_POINT('Ctrl Pts',(2.98674826259363,138.612474285438,12.1845754024765));
#81042=CARTESIAN_POINT('Ctrl Pts',(2.99297793832906,138.694107739314,12.1594854405036));
#81043=CARTESIAN_POINT('Ctrl Pts',(3.00210023764756,138.81608290532,12.1360429606042));
#81044=CARTESIAN_POINT('Ctrl Pts',(3.00496449352447,138.854795268941,12.1305824669314));
#81045=CARTESIAN_POINT('Ctrl Pts',(3.00896490474615,138.910141794031,12.125567022961));
#81046=CARTESIAN_POINT('Ctrl Pts',(3.01014290383602,138.926604861565,12.124423323036));
#81047=CARTESIAN_POINT('Ctrl Pts',(3.01222956436317,138.956146998181,12.1229940819346));
#81048=CARTESIAN_POINT('Ctrl Pts',(3.01314321927118,138.969216991939,12.1225797440055));
#81049=CARTESIAN_POINT('Ctrl Pts',(3.01459178329804,138.990197096921,12.1222642601981));
#81050=CARTESIAN_POINT('Ctrl Pts',(3.0151335793853,138.998103691501,12.1222249856122));
#81051=CARTESIAN_POINT('Ctrl Pts',(3.01621736838379,139.014052370774,12.1223063776968));
#81052=CARTESIAN_POINT('Ctrl Pts',(3.01675919825521,139.022093986797,12.1224297887329));
#81053=CARTESIAN_POINT('Ctrl Pts',(3.01821521393192,139.043867219511,12.1229870628074));
#81054=CARTESIAN_POINT('Ctrl Pts',(3.01912126697991,139.057593972395,12.1235788330994));
#81055=CARTESIAN_POINT('Ctrl Pts',(3.02443280326578,139.138879148907,12.1285093636998));
#81056=CARTESIAN_POINT('Ctrl Pts',(3.02860177066926,139.205979646122,12.1384267861221));
#81057=CARTESIAN_POINT('Ctrl Pts',(3.03587154333044,139.320451898672,12.1655841039019));
#81058=CARTESIAN_POINT('Ctrl Pts',(3.03895721604081,139.368256843347,12.180189590136));
#81059=CARTESIAN_POINT('Ctrl Pts',(3.04359096529599,139.436797037097,12.2059952215988));
#81060=CARTESIAN_POINT('Ctrl Pts',(3.04507989190951,139.45835620476,12.2148513481974));
#81061=CARTESIAN_POINT('Ctrl Pts',(3.04787113758353,139.497739910478,12.232412582544));
#81062=CARTESIAN_POINT('Ctrl Pts',(3.04916761574667,139.515634685109,12.2409397046497));
#81063=CARTESIAN_POINT('Ctrl Pts',(3.05137504973147,139.54536716872,12.2560398771981));
#81064=CARTESIAN_POINT('Ctrl Pts',(3.05227758045623,139.557322461036,12.2623730269015));
#81065=CARTESIAN_POINT('Ctrl Pts',(3.05411717887723,139.581267379282,12.2755907191006));
#81066=CARTESIAN_POINT('Ctrl Pts',(3.05505442439103,139.593250139573,12.2824832264138));
#81067=CARTESIAN_POINT('Ctrl Pts',(3.05746550176222,139.623509289031,12.3006045539693));
#81068=CARTESIAN_POINT('Ctrl Pts',(3.05894968522338,139.641604608392,12.3121242422439));
#81069=CARTESIAN_POINT('Ctrl Pts',(3.06554215939757,139.719627556223,12.3648427175057));
#81070=CARTESIAN_POINT('Ctrl Pts',(3.07083120899781,139.775971951013,12.4110413421109));
#81071=CARTESIAN_POINT('Ctrl Pts',(3.08102015697254,139.874688967301,12.5085590680788));
#81072=CARTESIAN_POINT('Ctrl Pts',(3.08589031281501,139.917701954065,12.5588629897604));
#81073=CARTESIAN_POINT('Ctrl Pts',(3.09147544082007,139.963911016168,12.623138209892));
#81074=CARTESIAN_POINT('Ctrl Pts',(3.09238996024387,139.971373009591,12.6338912684786));
#81075=CARTESIAN_POINT('Ctrl Pts',(3.09383953643681,139.983054365944,12.6513385176718));
#81076=CARTESIAN_POINT('Ctrl Pts',(3.0943814968792,139.987388028676,12.6579544434954));
#81077=CARTESIAN_POINT('Ctrl Pts',(3.09546525106988,139.995991877487,12.6713825741562));
#81078=CARTESIAN_POINT('Ctrl Pts',(3.09600688713132,140.000259596855,12.6781958213678));
#81079=CARTESIAN_POINT('Ctrl Pts',(3.09746176495002,140.011622790804,12.6967565012132));
#81080=CARTESIAN_POINT('Ctrl Pts',(3.09836689536958,140.018583480987,12.7085854903961));
#81081=CARTESIAN_POINT('Ctrl Pts',(3.1037043528733,140.058844002044,12.7798244821335));
#81082=CARTESIAN_POINT('Ctrl Pts',(3.10789707547799,140.087150147747,12.841917041871));
#81083=CARTESIAN_POINT('Ctrl Pts',(3.11660390358061,140.134274451286,12.974708996856));
#81084=CARTESIAN_POINT('Ctrl Pts',(3.12110633430577,140.152203248312,13.0454043933486));
#81085=CARTESIAN_POINT('Ctrl Pts',(3.12710258391186,140.166575295225,13.1369293866387));
#81086=CARTESIAN_POINT('Ctrl Pts',(3.1284022787735,140.169160448075,13.1566343284718));
#81087=CARTESIAN_POINT('Ctrl Pts',(3.130613529084,140.172666559752,13.1898570665235));
#81088=CARTESIAN_POINT('Ctrl Pts',(3.13151658938389,140.173855052481,13.2033427910992));
#81089=CARTESIAN_POINT('Ctrl Pts',(3.13335588486105,140.1757859432,13.2306225227783));
#81090=CARTESIAN_POINT('Ctrl Pts',(3.13429227554078,140.176518637259,13.2444150519524));
#81091=CARTESIAN_POINT('Ctrl Pts',(3.13669811018278,140.177767300632,13.2795891609969));
#81092=CARTESIAN_POINT('Ctrl Pts',(3.13817781536176,140.177943699201,13.3009769358588));
#81093=CARTESIAN_POINT('Ctrl Pts',(3.14492597166112,140.176113793225,13.3973598105194));
#81094=CARTESIAN_POINT('Ctrl Pts',(3.15038878228982,140.16752732199,13.4720444052847));
#81095=CARTESIAN_POINT('Ctrl Pts',(3.15918286321279,140.142578784104,13.5891553028662));
#81096=CARTESIAN_POINT('Ctrl Pts',(3.1624741893984,140.130769465302,13.6323519161863));
#81097=CARTESIAN_POINT('Ctrl Pts',(3.16698646687943,140.110873191644,13.6916272156261));
#81098=CARTESIAN_POINT('Ctrl Pts',(3.16825890618291,140.104834800466,13.7083518745864));
#81099=CARTESIAN_POINT('Ctrl Pts',(3.17049235453672,140.093435330735,13.7378185588005));
#81100=CARTESIAN_POINT('Ctrl Pts',(3.17145936623848,140.088224315112,13.7506149071824));
#81101=CARTESIAN_POINT('Ctrl Pts',(3.17297126890723,140.079619191058,13.7707253903087));
#81102=CARTESIAN_POINT('Ctrl Pts',(3.17352407284625,140.07637325241,13.7781010583297));
#81103=CARTESIAN_POINT('Ctrl Pts',(3.17460907842506,140.069798816063,13.7926335759461));
#81104=CARTESIAN_POINT('Ctrl Pts',(3.17514140838906,140.066473596856,13.7997913779438));
#81105=CARTESIAN_POINT('Ctrl Pts',(3.17654017180158,140.057478845261,13.818654701699));
#81106=CARTESIAN_POINT('Ctrl Pts',(3.17739954485955,140.051686754446,13.8303010588967));
#81107=CARTESIAN_POINT('Ctrl Pts',(3.18319503653078,140.010899055936,13.9090162568064));
#81108=CARTESIAN_POINT('Ctrl Pts',(3.18782625949251,139.96970051007,13.9726823967365));
#81109=CARTESIAN_POINT('Ctrl Pts',(3.19641049371281,139.883404792626,14.0814623062347));
#81110=CARTESIAN_POINT('Ctrl Pts',(3.20033522734364,139.840220335692,14.1277173593056));
#81111=CARTESIAN_POINT('Ctrl Pts',(3.2057955295871,139.777654015267,14.1847662548646));
#81112=CARTESIAN_POINT('Ctrl Pts',(3.2071971611452,139.761377998941,14.1988106265807));
#81113=CARTESIAN_POINT('Ctrl Pts',(3.20953050962994,139.734012143579,14.2211474117913));
#81114=CARTESIAN_POINT('Ctrl Pts',(3.21045142993331,139.72314382849,14.2297039082591));
#81115=CARTESIAN_POINT('Ctrl Pts',(3.21227731070719,139.701482611836,14.2461478909197));
#81116=CARTESIAN_POINT('Ctrl Pts',(3.21318162661513,139.690701116982,14.2540469734759));
#81117=CARTESIAN_POINT('Ctrl Pts',(3.21543335115408,139.663740597074,14.2731031039808));
#81118=CARTESIAN_POINT('Ctrl Pts',(3.21678875017656,139.647412817364,14.2840415611368));
#81119=CARTESIAN_POINT('Ctrl Pts',(3.22454817257749,139.553442105099,14.3436440393997));
#81120=CARTESIAN_POINT('Ctrl Pts',(3.23126726862673,139.470613359239,14.3835166309028));
#81121=CARTESIAN_POINT('Ctrl Pts',(3.24063725328227,139.349936070279,14.4251399231868));
#81122=CARTESIAN_POINT('Ctrl Pts',(3.24327494504001,139.315326856751,14.4353256545533));
#81123=CARTESIAN_POINT('Ctrl Pts',(3.24699933282617,139.264994642047,14.4476590642556));
#81124=CARTESIAN_POINT('Ctrl Pts',(3.2481228561815,139.249611481914,14.4511027953175));
#81125=CARTESIAN_POINT('Ctrl Pts',(3.25012410412826,139.221777515382,14.4567495461543));
#81126=CARTESIAN_POINT('Ctrl Pts',(3.25100627506426,139.209351642828,14.4590628547352));
#81127=CARTESIAN_POINT('Ctrl Pts',(3.25241755901399,139.189181689514,14.4624828955083));
#81128=CARTESIAN_POINT('Ctrl Pts',(3.25295297300493,139.181459857275,14.4637132492362));
#81129=CARTESIAN_POINT('Ctrl Pts',(3.25403740322027,139.165665589892,14.4660687755178));
#81130=CARTESIAN_POINT('Ctrl Pts',(3.25458605855115,139.157592672277,14.4671872328251));
#81131=CARTESIAN_POINT('Ctrl Pts',(3.25608317894581,139.135360394056,14.4700325096001));
#81132=CARTESIAN_POINT('Ctrl Pts',(3.25702271025748,139.121179785555,14.4715861103672));
#81133=CARTESIAN_POINT('Ctrl Pts',(3.26206992472539,139.043999212449,14.4786254307757));
#81134=CARTESIAN_POINT('Ctrl Pts',(3.26597626222497,138.980656890449,14.4792885652085));
#81135=CARTESIAN_POINT('Ctrl Pts',(3.27310977456839,138.865508511641,14.4712087642711));
#81136=CARTESIAN_POINT('Ctrl Pts',(3.27632805108019,138.813757416287,14.4641010452671));
#81137=CARTESIAN_POINT('Ctrl Pts',(3.28113272894299,138.739296470765,14.4487807598787));
#81138=CARTESIAN_POINT('Ctrl Pts',(3.28265458379954,138.716094883765,14.4432678355518));
#81139=CARTESIAN_POINT('Ctrl Pts',(3.28550025631884,138.673618388168,14.431802260449));
#81140=CARTESIAN_POINT('Ctrl Pts',(3.28681780100397,138.654298223247,14.4260512939375));
#81141=CARTESIAN_POINT('Ctrl Pts',(3.28905030627665,138.622216897484,14.4155983204253));
#81142=CARTESIAN_POINT('Ctrl Pts',(3.28995638114752,138.609372076202,14.4111658220458));
#81143=CARTESIAN_POINT('Ctrl Pts',(3.29179435789067,138.583688219458,14.4018024539359));
#81144=CARTESIAN_POINT('Ctrl Pts',(3.29272629481365,138.570853160238,14.3968669509632));
#81145=CARTESIAN_POINT('Ctrl Pts',(3.29510456870969,138.538589229407,14.3838074376025));
#81146=CARTESIAN_POINT('Ctrl Pts',(3.29656069414595,138.519287112543,14.3753852712255));
#81147=CARTESIAN_POINT('Ctrl Pts',(3.30363154586529,138.427758085779,14.3324914178884));
#81148=CARTESIAN_POINT('Ctrl Pts',(3.30947288778961,138.358954888242,14.2912399278952));
#81149=CARTESIAN_POINT('Ctrl Pts',(3.31976884540246,138.246687697056,14.2073230276489));
#81150=CARTESIAN_POINT('Ctrl Pts',(3.32418713544667,138.20132626255,14.1676612575244));
#81151=CARTESIAN_POINT('Ctrl Pts',(3.3293289804994,138.15024866075,14.1155861806615));
#81152=CARTESIAN_POINT('Ctrl Pts',(3.33022072606745,138.141454474181,14.106323613946));
#81153=CARTESIAN_POINT('Ctrl Pts',(3.33164332530257,138.127504042292,14.0911431025031));
#81154=CARTESIAN_POINT('Ctrl Pts',(3.33218065729488,138.122253423961,14.0853136729776));
#81155=CARTESIAN_POINT('Ctrl Pts',(3.33326475098052,138.111690696451,14.0733482380002));
#81156=CARTESIAN_POINT('Ctrl Pts',(3.33381121399088,138.106383020429,14.067208980407));
#81157=CARTESIAN_POINT('Ctrl Pts',(3.33529511167421,138.092031858323,14.0502583324014));
#81158=CARTESIAN_POINT('Ctrl Pts',(3.33622387349157,138.083118013998,14.0393383383797));
#81159=CARTESIAN_POINT('Ctrl Pts',(3.34108484292572,138.036986249448,13.9807061839521));
#81160=CARTESIAN_POINT('Ctrl Pts',(3.34483233938821,138.003286588448,13.9303335909428));
#81161=CARTESIAN_POINT('Ctrl Pts',(3.35192145539169,137.947047072064,13.8303940708217));
#81162=CARTESIAN_POINT('Ctrl Pts',(3.35525618173679,137.923776416898,13.7814251357171));
#81163=CARTESIAN_POINT('Ctrl Pts',(3.35976079208708,137.897668992085,13.7150382436852));
#81164=CARTESIAN_POINT('Ctrl Pts',(3.36085355029375,137.891730902631,13.6989108969421));
#81165=CARTESIAN_POINT('Ctrl Pts',(3.36195598355709,137.886148212184,13.682660760046));
#81166=CARTESIAN_POINT('Origin',(1.13913288526384,139.,13.3));
#81167=CARTESIAN_POINT('',(3.96044919307343,137.886148212663,13.6826607614402));
#81168=CARTESIAN_POINT('',(3.86234166189399,137.886148208814,13.6826607502373));
#81169=CARTESIAN_POINT('',(1.13913288526384,137.88614821265,13.6826607614027));
#81170=CARTESIAN_POINT('',(3.48683023682326,137.822250041178,13.300311439502));
#81171=CARTESIAN_POINT('Ctrl Pts',(3.96044919307343,137.886148212676,13.6826607614778));
#81172=CARTESIAN_POINT('Ctrl Pts',(3.96015776463529,137.887508143234,13.6866192574491));
#81173=CARTESIAN_POINT('Ctrl Pts',(3.9598673740692,137.888889210441,13.6905706046321));
#81174=CARTESIAN_POINT('Ctrl Pts',(3.95902514688492,137.892971474364,13.7020533816354));
#81175=CARTESIAN_POINT('Ctrl Pts',(3.95847628523608,137.895728441424,13.7095649065459));
#81176=CARTESIAN_POINT('Ctrl Pts',(3.95739856836759,137.901338771655,13.7243819812995));
#81177=CARTESIAN_POINT('Ctrl Pts',(3.9568695917225,137.904188957588,13.7316882291937));
#81178=CARTESIAN_POINT('Ctrl Pts',(3.95548012561848,137.911925627858,13.7509501318349));
#81179=CARTESIAN_POINT('Ctrl Pts',(3.95462659678981,137.916936314258,13.7628552121782));
#81180=CARTESIAN_POINT('Ctrl Pts',(3.95004470906071,137.945179112336,13.8269867884242));
#81181=CARTESIAN_POINT('Ctrl Pts',(3.94648761168793,137.971996572454,13.8775575001408));
#81182=CARTESIAN_POINT('Ctrl Pts',(3.93778423811119,138.046745328549,13.996682584095));
#81183=CARTESIAN_POINT('Ctrl Pts',(3.93266995385278,138.098491056627,14.0624573599495));
#81184=CARTESIAN_POINT('Ctrl Pts',(3.92594424512489,138.171173226379,14.136999392843));
#81185=CARTESIAN_POINT('Ctrl Pts',(3.92459527004339,138.185980641409,14.1514071907126));
#81186=CARTESIAN_POINT('Ctrl Pts',(3.92232926683204,138.211164474853,14.1746536465654));
#81187=CARTESIAN_POINT('Ctrl Pts',(3.92142188797792,138.22132943502,14.1837152325005));
#81188=CARTESIAN_POINT('Ctrl Pts',(3.91959724557429,138.241912327093,14.201433045302));
#81189=CARTESIAN_POINT('Ctrl Pts',(3.91868020238066,138.252327007952,14.2100898446223));
#81190=CARTESIAN_POINT('Ctrl Pts',(3.9163738095617,138.278678201926,14.2312356291197));
#81191=CARTESIAN_POINT('Ctrl Pts',(3.91497574236692,138.294791303743,14.2434964438661));
#81192=CARTESIAN_POINT('Ctrl Pts',(3.90857607814368,138.369128731626,14.2970930849324));
#81193=CARTESIAN_POINT('Ctrl Pts',(3.90339699772107,138.430714388301,14.3334912300905));
#81194=CARTESIAN_POINT('Ctrl Pts',(3.89311766151282,138.557269618509,14.3935280693941));
#81195=CARTESIAN_POINT('Ctrl Pts',(3.88804368875238,138.621794456477,14.4174863569865));
#81196=CARTESIAN_POINT('Ctrl Pts',(3.88222344565931,138.701215876073,14.4393022889455));
#81197=CARTESIAN_POINT('Ctrl Pts',(3.88126754943301,138.714450664671,14.4426912425384));
#81198=CARTESIAN_POINT('Ctrl Pts',(3.87977095098395,138.735520494207,14.4476975091276));
#81199=CARTESIAN_POINT('Ctrl Pts',(3.87922252781066,138.743317783362,14.4494664982435));
#81200=CARTESIAN_POINT('Ctrl Pts',(3.87814490592969,138.758802919911,14.4528142139738));
#81201=CARTESIAN_POINT('Ctrl Pts',(3.87761559652486,138.766489678663,14.4543957642497));
#81202=CARTESIAN_POINT('Ctrl Pts',(3.8762240980337,138.786892901242,14.45838158592));
#81203=CARTESIAN_POINT('Ctrl Pts',(3.87536890679318,138.79963458745,14.4606533805918));
#81204=CARTESIAN_POINT('Ctrl Pts',(3.87058201000085,138.871916405253,14.4723150692809));
#81205=CARTESIAN_POINT('Ctrl Pts',(3.86684152384165,138.93207770322,14.4773344184108));
#81206=CARTESIAN_POINT('Ctrl Pts',(3.85819792898884,139.071844141519,14.4782405035428));
#81207=CARTESIAN_POINT('Ctrl Pts',(3.85331561147581,139.151163420014,14.4707093713224));
#81208=CARTESIAN_POINT('Ctrl Pts',(3.84682729065043,139.249766186659,14.4511538051818));
#81209=CARTESIAN_POINT('Ctrl Pts',(3.84545358254944,139.270300942082,14.4465057974875));
#81210=CARTESIAN_POINT('Ctrl Pts',(3.843157867969,139.303965112743,14.4379313141833));
#81211=CARTESIAN_POINT('Ctrl Pts',(3.84224607310668,139.317170664146,14.4343214750324));
#81212=CARTESIAN_POINT('Ctrl Pts',(3.84042158748146,139.343247417855,14.4267022424632));
#81213=CARTESIAN_POINT('Ctrl Pts',(3.8395092642167,139.356118658441,14.4227004087814));
#81214=CARTESIAN_POINT('Ctrl Pts',(3.83723270299145,139.387804862289,14.4122490619253));
#81215=CARTESIAN_POINT('Ctrl Pts',(3.83586023482043,139.406529892719,14.4055423779088));
#81216=CARTESIAN_POINT('Ctrl Pts',(3.82960759071628,139.490101878828,14.3731994202034));
#81217=CARTESIAN_POINT('Ctrl Pts',(3.82455807089613,139.552755321523,14.3423126266406));
#81218=CARTESIAN_POINT('Ctrl Pts',(3.8141963485541,139.673431807308,14.2688683247508));
#81219=CARTESIAN_POINT('Ctrl Pts',(3.80890316081983,139.731048497991,14.2261672294806));
#81220=CARTESIAN_POINT('Ctrl Pts',(3.80290028417302,139.794450651987,14.169553632052));
#81221=CARTESIAN_POINT('Ctrl Pts',(3.80196116231918,139.804313168165,14.1604392619546));
#81222=CARTESIAN_POINT('Ctrl Pts',(3.80048448420287,139.819761473143,14.1456650312962));
#81223=CARTESIAN_POINT('Ctrl Pts',(3.79993953222665,139.825449259723,14.1401141273428));
#81224=CARTESIAN_POINT('Ctrl Pts',(3.79886253248985,139.836671893302,14.1289375572586));
#81225=CARTESIAN_POINT('Ctrl Pts',(3.79833046011748,139.842207243204,14.1233130017159));
#81226=CARTESIAN_POINT('Ctrl Pts',(3.79692220936045,139.856818795379,14.108164389781));
#81227=CARTESIAN_POINT('Ctrl Pts',(3.79605333733977,139.865792948763,14.098542882218));
#81228=CARTESIAN_POINT('Ctrl Pts',(3.79211768698261,139.90613538509,14.0538104998538));
#81229=CARTESIAN_POINT('Ctrl Pts',(3.78916301506082,139.935545025994,14.0169853870527));
#81230=CARTESIAN_POINT('Ctrl Pts',(3.78036759505297,140.017124249449,13.9012377717556));
#81231=CARTESIAN_POINT('Ctrl Pts',(3.77462167143407,140.062072970699,13.8177145472912));
#81232=CARTESIAN_POINT('Ctrl Pts',(3.76721354109111,140.103851055827,13.7111053363814));
#81233=CARTESIAN_POINT('Ctrl Pts',(3.76590638509228,140.110669994167,13.6923096208639));
#81234=CARTESIAN_POINT('Ctrl Pts',(3.76377952641901,140.120858627309,13.6618267917514));
#81235=CARTESIAN_POINT('Ctrl Pts',(3.76296986172559,140.124531594255,13.65024472087));
#81236=CARTESIAN_POINT('Ctrl Pts',(3.76125396351118,140.131880709298,13.6257622031382));
#81237=CARTESIAN_POINT('Ctrl Pts',(3.7603465663144,140.135516947882,13.6128517033324));
#81238=CARTESIAN_POINT('Ctrl Pts',(3.7581015738672,140.143899111256,13.5810168466342));
#81239=CARTESIAN_POINT('Ctrl Pts',(3.75675625709921,140.148396650425,13.5620318659954));
#81240=CARTESIAN_POINT('Ctrl Pts',(3.75044123120765,140.167082814234,13.4733931797274));
#81241=CARTESIAN_POINT('Ctrl Pts',(3.74529334605313,140.175416456501,13.4026677939246));
#81242=CARTESIAN_POINT('Ctrl Pts',(3.73487808904619,140.179230029919,13.2607371967239));
#81243=CARTESIAN_POINT('Ctrl Pts',(3.72963381280529,140.174727340141,13.1898087607957));
#81244=CARTESIAN_POINT('Ctrl Pts',(3.72367069765558,140.161804126306,13.1063812395129));
#81245=CARTESIAN_POINT('Ctrl Pts',(3.72272703590348,140.159510037494,13.0930856111926));
#81246=CARTESIAN_POINT('Ctrl Pts',(3.72124496447285,140.155499837138,13.0720119503117));
#81247=CARTESIAN_POINT('Ctrl Pts',(3.72069907154485,140.153932499023,13.0642072488425));
#81248=CARTESIAN_POINT('Ctrl Pts',(3.71962192658602,140.150656598908,13.0487102669889));
#81249=CARTESIAN_POINT('Ctrl Pts',(3.71909062639947,140.148949741658,13.0410180744253));
#81250=CARTESIAN_POINT('Ctrl Pts',(3.71768703672218,140.144200701203,13.0205875454658));
#81251=CARTESIAN_POINT('Ctrl Pts',(3.71682196743311,140.1410229364,13.0078814309226));
#81252=CARTESIAN_POINT('Ctrl Pts',(3.71210761707385,140.122354549357,12.9381967205246));
#81253=CARTESIAN_POINT('Ctrl Pts',(3.70844041445968,140.1028061407,12.8823858134711));
#81254=CARTESIAN_POINT('Ctrl Pts',(3.6998004201543,140.046857668103,12.7543951504766));
#81255=CARTESIAN_POINT('Ctrl Pts',(3.69485131314189,140.007067153053,12.6840374098686));
#81256=CARTESIAN_POINT('Ctrl Pts',(3.68829417997797,139.948278366409,12.6012138331182));
#81257=CARTESIAN_POINT('Ctrl Pts',(3.6869268460941,139.935699084951,12.5844574767372));
#81258=CARTESIAN_POINT('Ctrl Pts',(3.68463879650462,139.914184062106,12.5573362449958));
#81259=CARTESIAN_POINT('Ctrl Pts',(3.68372814649029,139.905502373739,12.5467753475822));
#81260=CARTESIAN_POINT('Ctrl Pts',(3.68190367393702,139.887889679922,12.5260949190062));
#81261=CARTESIAN_POINT('Ctrl Pts',(3.68099018158458,139.878964649269,12.515973038045));
#81262=CARTESIAN_POINT('Ctrl Pts',(3.67870619779968,139.856400404893,12.4912525225724));
#81263=CARTESIAN_POINT('Ctrl Pts',(3.67732735551821,139.842560370669,12.4768438346986));
#81264=CARTESIAN_POINT('Ctrl Pts',(3.67094858481372,139.777587840458,12.4125576460861));
#81265=CARTESIAN_POINT('Ctrl Pts',(3.66577010803782,139.722357453954,12.3670511700812));
#81266=CARTESIAN_POINT('Ctrl Pts',(3.65544480934813,139.606085562461,12.2877949039917));
#81267=CARTESIAN_POINT('Ctrl Pts',(3.65032375135953,139.545477530907,12.2538859999674));
#81268=CARTESIAN_POINT('Ctrl Pts',(3.64446311470459,139.46980635545,12.2199247031927));
#81269=CARTESIAN_POINT('Ctrl Pts',(3.64350986180661,139.457280816154,12.214562321617));
#81270=CARTESIAN_POINT('Ctrl Pts',(3.64201640107588,139.437268164405,12.2064025359347));
#81271=CARTESIAN_POINT('Ctrl Pts',(3.64146852387238,139.429841171078,12.2034620671792));
#81272=CARTESIAN_POINT('Ctrl Pts',(3.64039101527643,139.415053050234,12.1977805513095));
#81273=CARTESIAN_POINT('Ctrl Pts',(3.63986128658951,139.407693323009,12.1950371456818));
#81274=CARTESIAN_POINT('Ctrl Pts',(3.6384672320587,139.388105049335,12.1879578005358));
#81275=CARTESIAN_POINT('Ctrl Pts',(3.63760995092967,139.375830959692,12.1837498009107));
#81276=CARTESIAN_POINT('Ctrl Pts',(3.63289601013944,139.307243035411,12.1614950666583));
#81277=CARTESIAN_POINT('Ctrl Pts',(3.62922284791983,139.249695234406,12.1475045697928));
#81278=CARTESIAN_POINT('Ctrl Pts',(3.62056617207898,139.111604178754,12.1247686468326));
#81279=CARTESIAN_POINT('Ctrl Pts',(3.61560673885947,139.030743099405,12.1198823701455));
#81280=CARTESIAN_POINT('Ctrl Pts',(3.60903900459623,138.929107147146,12.1241992199487));
#81281=CARTESIAN_POINT('Ctrl Pts',(3.60767271457875,138.908221097989,12.1256449356169));
#81282=CARTESIAN_POINT('Ctrl Pts',(3.60538591974876,138.873780571632,12.1289532355704));
#81283=CARTESIAN_POINT('Ctrl Pts',(3.60447545679667,138.860199782263,12.1304967972824));
#81284=CARTESIAN_POINT('Ctrl Pts',(3.6026509829604,138.833267393687,12.1340336767718));
#81285=CARTESIAN_POINT('Ctrl Pts',(3.60173729611322,138.819917097004,12.1360208977051));
#81286=CARTESIAN_POINT('Ctrl Pts',(3.59945207975801,138.786884142316,12.1415198069981));
#81287=CARTESIAN_POINT('Ctrl Pts',(3.59807217932877,138.767251825228,12.1453039671509));
#81288=CARTESIAN_POINT('Ctrl Pts',(3.59170956579801,138.678201420607,12.1648317784664));
#81289=CARTESIAN_POINT('Ctrl Pts',(3.58654976558408,138.610212418041,12.1863465906194));
#81290=CARTESIAN_POINT('Ctrl Pts',(3.57622490560696,138.480442781481,12.2407579136326));
#81291=CARTESIAN_POINT('Ctrl Pts',(3.57108479195691,138.418799135787,12.2732865867026));
#81292=CARTESIAN_POINT('Ctrl Pts',(3.56520802955033,138.348959074238,12.318457388931));
#81293=CARTESIAN_POINT('Ctrl Pts',(3.56425603221813,138.337662720374,12.3260443786691));
#81294=CARTESIAN_POINT('Ctrl Pts',(3.56276406206246,138.31995022417,12.3383913965552));
#81295=CARTESIAN_POINT('Ctrl Pts',(3.56221644432537,138.313447001667,12.3430236190217));
#81296=CARTESIAN_POINT('Ctrl Pts',(3.56113898754398,138.300638180529,12.3523450822805));
#81297=CARTESIAN_POINT('Ctrl Pts',(3.56060905759279,138.294331441897,12.357031977602));
#81298=CARTESIAN_POINT('Ctrl Pts',(3.5592137781077,138.277724190548,12.3696337038068));
#81299=CARTESIAN_POINT('Ctrl Pts',(3.55835549577434,138.267506567273,12.3776566823256));
#81300=CARTESIAN_POINT('Ctrl Pts',(3.5564354978976,138.244709044667,12.3961753753526));
#81301=CARTESIAN_POINT('Ctrl Pts',(3.5553793500769,138.232211034531,12.406767926361));
#81302=CARTESIAN_POINT('Ctrl Pts',(3.5518658918916,138.190965416043,12.4432307864417));
#81303=CARTESIAN_POINT('Ctrl Pts',(3.54945897851472,138.163270519238,12.4702563109205));
#81304=CARTESIAN_POINT('Ctrl Pts',(3.54173447847104,138.078385651491,12.5616704197462));
#81305=CARTESIAN_POINT('Ctrl Pts',(3.53646858814523,138.026913350294,12.6309675312097));
#81306=CARTESIAN_POINT('Ctrl Pts',(3.52958953609531,137.973176913908,12.7228142105224));
#81307=CARTESIAN_POINT('Ctrl Pts',(3.52826004731341,137.963359056369,12.7406391510084));
#81308=CARTESIAN_POINT('Ctrl Pts',(3.52601738952816,137.947775802657,12.7707522381477));
#81309=CARTESIAN_POINT('Ctrl Pts',(3.52511343399577,137.941752039337,12.782902153663));
#81310=CARTESIAN_POINT('Ctrl Pts',(3.52328824497287,137.93011090896,12.8074380320375));
#81311=CARTESIAN_POINT('Ctrl Pts',(3.52236711111442,137.924495626892,12.819822662089));
#81312=CARTESIAN_POINT('Ctrl Pts',(3.52003511523346,137.910934975582,12.8511628372026));
#81313=CARTESIAN_POINT('Ctrl Pts',(3.51861511185837,137.90326930228,12.8702336560898));
#81314=CARTESIAN_POINT('Ctrl Pts',(3.51546510033011,137.88755743913,12.9124845090497));
#81315=CARTESIAN_POINT('Ctrl Pts',(3.51372902428973,137.879728870532,12.9357347661782));
#81316=CARTESIAN_POINT('Ctrl Pts',(3.50803170725098,137.856689738697,13.0119507942234));
#81317=CARTESIAN_POINT('Ctrl Pts',(3.50399726602573,137.844468960527,13.0657399807676));
#81318=CARTESIAN_POINT('Ctrl Pts',(3.49552094071799,137.826850658652,13.179781295226));
#81319=CARTESIAN_POINT('Ctrl Pts',(3.49108936154799,137.82223409131,13.2399948902523));
#81320=CARTESIAN_POINT('Ctrl Pts',(3.48683023682335,137.822250041178,13.300311439502));
#81321=CARTESIAN_POINT('Ctrl Pts',(3.48683023682336,137.822250041178,13.3003114395019));
#81322=CARTESIAN_POINT('Ctrl Pts',(3.48596619464028,137.822253276903,13.3125477665077));
#81323=CARTESIAN_POINT('Ctrl Pts',(3.48511045956081,137.822446998391,13.3247739288273));
#81324=CARTESIAN_POINT('Ctrl Pts',(3.48378069926075,137.823050592295,13.3439746885546));
#81325=CARTESIAN_POINT('Ctrl Pts',(3.48330109326705,137.8233315726,13.3509421207309));
#81326=CARTESIAN_POINT('Ctrl Pts',(3.48232487836774,137.824034391365,13.3652192482236));
#81327=CARTESIAN_POINT('Ctrl Pts',(3.48182878743761,137.824462509499,13.3725277516578));
#81328=CARTESIAN_POINT('Ctrl Pts',(3.48062054569804,137.825680116448,13.3904495324128));
#81329=CARTESIAN_POINT('Ctrl Pts',(3.47991244642756,137.826545343786,13.4010568989226));
#81330=CARTESIAN_POINT('Ctrl Pts',(3.4773123081919,137.830284806035,13.4403247518565));
#81331=CARTESIAN_POINT('Ctrl Pts',(3.47546267205911,137.834066512121,13.4688906677266));
#81332=CARTESIAN_POINT('Ctrl Pts',(3.47172975987481,137.84395172549,13.5270675258845));
#81333=CARTESIAN_POINT('Ctrl Pts',(3.46985054954414,137.850154913566,13.5566392528942));
#81334=CARTESIAN_POINT('Ctrl Pts',(3.46677831503639,137.862197397912,13.6047564622898));
#81335=CARTESIAN_POINT('Ctrl Pts',(3.46558093876604,137.8673705408,13.6234528984423));
#81336=CARTESIAN_POINT('Ctrl Pts',(3.46350161923839,137.877140051955,13.6556452581504));
#81337=CARTESIAN_POINT('Ctrl Pts',(3.46262081792885,137.881522651725,13.6691966452519));
#81338=CARTESIAN_POINT('Ctrl Pts',(3.46173780698925,137.886148221013,13.6826607857451));
#81339=CARTESIAN_POINT('Ctrl Pts',(3.36195598355709,137.886148212184,13.682660760046));
#81340=CARTESIAN_POINT('Ctrl Pts',(3.36241237182347,137.883837075084,13.6759334849782));
#81341=CARTESIAN_POINT('Ctrl Pts',(3.36287041208775,137.881586846862,13.6691851655125));
#81342=CARTESIAN_POINT('Ctrl Pts',(3.3646512225657,137.873108986812,13.6429713885228));
#81343=CARTESIAN_POINT('Ctrl Pts',(3.36598643499762,137.867327686068,13.6233667838123));
#81344=CARTESIAN_POINT('Ctrl Pts',(3.36824003654619,137.858543767653,13.5904457321609));
#81345=CARTESIAN_POINT('Ctrl Pts',(3.36914914820719,137.855257213339,13.5772092705302));
#81346=CARTESIAN_POINT('Ctrl Pts',(3.37098619450111,137.849132410593,13.5505721754297));
#81347=CARTESIAN_POINT('Ctrl Pts',(3.37191404927104,137.8462966229,13.5371731720421));
#81348=CARTESIAN_POINT('Ctrl Pts',(3.37426695052869,137.839752734046,13.5033520960691));
#81349=CARTESIAN_POINT('Ctrl Pts',(3.37570135621474,137.836349759909,13.4828765067076));
#81350=CARTESIAN_POINT('Ctrl Pts',(3.3829584133633,137.822041920829,13.3800551942519));
#81351=CARTESIAN_POINT('Ctrl Pts',(3.38902897133321,137.819330863159,13.2968199616939));
#81352=CARTESIAN_POINT('Ctrl Pts',(3.39807601646271,137.828323987451,13.1739792352492));
#81353=CARTESIAN_POINT('Ctrl Pts',(3.40102047205989,137.833298792102,13.1341250377483));
#81354=CARTESIAN_POINT('Ctrl Pts',(3.40511781261743,137.843220397392,13.0781067613406));
#81355=CARTESIAN_POINT('Ctrl Pts',(3.40631434047634,137.846493477373,13.0616758138232));
#81356=CARTESIAN_POINT('Ctrl Pts',(3.4084299222341,137.852975258874,13.0324105356111));
#81357=CARTESIAN_POINT('Ctrl Pts',(3.40935416190632,137.856051713428,13.0195499459066));
#81358=CARTESIAN_POINT('Ctrl Pts',(3.4108152745144,137.861320269585,12.9990572938999));
#81359=CARTESIAN_POINT('Ctrl Pts',(3.41135923425297,137.863373999396,12.9913912091947));
#81360=CARTESIAN_POINT('Ctrl Pts',(3.4124430282484,137.867655756815,12.9760312951153));
#81361=CARTESIAN_POINT('Ctrl Pts',(3.41298276217872,137.869885085676,12.9683382796906));
#81362=CARTESIAN_POINT('Ctrl Pts',(3.41442621482104,137.876104644351,12.9476668731876));
#81363=CARTESIAN_POINT('Ctrl Pts',(3.41532203935336,137.880241225149,12.934733346848));
#81364=CARTESIAN_POINT('Ctrl Pts',(3.42079692728527,137.907177593431,12.8552763113865));
#81365=CARTESIAN_POINT('Ctrl Pts',(3.42511868834227,137.935676453949,12.7908263511326));
#81366=CARTESIAN_POINT('Ctrl Pts',(3.43380871729351,138.003818548769,12.667815068597));
#81367=CARTESIAN_POINT('Ctrl Pts',(3.43816263513904,138.043308840823,12.6095104157656));
#81368=CARTESIAN_POINT('Ctrl Pts',(3.44401017102428,138.100487858893,12.5394883225751));
#81369=CARTESIAN_POINT('Ctrl Pts',(3.44532582852851,138.113614072183,12.5242294072873));
#81370=CARTESIAN_POINT('Ctrl Pts',(3.44755608421039,138.136242641866,12.4992486236562));
#81371=CARTESIAN_POINT('Ctrl Pts',(3.44846183822241,138.145534236986,12.4893411481007));
#81372=CARTESIAN_POINT('Ctrl Pts',(3.45029993731405,138.164577671986,12.4697266410326));
#81373=CARTESIAN_POINT('Ctrl Pts',(3.45123232997283,138.174332402686,12.4600254125638));
#81374=CARTESIAN_POINT('Ctrl Pts',(3.45361342668149,138.199467048716,12.4358895471716));
#81375=CARTESIAN_POINT('Ctrl Pts',(3.45507196727483,138.215068356333,12.4216936207663));
#81376=CARTESIAN_POINT('Ctrl Pts',(3.46309465989909,138.301931639212,12.3468184662482));
#81377=CARTESIAN_POINT('Ctrl Pts',(3.4699820893236,138.379842980158,12.294388804727));
#81378=CARTESIAN_POINT('Ctrl Pts',(3.48036913911613,138.505937879985,12.2298073432981));
#81379=CARTESIAN_POINT('Ctrl Pts',(3.48387180715933,138.550067040572,12.2105180379852));
#81380=CARTESIAN_POINT('Ctrl Pts',(3.48809896371012,138.606513260801,12.1898617500924));
#81381=CARTESIAN_POINT('Ctrl Pts',(3.48893427713972,138.617832876857,12.1859142464915));
#81382=CARTESIAN_POINT('Ctrl Pts',(3.49028523651756,138.636443087598,12.1797413306903));
#81383=CARTESIAN_POINT('Ctrl Pts',(3.4908064053045,138.643698310538,12.1774127054966));
#81384=CARTESIAN_POINT('Ctrl Pts',(3.49188745750944,138.65891671153,12.1726906470384));
#81385=CARTESIAN_POINT('Ctrl Pts',(3.49244659286099,138.666883520382,12.1703108354951));
#81386=CARTESIAN_POINT('Ctrl Pts',(3.49400742384673,138.689369390241,12.1638525184366));
#81387=CARTESIAN_POINT('Ctrl Pts',(3.49499888336913,138.703943070141,12.159968061096));
#81388=CARTESIAN_POINT('Ctrl Pts',(3.4972815514475,138.738055901977,12.1515739931941));
#81389=CARTESIAN_POINT('Ctrl Pts',(3.49856357481888,138.757643883482,12.1472812119887));
#81390=CARTESIAN_POINT('Ctrl Pts',(3.50341875097642,138.832996659859,12.1327732635331));
#81391=CARTESIAN_POINT('Ctrl Pts',(3.50689443931797,138.889364323222,12.1260882507653));
#81392=CARTESIAN_POINT('Ctrl Pts',(3.51403761257599,139.004676866257,12.1207952662246));
#81393=CARTESIAN_POINT('Ctrl Pts',(3.51769866205715,139.063470571353,12.1224957895716));
#81394=CARTESIAN_POINT('Ctrl Pts',(3.52286147547534,139.143063494294,12.130777553757));
#81395=CARTESIAN_POINT('Ctrl Pts',(3.52425019959525,139.164173581776,12.1335544435307));
#81396=CARTESIAN_POINT('Ctrl Pts',(3.52656800458119,139.19881782905,12.1390707183034));
#81397=CARTESIAN_POINT('Ctrl Pts',(3.52748658991739,139.212400174396,12.1414787594018));
#81398=CARTESIAN_POINT('Ctrl Pts',(3.52932282082344,139.239236747527,12.1467244504931));
#81399=CARTESIAN_POINT('Ctrl Pts',(3.5302400612073,139.252490500797,12.1495534628818));
#81400=CARTESIAN_POINT('Ctrl Pts',(3.53252607210383,139.285130803349,12.1571117223191));
#81401=CARTESIAN_POINT('Ctrl Pts',(3.53390309486758,139.304450947544,12.1621060128241));
#81402=CARTESIAN_POINT('Ctrl Pts',(3.54019137834316,139.391098824605,12.1868692633379));
#81403=CARTESIAN_POINT('Ctrl Pts',(3.54527426339156,139.456695396699,12.2121375057453));
#81404=CARTESIAN_POINT('Ctrl Pts',(3.55562246577164,139.583290210715,12.274379399949));
#81405=CARTESIAN_POINT('Ctrl Pts',(3.56086681788583,139.643983682482,12.3113587598672));
#81406=CARTESIAN_POINT('Ctrl Pts',(3.56683243050722,139.711850679058,12.3616255883316));
#81407=CARTESIAN_POINT('Ctrl Pts',(3.56777836572911,139.722578492947,12.3698611466092));
#81408=CARTESIAN_POINT('Ctrl Pts',(3.56926525265173,139.739421798109,12.3832587978587));
#81409=CARTESIAN_POINT('Ctrl Pts',(3.5698137054281,139.745630317725,12.3883013293743));
#81410=CARTESIAN_POINT('Ctrl Pts',(3.57089791418575,139.757904212338,12.3984793872533));
#81411=CARTESIAN_POINT('Ctrl Pts',(3.57143369004956,139.763969925577,12.4036138266559));
#81412=CARTESIAN_POINT('Ctrl Pts',(3.57285338884438,139.780027452261,12.417487435491));
#81413=CARTESIAN_POINT('Ctrl Pts',(3.57372986304751,139.789924595509,12.4263350625362));
#81414=CARTESIAN_POINT('Ctrl Pts',(3.578456686363,139.843053967571,12.4754716197305));
#81415=CARTESIAN_POINT('Ctrl Pts',(3.58212575599146,139.883361452405,12.5188078193927));
#81416=CARTESIAN_POINT('Ctrl Pts',(3.59073898875675,139.970271904251,12.6276218639937));
#81417=CARTESIAN_POINT('Ctrl Pts',(3.59566049872391,140.013766105479,12.6951886647184));
#81418=CARTESIAN_POINT('Ctrl Pts',(3.6021924666431,140.059591321606,12.7854087275828));
#81419=CARTESIAN_POINT('Ctrl Pts',(3.60356585260536,140.068616515949,12.804422962466));
#81420=CARTESIAN_POINT('Ctrl Pts',(3.60586521440667,140.082687572064,12.8362417593078));
#81421=CARTESIAN_POINT('Ctrl Pts',(3.6067810488211,140.088027252898,12.8489115890893));
#81422=CARTESIAN_POINT('Ctrl Pts',(3.60861723779828,140.098201413881,12.874284845953));
#81423=CARTESIAN_POINT('Ctrl Pts',(3.60953727726179,140.103040208997,12.8869842518208));
#81424=CARTESIAN_POINT('Ctrl Pts',(3.61184108729313,140.114511259055,12.9187305300396));
#81425=CARTESIAN_POINT('Ctrl Pts',(3.6132334013076,140.120875835878,12.9378687691318));
#81426=CARTESIAN_POINT('Ctrl Pts',(3.61924604796346,140.145946437036,13.0202634392441));
#81427=CARTESIAN_POINT('Ctrl Pts',(3.62401479966679,140.159809358087,13.084859005461));
#81428=CARTESIAN_POINT('Ctrl Pts',(3.63439034052384,140.177808784029,13.2252865173418));
#81429=CARTESIAN_POINT('Ctrl Pts',(3.63999523230505,140.180176251222,13.3010633326068));
#81430=CARTESIAN_POINT('Ctrl Pts',(3.64624858796237,140.174414308321,13.3895282399384));
#81431=CARTESIAN_POINT('Ctrl Pts',(3.64715742750856,140.173353807826,13.4024946358839));
#81432=CARTESIAN_POINT('Ctrl Pts',(3.64860026944275,140.171305031423,13.4232958898383));
#81433=CARTESIAN_POINT('Ctrl Pts',(3.64914106889275,140.170452458468,13.4311426955614));
#81434=CARTESIAN_POINT('Ctrl Pts',(3.65022485608359,140.168570225911,13.4469816631424));
#81435=CARTESIAN_POINT('Ctrl Pts',(3.65076765180375,140.167537309942,13.4549729708839));
#81436=CARTESIAN_POINT('Ctrl Pts',(3.65222948327559,140.16451138398,13.476632593384));
#81437=CARTESIAN_POINT('Ctrl Pts',(3.65314027461669,140.162359753237,13.4902779057982));
#81438=CARTESIAN_POINT('Ctrl Pts',(3.65849884545204,140.148134453274,13.5712111136521));
#81439=CARTESIAN_POINT('Ctrl Pts',(3.66270592696095,140.13045951786,13.6373895818358));
#81440=CARTESIAN_POINT('Ctrl Pts',(3.67119864960379,140.083586309109,13.7665891470757));
#81441=CARTESIAN_POINT('Ctrl Pts',(3.67547120883528,140.054370517278,13.8293073323675));
#81442=CARTESIAN_POINT('Ctrl Pts',(3.68130814915284,140.00910199199,13.9076744869996));
#81443=CARTESIAN_POINT('Ctrl Pts',(3.68270688660635,139.997868707795,13.9259497275824));
#81444=CARTESIAN_POINT('Ctrl Pts',(3.68503674684559,139.978585767844,13.9554815316255));
#81445=CARTESIAN_POINT('Ctrl Pts',(3.68595714072617,139.970825358354,13.9669214642655));
#81446=CARTESIAN_POINT('Ctrl Pts',(3.68779350536935,139.955075094265,13.9892819802223));
#81447=CARTESIAN_POINT('Ctrl Pts',(3.68870901336687,139.947094824133,14.0002067205409));
#81448=CARTESIAN_POINT('Ctrl Pts',(3.6909839352324,139.92696338637,14.0267921120005));
#81449=CARTESIAN_POINT('Ctrl Pts',(3.6923514210906,139.91460207103,14.0422875873205));
#81450=CARTESIAN_POINT('Ctrl Pts',(3.69856311300457,139.857331980322,14.1104749330372));
#81451=CARTESIAN_POINT('Ctrl Pts',(3.70357422042904,139.808227123204,14.1594497745731));
#81452=CARTESIAN_POINT('Ctrl Pts',(3.71396196866625,139.69952420593,14.250267498483));
#81453=CARTESIAN_POINT('Ctrl Pts',(3.71932219536306,139.639763858105,14.2914867961921));
#81454=CARTESIAN_POINT('Ctrl Pts',(3.72538139581134,139.564935664206,14.333499606884));
#81455=CARTESIAN_POINT('Ctrl Pts',(3.72631611186194,139.553168827342,14.3398451945717));
#81456=CARTESIAN_POINT('Ctrl Pts',(3.72778966891356,139.534221328444,14.3496504597366));
#81457=CARTESIAN_POINT('Ctrl Pts',(3.72833579527716,139.527109531827,14.3532397953035));
#81458=CARTESIAN_POINT('Ctrl Pts',(3.72941973324274,139.512803151647,14.3602790385105));
#81459=CARTESIAN_POINT('Ctrl Pts',(3.72995750469923,139.505608834922,14.3637285496196));
#81460=CARTESIAN_POINT('Ctrl Pts',(3.73138919203561,139.486214288058,14.3727865628801));
#81461=CARTESIAN_POINT('Ctrl Pts',(3.73227543482366,139.473951904242,14.378260160526));
#81462=CARTESIAN_POINT('Ctrl Pts',(3.73683763652325,139.40966221112,14.4056485847371));
#81463=CARTESIAN_POINT('Ctrl Pts',(3.74034992680729,139.356196658669,14.4240139296472));
#81464=CARTESIAN_POINT('Ctrl Pts',(3.74898877104284,139.221252018408,14.4597646392731));
#81465=CARTESIAN_POINT('Ctrl Pts',(3.75408385317169,139.13886923152,14.4724846800504));
#81466=CARTESIAN_POINT('Ctrl Pts',(3.76079320739871,139.035115397669,14.4774091526065));
#81467=CARTESIAN_POINT('Ctrl Pts',(3.76214774979994,139.014372791898,14.4778449566465));
#81468=CARTESIAN_POINT('Ctrl Pts',(3.76442449573541,138.979937075474,14.477658717995));
#81469=CARTESIAN_POINT('Ctrl Pts',(3.76533698738087,138.966246528022,14.4773458512391));
#81470=CARTESIAN_POINT('Ctrl Pts',(3.76717341750225,138.938936596162,14.4762450250355));
#81471=CARTESIAN_POINT('Ctrl Pts',(3.76809715491837,138.925319267852,14.4754589993785));
#81472=CARTESIAN_POINT('Ctrl Pts',(3.77042428982301,138.89133070851,14.4729041242417));
#81473=CARTESIAN_POINT('Ctrl Pts',(3.77183661596766,138.870986829986,14.4708409842814));
#81474=CARTESIAN_POINT('Ctrl Pts',(3.77496332499627,138.826589667418,14.4651674184899));
#81475=CARTESIAN_POINT('Ctrl Pts',(3.77668356875944,138.802574083427,14.4613393666294));
#81476=CARTESIAN_POINT('Ctrl Pts',(3.78230049541797,138.725440305582,14.4465827306297));
#81477=CARTESIAN_POINT('Ctrl Pts',(3.78626816478442,138.672956510601,14.4327297149224));
#81478=CARTESIAN_POINT('Ctrl Pts',(3.79468713727952,138.564413637379,14.3959053673396));
#81479=CARTESIAN_POINT('Ctrl Pts',(3.79913018828996,138.508782442564,14.3721243087026));
#81480=CARTESIAN_POINT('Ctrl Pts',(3.80440142765512,138.44271891374,14.3376567850524));
#81481=CARTESIAN_POINT('Ctrl Pts',(3.80538886508177,138.430337307749,14.3309113801462));
#81482=CARTESIAN_POINT('Ctrl Pts',(3.80692498298134,138.411023250858,14.3199349571874));
#81483=CARTESIAN_POINT('Ctrl Pts',(3.80748198290369,138.404008723537,14.3158520247486));
#81484=CARTESIAN_POINT('Ctrl Pts',(3.80856808693406,138.390298207881,14.3076806654435));
#81485=CARTESIAN_POINT('Ctrl Pts',(3.80909742091858,138.383599843808,14.3035972560907));
#81486=CARTESIAN_POINT('Ctrl Pts',(3.81047768361035,138.366107611113,14.2926925621302));
#81487=CARTESIAN_POINT('Ctrl Pts',(3.81132189109702,138.355382621629,14.2857619145525));
#81488=CARTESIAN_POINT('Ctrl Pts',(3.81608774883458,138.294848230974,14.245233111747));
#81489=CARTESIAN_POINT('Ctrl Pts',(3.81981808406148,138.247549018368,14.2080329938247));
#81490=CARTESIAN_POINT('Ctrl Pts',(3.8284904768729,138.144281287434,14.1131792843514));
#81491=CARTESIAN_POINT('Ctrl Pts',(3.83341021764234,138.090962193914,14.0531028302434));
#81492=CARTESIAN_POINT('Ctrl Pts',(3.83994036460814,138.031859088223,13.9710001760125));
#81493=CARTESIAN_POINT('Ctrl Pts',(3.84131392176737,138.020023168778,13.9535926738573));
#81494=CARTESIAN_POINT('Ctrl Pts',(3.84361348930118,138.001237309109,13.9243053624643));
#81495=CARTESIAN_POINT('Ctrl Pts',(3.84452935432236,137.994017579342,13.9126038202928));
#81496=CARTESIAN_POINT('Ctrl Pts',(3.84636554275031,137.980072700224,13.8890908497109));
#81497=CARTESIAN_POINT('Ctrl Pts',(3.84728555003971,137.97334387554,13.8772840732483));
#81498=CARTESIAN_POINT('Ctrl Pts',(3.84958915601224,137.957141519708,13.8476749462109));
#81499=CARTESIAN_POINT('Ctrl Pts',(3.8509812947885,137.94791839133,13.8297413122385));
#81500=CARTESIAN_POINT('Ctrl Pts',(3.8556364864431,137.918954180526,13.7696796720604));
#81501=CARTESIAN_POINT('Ctrl Pts',(3.85896366269804,137.901253914743,13.7266305527279));
#81502=CARTESIAN_POINT('Ctrl Pts',(3.86234166104071,137.886148208794,13.6826607501787));
#81503=CARTESIAN_POINT('Origin',(1.13913288526384,139.,13.3));
#81504=CARTESIAN_POINT('',(4.46223878927246,137.886148213663,13.6826607643511));
#81505=CARTESIAN_POINT('',(4.36393196101569,137.88614821266,13.6826607614313));
#81506=CARTESIAN_POINT('',(1.13913288526384,137.88614821265,13.6826607614027));
#81507=CARTESIAN_POINT('Ctrl Pts',(4.46223878927246,137.886148214676,13.6826607672995));
#81508=CARTESIAN_POINT('Ctrl Pts',(4.45883984757335,137.901538260174,13.7274582253084));
#81509=CARTESIAN_POINT('Ctrl Pts',(4.45537582733297,137.919617125364,13.7712873632294));
#81510=CARTESIAN_POINT('Ctrl Pts',(4.44726731267853,137.967797810042,13.8706389399772));
#81511=CARTESIAN_POINT('Ctrl Pts',(4.442622440193,137.999821846321,13.9250720199846));
#81512=CARTESIAN_POINT('Ctrl Pts',(4.43715156406992,138.044237488671,13.9883429697029));
#81513=CARTESIAN_POINT('Ctrl Pts',(4.43615335261791,138.052634187618,13.9998543310981));
#81514=CARTESIAN_POINT('Ctrl Pts',(4.43460660152402,138.066138494095,14.0176793164653));
#81515=CARTESIAN_POINT('Ctrl Pts',(4.43404949841628,138.071105742906,14.0240969427439));
#81516=CARTESIAN_POINT('Ctrl Pts',(4.43296938357515,138.080947272155,14.0365441229199));
#81517=CARTESIAN_POINT('Ctrl Pts',(4.43244605420597,138.085815451089,14.0425777921083));
#81518=CARTESIAN_POINT('Ctrl Pts',(4.4310916979544,138.098664698075,14.0581853851372));
#81519=CARTESIAN_POINT('Ctrl Pts',(4.43026699553161,138.106739069333,14.0676817996047));
#81520=CARTESIAN_POINT('Ctrl Pts',(4.42541626619723,138.155614040048,14.1233490357373));
#81521=CARTESIAN_POINT('Ctrl Pts',(4.42159405130105,138.19984090546,14.1663940138214));
#81522=CARTESIAN_POINT('Ctrl Pts',(4.41289925732351,138.307979880114,14.256264069738));
#81523=CARTESIAN_POINT('Ctrl Pts',(4.40804619480079,138.373638761826,14.3005013590557));
#81524=CARTESIAN_POINT('Ctrl Pts',(4.40158816018715,138.461814227166,14.3478053413701));
#81525=CARTESIAN_POINT('Ctrl Pts',(4.40021187739387,138.480664531222,14.3572750548741));
#81526=CARTESIAN_POINT('Ctrl Pts',(4.39791306533311,138.512158212797,14.3720508682451));
#81527=CARTESIAN_POINT('Ctrl Pts',(4.397000806824,138.524658479204,14.3776516530701));
#81528=CARTESIAN_POINT('Ctrl Pts',(4.39517630591881,138.549641960991,14.3883263304494));
#81529=CARTESIAN_POINT('Ctrl Pts',(4.39426444597717,138.56212021756,14.3934065276689));
#81530=CARTESIAN_POINT('Ctrl Pts',(4.39199083313674,138.593195146005,14.4054406324546));
#81531=CARTESIAN_POINT('Ctrl Pts',(4.39062089783546,138.61188511634,14.4121402495605));
#81532=CARTESIAN_POINT('Ctrl Pts',(4.38411576409656,138.700422223433,14.4413737525114));
#81533=CARTESIAN_POINT('Ctrl Pts',(4.37879027301252,138.77209714738,14.4578160350299));
#81534=CARTESIAN_POINT('Ctrl Pts',(4.36845327184661,138.911700192532,14.4763713952914));
#81535=CARTESIAN_POINT('Ctrl Pts',(4.3634732240909,138.979221341052,14.4794982430917));
#81536=CARTESIAN_POINT('Ctrl Pts',(4.35773579559411,139.060339039161,14.4762831904497));
#81537=CARTESIAN_POINT('Ctrl Pts',(4.35677651128038,139.074025502447,14.4755012588335));
#81538=CARTESIAN_POINT('Ctrl Pts',(4.35527589183683,139.095678275676,14.4738844932215));
#81539=CARTESIAN_POINT('Ctrl Pts',(4.35472676946382,139.103654653727,14.4732070823743));
#81540=CARTESIAN_POINT('Ctrl Pts',(4.35364899444119,139.119427482003,14.4717054188381));
#81541=CARTESIAN_POINT('Ctrl Pts',(4.35312021400177,139.127223777123,14.4708845500855));
#81542=CARTESIAN_POINT('Ctrl Pts',(4.35173194788079,139.147826140412,14.4685071227221));
#81543=CARTESIAN_POINT('Ctrl Pts',(4.3508794008774,139.160616256457,14.4668178588765));
#81544=CARTESIAN_POINT('Ctrl Pts',(4.34897470980326,139.189427692726,14.4625298076386));
#81545=CARTESIAN_POINT('Ctrl Pts',(4.34792800012487,139.205428428913,14.4598093021381));
#81546=CARTESIAN_POINT('Ctrl Pts',(4.34446323982024,139.258728114645,14.4496093571142));
#81547=CARTESIAN_POINT('Ctrl Pts',(4.34209412215202,139.295721751769,14.4406537229038));
#81548=CARTESIAN_POINT('Ctrl Pts',(4.33432497097638,139.416058457358,14.4052724124232));
#81549=CARTESIAN_POINT('Ctrl Pts',(4.32898282799453,139.496885753533,14.3713705178584));
#81550=CARTESIAN_POINT('Ctrl Pts',(4.32202694378543,139.590845735638,14.3190209005579));
#81551=CARTESIAN_POINT('Ctrl Pts',(4.32070800932295,139.608217705487,14.3087484440332));
#81552=CARTESIAN_POINT('Ctrl Pts',(4.31856728609634,139.635638199719,14.2915682042359));
#81553=CARTESIAN_POINT('Ctrl Pts',(4.31775579915853,139.645858684081,14.2849416053744));
#81554=CARTESIAN_POINT('Ctrl Pts',(4.31604025158083,139.66708876973,14.2707042419827));
#81555=CARTESIAN_POINT('Ctrl Pts',(4.31513508841991,139.67807503198,14.2630619800493));
#81556=CARTESIAN_POINT('Ctrl Pts',(4.31290459713402,139.704609389953,14.2439250336748));
#81557=CARTESIAN_POINT('Ctrl Pts',(4.31157177889594,139.720008745971,14.2322318327998));
#81558=CARTESIAN_POINT('Ctrl Pts',(4.30865214745907,139.752743788209,14.2060800796655));
#81559=CARTESIAN_POINT('Ctrl Pts',(4.30706072335657,139.769965467499,14.1914916637237));
#81560=CARTESIAN_POINT('Ctrl Pts',(4.30209177922903,139.821848796696,14.1449162480972));
#81561=CARTESIAN_POINT('Ctrl Pts',(4.29866046480935,139.85501434169,14.1113375841883));
#81562=CARTESIAN_POINT('Ctrl Pts',(4.2898472743371,139.934192371447,14.0209123679554));
#81563=CARTESIAN_POINT('Ctrl Pts',(4.28444103841335,139.977096104843,13.9616000841065));
#81564=CARTESIAN_POINT('Ctrl Pts',(4.27834744578894,140.020975857553,13.8872643767603));
#81565=CARTESIAN_POINT('Ctrl Pts',(4.27741968537076,140.027528112962,13.8757231663888));
#81566=CARTESIAN_POINT('Ctrl Pts',(4.27595651050231,140.03767482986,13.857125344645));
#81567=CARTESIAN_POINT('Ctrl Pts',(4.27541391759355,140.041395434055,13.8501393109333));
#81568=CARTESIAN_POINT('Ctrl Pts',(4.27433720048232,140.048699062977,13.836085915959));
#81569=CARTESIAN_POINT('Ctrl Pts',(4.2738031118734,140.052281762572,13.8290188421305));
#81570=CARTESIAN_POINT('Ctrl Pts',(4.27238275705343,140.061691326891,13.8099840660879));
#81571=CARTESIAN_POINT('Ctrl Pts',(4.27150402194782,140.067387270411,13.7979524808835));
#81572=CARTESIAN_POINT('Ctrl Pts',(4.26952918233838,140.079861508819,13.770404898972));
#81573=CARTESIAN_POINT('Ctrl Pts',(4.26843913697486,140.086511757881,13.7548339315658));
#81574=CARTESIAN_POINT('Ctrl Pts',(4.26474657679644,140.108115316652,13.7010703443708));
#81575=CARTESIAN_POINT('Ctrl Pts',(4.26220000385717,140.121409211381,13.6622413140163));
#81576=CARTESIAN_POINT('Ctrl Pts',(4.25462151029059,140.154985078119,13.5444277020347));
#81577=CARTESIAN_POINT('Ctrl Pts',(4.24962214760114,140.169123891407,13.4639612278263));
#81578=CARTESIAN_POINT('Ctrl Pts',(4.24301350762205,140.176309023071,13.3618673914798));
#81579=CARTESIAN_POINT('Ctrl Pts',(4.24165139255027,140.177220432482,13.3410177904647));
#81580=CARTESIAN_POINT('Ctrl Pts',(4.23936961470675,140.177811212067,13.3065025107405));
#81581=CARTESIAN_POINT('Ctrl Pts',(4.23845989866968,140.177807427122,13.2928465347871));
#81582=CARTESIAN_POINT('Ctrl Pts',(4.23663540983044,140.177327590376,13.2656887699477));
#81583=CARTESIAN_POINT('Ctrl Pts',(4.23572093635781,140.176856658747,13.2521889773352));
#81584=CARTESIAN_POINT('Ctrl Pts',(4.23343074134145,140.175110049721,13.218676651758));
#81585=CARTESIAN_POINT('Ctrl Pts',(4.23204656768424,140.173555291358,13.198683623914));
#81586=CARTESIAN_POINT('Ctrl Pts',(4.22899174975599,140.169049348557,13.1551514016407));
#81587=CARTESIAN_POINT('Ctrl Pts',(4.22731566280452,140.165895823589,13.1316423629123));
#81588=CARTESIAN_POINT('Ctrl Pts',(4.22192166952304,140.153602640877,13.0571453659457));
#81589=CARTESIAN_POINT('Ctrl Pts',(4.21813886193538,140.141809436159,13.0066609810062));
#81590=CARTESIAN_POINT('Ctrl Pts',(4.20962252947812,140.108043336665,12.8957023586665));
#81591=CARTESIAN_POINT('Ctrl Pts',(4.20489053403361,140.084360967074,12.8359103970641));
#81592=CARTESIAN_POINT('Ctrl Pts',(4.19935221576864,140.049684424948,12.7657192386257));
#81593=CARTESIAN_POINT('Ctrl Pts',(4.19836597707902,140.043221543054,12.7532073703155));
#81594=CARTESIAN_POINT('Ctrl Pts',(4.19683340086377,140.032698650515,12.7337016126807));
#81595=CARTESIAN_POINT('Ctrl Pts',(4.19627874147077,140.028788579058,12.7266288849215));
#81596=CARTESIAN_POINT('Ctrl Pts',(4.19519945239944,140.020973205864,12.7128294450961));
#81597=CARTESIAN_POINT('Ctrl Pts',(4.19467456224787,140.017073517697,12.7061001658846));
#81598=CARTESIAN_POINT('Ctrl Pts',(4.19331037065193,140.006686924027,12.6885795083732));
#81599=CARTESIAN_POINT('Ctrl Pts',(4.19247757065418,140.000092909207,12.6778522801052));
#81600=CARTESIAN_POINT('Ctrl Pts',(4.18763637439323,139.960354628201,12.6154705537781));
#81601=CARTESIAN_POINT('Ctrl Pts',(4.18382917001659,139.923381698074,12.5663586264395));
#81602=CARTESIAN_POINT('Ctrl Pts',(4.17514977927128,139.830466074514,12.4611568800536));
#81603=CARTESIAN_POINT('Ctrl Pts',(4.17029713669324,139.772372342863,12.4073795892837));
#81604=CARTESIAN_POINT('Ctrl Pts',(4.16383953751664,139.692499081472,12.3471175278124));
#81605=CARTESIAN_POINT('Ctrl Pts',(4.16246321877293,139.675323426076,12.3348688352704));
#81606=CARTESIAN_POINT('Ctrl Pts',(4.16016436345579,139.646467503178,12.3154379432019));
#81607=CARTESIAN_POINT('Ctrl Pts',(4.15925209846732,139.634973858544,12.3079864675178));
#81608=CARTESIAN_POINT('Ctrl Pts',(4.15742759730676,139.61192278093,12.2936068995195));
#81609=CARTESIAN_POINT('Ctrl Pts',(4.15651574379753,139.600371218434,12.2866733318614));
#81610=CARTESIAN_POINT('Ctrl Pts',(4.15424217192136,139.571509725801,12.2700166045455));
#81611=CARTESIAN_POINT('Ctrl Pts',(4.15287227181573,139.554068616706,12.2605304015603));
#81612=CARTESIAN_POINT('Ctrl Pts',(4.14649639509764,139.472710868938,12.2189093867736));
#81613=CARTESIAN_POINT('Ctrl Pts',(4.14131081953153,139.406198693131,12.1922039408861));
#81614=CARTESIAN_POINT('Ctrl Pts',(4.13096433975432,139.271110897189,12.1517738831739));
#81615=CARTESIAN_POINT('Ctrl Pts',(4.12582926277561,139.202898331166,12.137778860655));
#81616=CARTESIAN_POINT('Ctrl Pts',(4.11995675104902,139.120323250853,12.12833339702));
#81617=CARTESIAN_POINT('Ctrl Pts',(4.1190044122164,139.106774203128,12.1270210476052));
#81618=CARTESIAN_POINT('Ctrl Pts',(4.11751203662919,139.085244994571,12.1253119093653));
#81619=CARTESIAN_POINT('Ctrl Pts',(4.11696434831162,139.077278729014,12.1247609490538));
#81620=CARTESIAN_POINT('Ctrl Pts',(4.1158868775848,139.061464499495,12.1238287117657));
#81621=CARTESIAN_POINT('Ctrl Pts',(4.11535700252979,139.053617147161,12.1234448618862));
#81622=CARTESIAN_POINT('Ctrl Pts',(4.11396205697664,139.032790869798,12.1226349598366));
#81623=CARTESIAN_POINT('Ctrl Pts',(4.11310404754831,139.019807311156,12.1223449639349));
#81624=CARTESIAN_POINT('Ctrl Pts',(4.11118477871192,138.990448123899,12.1221749268985));
#81625=CARTESIAN_POINT('Ctrl Pts',(4.11012908063906,138.97407426414,12.1224215309074));
#81626=CARTESIAN_POINT('Ctrl Pts',(4.10661795418094,138.919095177664,12.1243969597955));
#81627=CARTESIAN_POINT('Ctrl Pts',(4.10421285225986,138.880569461679,12.1276839954234));
#81628=CARTESIAN_POINT('Ctrl Pts',(4.09648626112016,138.756913829389,12.1443947797012));
#81629=CARTESIAN_POINT('Ctrl Pts',(4.0912167546949,138.673086100112,12.1652576904566));
#81630=CARTESIAN_POINT('Ctrl Pts',(4.08433405569668,138.573203056165,12.2021142422659));
#81631=CARTESIAN_POINT('Ctrl Pts',(4.08300505710345,138.554307555417,12.2096482526637));
#81632=CARTESIAN_POINT('Ctrl Pts',(4.08085246850904,138.524399964962,12.2224803175672));
#81633=CARTESIAN_POINT('Ctrl Pts',(4.08003940761502,138.513258335464,12.2274672068139));
#81634=CARTESIAN_POINT('Ctrl Pts',(4.07832404442594,138.490090188883,12.238272402639));
#81635=CARTESIAN_POINT('Ctrl Pts',(4.07742069060003,138.47808119861,12.2441239439785));
#81636=CARTESIAN_POINT('Ctrl Pts',(4.07520204452629,138.449068280091,12.2588767616139));
#81637=CARTESIAN_POINT('Ctrl Pts',(4.07387945019642,138.432177912427,12.2679915897651));
#81638=CARTESIAN_POINT('Ctrl Pts',(4.06739663749784,138.351381900692,12.3141768591782));
#81639=CARTESIAN_POINT('Ctrl Pts',(4.0620409255153,138.290847261586,12.3567864633664));
#81640=CARTESIAN_POINT('Ctrl Pts',(4.05159333881989,138.182635933775,12.4492917819815));
#81641=CARTESIAN_POINT('Ctrl Pts',(4.04653348150186,138.13454146534,12.4982697631419));
#81642=CARTESIAN_POINT('Ctrl Pts',(4.0407255093698,138.082284346631,12.5617047430064));
#81643=CARTESIAN_POINT('Ctrl Pts',(4.0397689569501,138.073777007686,12.5724060776149));
#81644=CARTESIAN_POINT('Ctrl Pts',(4.03827157965962,138.060590830572,12.5895991105448));
#81645=CARTESIAN_POINT('Ctrl Pts',(4.03772302101481,138.055788767651,12.5959941977968));
#81646=CARTESIAN_POINT('Ctrl Pts',(4.03664537016418,138.046405152408,12.6087594598157));
#81647=CARTESIAN_POINT('Ctrl Pts',(4.03611616394323,138.041821411729,12.6151274439781));
#81648=CARTESIAN_POINT('Ctrl Pts',(4.03472529530285,138.029851273586,12.632112454111));
#81649=CARTESIAN_POINT('Ctrl Pts',(4.03387061919083,138.022575286856,12.642806505144));
#81650=CARTESIAN_POINT('Ctrl Pts',(4.0289660098986,137.981405004415,12.7055142484427));
#81651=CARTESIAN_POINT('Ctrl Pts',(4.0251195025581,137.951485670696,12.7600290313087));
#81652=CARTESIAN_POINT('Ctrl Pts',(4.01649748653914,137.894250419969,12.8872063188554));
#81653=CARTESIAN_POINT('Ctrl Pts',(4.01173855375662,137.869531004189,12.9607078250999));
#81654=CARTESIAN_POINT('Ctrl Pts',(4.00537865271191,137.847444882588,13.0567684620347));
#81655=CARTESIAN_POINT('Ctrl Pts',(4.00399506805886,137.843252005322,13.0775615444864));
#81656=CARTESIAN_POINT('Ctrl Pts',(4.00168746726154,137.837275326005,13.1119718177466));
#81657=CARTESIAN_POINT('Ctrl Pts',(4.00077389022519,137.835164120319,13.1255276198361));
#81658=CARTESIAN_POINT('Ctrl Pts',(3.9989493155907,137.831452273062,13.1524455747605));
#81659=CARTESIAN_POINT('Ctrl Pts',(3.99803874251361,137.82984290811,13.1658044236526));
#81660=CARTESIAN_POINT('Ctrl Pts',(3.99577333998866,137.826436475754,13.1988371011533));
#81661=CARTESIAN_POINT('Ctrl Pts',(3.99441046093843,137.82490493676,13.2185335185329));
#81662=CARTESIAN_POINT('Ctrl Pts',(3.9914118735987,137.82265130905,13.2614632296254));
#81663=CARTESIAN_POINT('Ctrl Pts',(3.98977107650809,137.822120233597,13.2846978653725));
#81664=CARTESIAN_POINT('Ctrl Pts',(3.98455776885865,137.822612178877,13.3577431471365));
#81665=CARTESIAN_POINT('Ctrl Pts',(3.9809252128372,137.826107399488,13.4074789277716));
#81666=CARTESIAN_POINT('Ctrl Pts',(3.97227842026258,137.841796571579,13.5242435099982));
#81667=CARTESIAN_POINT('Ctrl Pts',(3.96725672351583,137.856675228393,13.5907406938577));
#81668=CARTESIAN_POINT('Ctrl Pts',(3.96177807351904,137.88008103812,13.6646462785259));
#81669=CARTESIAN_POINT('Ctrl Pts',(3.96111095830634,137.883060131196,13.6736719509654));
#81670=CARTESIAN_POINT('Ctrl Pts',(3.96044919307343,137.886148212676,13.6826607614778));
#81671=CARTESIAN_POINT('Ctrl Pts',(3.86234166104071,137.886148208794,13.6826607501787));
#81672=CARTESIAN_POINT('Ctrl Pts',(3.863044184664,137.883006669279,13.6735163333174));
#81673=CARTESIAN_POINT('Ctrl Pts',(3.86374880232695,137.87997734707,13.6643320879671));
#81674=CARTESIAN_POINT('Ctrl Pts',(3.87062727730392,137.851575758721,13.5745197877842));
#81675=CARTESIAN_POINT('Ctrl Pts',(3.87692097289799,137.834839327831,13.4914185579036));
#81676=CARTESIAN_POINT('Ctrl Pts',(3.8838435464494,137.825914792403,13.3938124442637));
#81677=CARTESIAN_POINT('Ctrl Pts',(3.88478660732029,137.824917709719,13.3803647899413));
#81678=CARTESIAN_POINT('Ctrl Pts',(3.88627007993735,137.823697883064,13.3589255944686));
#81679=CARTESIAN_POINT('Ctrl Pts',(3.88681793719884,137.82332519609,13.3509441980889));
#81680=CARTESIAN_POINT('Ctrl Pts',(3.88790206571254,137.822743603264,13.3350101729448));
#81681=CARTESIAN_POINT('Ctrl Pts',(3.88843834175249,137.822533987937,13.3270579966016));
#81682=CARTESIAN_POINT('Ctrl Pts',(3.88986105329992,137.822189017246,13.3057935938219));
#81683=CARTESIAN_POINT('Ctrl Pts',(3.89073998378341,137.822198760501,13.2924797543214));
#81684=CARTESIAN_POINT('Ctrl Pts',(3.89540832308217,137.823463100492,13.2210098048795));
#81685=CARTESIAN_POINT('Ctrl Pts',(3.89902262471667,137.828799245817,13.1630003930873));
#81686=CARTESIAN_POINT('Ctrl Pts',(3.90764572898961,137.851806010317,13.0255159015268));
#81687=CARTESIAN_POINT('Ctrl Pts',(3.91262902588312,137.873457832592,12.9470237483517));
#81688=CARTESIAN_POINT('Ctrl Pts',(3.91922440940153,137.910633308223,12.8518772809854));
#81689=CARTESIAN_POINT('Ctrl Pts',(3.92059153722713,137.918774431264,12.8325762704663));
#81690=CARTESIAN_POINT('Ctrl Pts',(3.92288338263702,137.933097014266,12.8009993982069));
#81691=CARTESIAN_POINT('Ctrl Pts',(3.92379810211894,137.938986608803,12.788595914807));
#81692=CARTESIAN_POINT('Ctrl Pts',(3.92563433408657,137.951141418996,12.7641120885698));
#81693=CARTESIAN_POINT('Ctrl Pts',(3.92655556892097,137.957401834685,12.7520317388586));
#81694=CARTESIAN_POINT('Ctrl Pts',(3.92886694038054,137.973500777671,12.7222416038312));
#81695=CARTESIAN_POINT('Ctrl Pts',(3.93026574486999,137.983589286966,12.7046727021241));
#81696=CARTESIAN_POINT('Ctrl Pts',(3.93647404406036,138.02983654806,12.6287390669985));
#81697=CARTESIAN_POINT('Ctrl Pts',(3.94144587200666,138.070600854173,12.5733481309762));
#81698=CARTESIAN_POINT('Ctrl Pts',(3.95175854232748,138.163506789647,12.4678011336225));
#81699=CARTESIAN_POINT('Ctrl Pts',(3.9570835177498,138.215920007638,12.4182427606383));
#81700=CARTESIAN_POINT('Ctrl Pts',(3.96311442826415,138.28308441392,12.3654909836635));
#81701=CARTESIAN_POINT('Ctrl Pts',(3.96405268996194,138.293776834541,12.3573845226047));
#81702=CARTESIAN_POINT('Ctrl Pts',(3.965530460591,138.311043161827,12.3447528319018));
#81703=CARTESIAN_POINT('Ctrl Pts',(3.96607732259554,138.317528237061,12.3401088711434));
#81704=CARTESIAN_POINT('Ctrl Pts',(3.96716133334605,138.330585207647,12.3309580061969));
#81705=CARTESIAN_POINT('Ctrl Pts',(3.96769846150726,138.33715666421,12.3264511972035));
#81706=CARTESIAN_POINT('Ctrl Pts',(3.96912629279859,138.354882192617,12.3145574407366));
#81707=CARTESIAN_POINT('Ctrl Pts',(3.9700093949864,138.366117570292,12.3072930312282));
#81708=CARTESIAN_POINT('Ctrl Pts',(3.97478027087287,138.428142352453,12.2686725000216));
#81709=CARTESIAN_POINT('Ctrl Pts',(3.97848364990891,138.481141040819,12.2410171718372));
#81710=CARTESIAN_POINT('Ctrl Pts',(3.98707301726176,138.608805655808,12.1862970875214));
#81711=CARTESIAN_POINT('Ctrl Pts',(3.99193861258386,138.684551617322,12.1625211813024));
#81712=CARTESIAN_POINT('Ctrl Pts',(3.99841287816808,138.782798876687,12.1422586217277));
#81713=CARTESIAN_POINT('Ctrl Pts',(3.99979144442897,138.803600695929,12.1385489028142));
#81714=CARTESIAN_POINT('Ctrl Pts',(4.00209703201997,138.838100074831,12.1333497024605));
#81715=CARTESIAN_POINT('Ctrl Pts',(4.00301379278357,138.851744506969,12.1315374271211));
#81716=CARTESIAN_POINT('Ctrl Pts',(4.00484997318898,138.878904672416,12.1284133383298));
#81717=CARTESIAN_POINT('Ctrl Pts',(4.00576904704223,138.892417553609,12.1270953258911));
#81718=CARTESIAN_POINT('Ctrl Pts',(4.00806673190948,138.925978746086,12.1244066804823));
#81719=CARTESIAN_POINT('Ctrl Pts',(4.00945378589659,138.946044402116,12.1233150354261));
#81720=CARTESIAN_POINT('Ctrl Pts',(4.01590713115923,139.038458687569,12.1206560395116));
#81721=CARTESIAN_POINT('Ctrl Pts',(4.02115697858442,139.110816955669,12.1252456511503));
#81722=CARTESIAN_POINT('Ctrl Pts',(4.03146088357986,139.249519309731,12.1469750639376));
#81723=CARTESIAN_POINT('Ctrl Pts',(4.03648604885995,139.315718338391,12.1633163723464));
#81724=CARTESIAN_POINT('Ctrl Pts',(4.04226631500642,139.393128952584,12.1897148811974));
#81725=CARTESIAN_POINT('Ctrl Pts',(4.04322679105769,139.406040985135,12.1943715914929));
#81726=CARTESIAN_POINT('Ctrl Pts',(4.04473094170385,139.426382976811,12.2021123695186));
#81727=CARTESIAN_POINT('Ctrl Pts',(4.04528240065399,139.433867420922,12.2050485112206));
#81728=CARTESIAN_POINT('Ctrl Pts',(4.04636712325934,139.448653627604,12.2110245517681));
#81729=CARTESIAN_POINT('Ctrl Pts',(4.04690048201913,139.455955956674,12.2140617984208));
#81730=CARTESIAN_POINT('Ctrl Pts',(4.04830553178762,139.475258833131,12.2223194574133));
#81731=CARTESIAN_POINT('Ctrl Pts',(4.04917004630636,139.487204309322,12.2276668863286));
#81732=CARTESIAN_POINT('Ctrl Pts',(4.05110498771915,139.514021677953,12.240212444166));
#81733=CARTESIAN_POINT('Ctrl Pts',(4.0521697442321,139.528836410017,12.24752669628));
#81734=CARTESIAN_POINT('Ctrl Pts',(4.05572143299817,139.578225222409,12.2732169789663));
#81735=CARTESIAN_POINT('Ctrl Pts',(4.05815692151328,139.612037170705,12.2930051339613));
#81736=CARTESIAN_POINT('Ctrl Pts',(4.06584296724123,139.715931877936,12.3609783543525));
#81737=CARTESIAN_POINT('Ctrl Pts',(4.07104648270154,139.781807688376,12.4150732538963));
#81738=CARTESIAN_POINT('Ctrl Pts',(4.07786568259445,139.855653334548,12.4904483478774));
#81739=CARTESIAN_POINT('Ctrl Pts',(4.07920668689932,139.86963343173,12.505484979092));
#81740=CARTESIAN_POINT('Ctrl Pts',(4.08146721712582,139.892245704048,12.5311182722933));
#81741=CARTESIAN_POINT('Ctrl Pts',(4.08237733608271,139.901099516073,12.5415139136248));
#81742=CARTESIAN_POINT('Ctrl Pts',(4.08421415692083,139.91845665087,12.5626265990101));
#81743=CARTESIAN_POINT('Ctrl Pts',(4.08514074215499,139.926957956123,12.5733425345301));
#81744=CARTESIAN_POINT('Ctrl Pts',(4.08748571731678,139.947826438644,12.6006096138682));
#81745=CARTESIAN_POINT('Ctrl Pts',(4.08891333341489,139.959947883799,12.6173420794325));
#81746=CARTESIAN_POINT('Ctrl Pts',(4.0920807929871,139.985560860128,12.6547302026406));
#81747=CARTESIAN_POINT('Ctrl Pts',(4.09382677070315,139.998855882451,12.6755081253717));
#81748=CARTESIAN_POINT('Ctrl Pts',(4.09958412488075,140.04006275325,12.7445937437427));
#81749=CARTESIAN_POINT('Ctrl Pts',(4.10367059351438,140.065195490999,12.7944663958533));
#81750=CARTESIAN_POINT('Ctrl Pts',(4.11195730571419,140.1086890359,12.8985562526817));
#81751=CARTESIAN_POINT('Ctrl Pts',(4.11614694660291,140.126829313793,12.9527174174099));
#81752=CARTESIAN_POINT('Ctrl Pts',(4.12122732478859,140.144610884334,13.0221940472427));
#81753=CARTESIAN_POINT('Ctrl Pts',(4.12225596707458,140.147982242468,13.0364719296508));
#81754=CARTESIAN_POINT('Ctrl Pts',(4.12384081880359,140.152827789133,13.0588550045718));
#81755=CARTESIAN_POINT('Ctrl Pts',(4.12440619028848,140.154485099265,13.066918499123));
#81756=CARTESIAN_POINT('Ctrl Pts',(4.12549530239638,140.157540678443,13.0826181014993));
#81757=CARTESIAN_POINT('Ctrl Pts',(4.1260194683181,140.158948231242,13.0902517844252));
#81758=CARTESIAN_POINT('Ctrl Pts',(4.12736690079609,140.162398491818,13.1100600443844));
#81759=CARTESIAN_POINT('Ctrl Pts',(4.12818403990934,140.164325520632,13.1222542469693));
#81760=CARTESIAN_POINT('Ctrl Pts',(4.13305057899264,140.174765558045,13.1958012608342));
#81761=CARTESIAN_POINT('Ctrl Pts',(4.1368928406087,140.178620466317,13.257724628146));
#81762=CARTESIAN_POINT('Ctrl Pts',(4.14560146851328,140.176268320244,13.3985379795315));
#81763=CARTESIAN_POINT('Ctrl Pts',(4.15044849390026,140.167031755995,13.4770658970451));
#81764=CARTESIAN_POINT('Ctrl Pts',(4.15690352262628,140.145453726776,13.5747330931787));
#81765=CARTESIAN_POINT('Ctrl Pts',(4.15828370065542,140.140334965799,13.5952602056001));
#81766=CARTESIAN_POINT('Ctrl Pts',(4.16059122597909,140.1309765661,13.6289021736007));
#81767=CARTESIAN_POINT('Ctrl Pts',(4.16150827554353,140.127054431181,13.6421007379544));
#81768=CARTESIAN_POINT('Ctrl Pts',(4.16334445807152,140.118808279858,13.668167500933));
#81769=CARTESIAN_POINT('Ctrl Pts',(4.16426323575358,140.114491376416,13.681035721279));
#81770=CARTESIAN_POINT('Ctrl Pts',(4.16655903885429,140.103241826412,13.7127412809699));
#81771=CARTESIAN_POINT('Ctrl Pts',(4.16794447643526,140.096048407646,13.7314808158143));
#81772=CARTESIAN_POINT('Ctrl Pts',(4.17099985047535,140.079321879548,13.7719335935678));
#81773=CARTESIAN_POINT('Ctrl Pts',(4.17267518388653,140.069604863876,13.7935608790472));
#81774=CARTESIAN_POINT('Ctrl Pts',(4.1780547896094,140.036683170128,13.8612895158023));
#81775=CARTESIAN_POINT('Ctrl Pts',(4.18182339601313,140.011099937413,13.9061633292076));
#81776=CARTESIAN_POINT('Ctrl Pts',(4.19035047334182,139.947084298549,14.0030586809752));
#81777=CARTESIAN_POINT('Ctrl Pts',(4.19510806201368,139.907140701683,14.0538946776807));
#81778=CARTESIAN_POINT('Ctrl Pts',(4.20066676073147,139.853677786797,14.1114964363587));
#81779=CARTESIAN_POINT('Ctrl Pts',(4.20165013783448,139.843941659251,14.1216171548754));
#81780=CARTESIAN_POINT('Ctrl Pts',(4.20318144533018,139.828304239512,14.1373009186825));
#81781=CARTESIAN_POINT('Ctrl Pts',(4.20373761376925,139.822522842852,14.1429809751423));
#81782=CARTESIAN_POINT('Ctrl Pts',(4.20482347704923,139.811024340808,14.1540469892431));
#81783=CARTESIAN_POINT('Ctrl Pts',(4.20535338184087,139.805311151524,14.1594362668702));
#81784=CARTESIAN_POINT('Ctrl Pts',(4.20673719494012,139.790135862876,14.1734669826889));
#81785=CARTESIAN_POINT('Ctrl Pts',(4.20758431720912,139.78058558091,14.182012151804));
#81786=CARTESIAN_POINT('Ctrl Pts',(4.20947287529198,139.758757792836,14.2009103757974));
#81787=CARTESIAN_POINT('Ctrl Pts',(4.21050904345583,139.746404046763,14.2111717419622));
#81788=CARTESIAN_POINT('Ctrl Pts',(4.2139136676338,139.704715992399,14.2443819634546));
#81789=CARTESIAN_POINT('Ctrl Pts',(4.21623507960074,139.674502187942,14.2661930787221));
#81790=CARTESIAN_POINT('Ctrl Pts',(4.22405775170889,139.568755265612,14.335148844342));
#81791=CARTESIAN_POINT('Ctrl Pts',(4.22949294553982,139.488944500588,14.3751499681993));
#81792=CARTESIAN_POINT('Ctrl Pts',(4.23654555759565,139.386600936416,14.412670383838));
#81793=CARTESIAN_POINT('Ctrl Pts',(4.23785427001054,139.367637298898,14.4190792674328));
#81794=CARTESIAN_POINT('Ctrl Pts',(4.23998668599268,139.33685795315,14.4286145707674));
#81795=CARTESIAN_POINT('Ctrl Pts',(4.24080036841133,139.325140370329,14.4320458694704));
#81796=CARTESIAN_POINT('Ctrl Pts',(4.24252755420066,139.300341246337,14.4388910983532));
#81797=CARTESIAN_POINT('Ctrl Pts',(4.24344227492753,139.287250105735,14.442263169512));
#81798=CARTESIAN_POINT('Ctrl Pts',(4.24571213738936,139.254887704861,14.4500077152275));
#81799=CARTESIAN_POINT('Ctrl Pts',(4.24707526915934,139.235559524803,14.4541217938672));
#81800=CARTESIAN_POINT('Ctrl Pts',(4.25007177527111,139.193326942467,14.4620061251788));
#81801=CARTESIAN_POINT('Ctrl Pts',(4.25171017753887,139.170396420552,14.4655893267413));
#81802=CARTESIAN_POINT('Ctrl Pts',(4.25690135201986,139.098224813765,14.4746919794484));
#81803=CARTESIAN_POINT('Ctrl Pts',(4.2605134260896,139.048735289351,14.4777832766728));
#81804=CARTESIAN_POINT('Ctrl Pts',(4.26916697635402,138.930821355767,14.4777034180323));
#81805=CARTESIAN_POINT('Ctrl Pts',(4.27421714700351,138.862569582109,14.4717018650513));
#81806=CARTESIAN_POINT('Ctrl Pts',(4.28001937562035,138.781718469343,14.4574265510309));
#81807=CARTESIAN_POINT('Ctrl Pts',(4.28097887678128,138.768258454996,14.4548068863584));
#81808=CARTESIAN_POINT('Ctrl Pts',(4.28248187046343,138.746986105409,14.4502797992677));
#81809=CARTESIAN_POINT('Ctrl Pts',(4.28303312823117,138.739142691218,14.4485265001495));
#81810=CARTESIAN_POINT('Ctrl Pts',(4.28411781100202,138.723615338628,14.4448882751248));
#81811=CARTESIAN_POINT('Ctrl Pts',(4.28465132612426,138.715931269189,14.4430059525042));
#81812=CARTESIAN_POINT('Ctrl Pts',(4.28605732832364,138.695576341321,14.437801769148));
#81813=CARTESIAN_POINT('Ctrl Pts',(4.28692262128515,138.682940520705,14.4343456051301));
#81814=CARTESIAN_POINT('Ctrl Pts',(4.2888596454158,138.654485328609,14.4260498427597));
#81815=CARTESIAN_POINT('Ctrl Pts',(4.28992568776206,138.638704781494,14.4210862841359));
#81816=CARTESIAN_POINT('Ctrl Pts',(4.29348409797901,138.585859886533,14.4032328019405));
#81817=CARTESIAN_POINT('Ctrl Pts',(4.29592481694604,138.549334961245,14.38882324173));
#81818=CARTESIAN_POINT('Ctrl Pts',(4.30360507289333,138.43634369359,14.3375845565311));
#81819=CARTESIAN_POINT('Ctrl Pts',(4.30879834105075,138.363109819112,14.2943136048585));
#81820=CARTESIAN_POINT('Ctrl Pts',(4.3156071833194,138.278696391242,14.2312563983944));
#81821=CARTESIAN_POINT('Ctrl Pts',(4.31694951655112,138.262558123966,14.218529679677));
#81822=CARTESIAN_POINT('Ctrl Pts',(4.31921163723704,138.236262045307,14.1966526354109));
#81823=CARTESIAN_POINT('Ctrl Pts',(4.32012198792993,138.225915443102,14.1877357063215));
#81824=CARTESIAN_POINT('Ctrl Pts',(4.32195876188461,138.205525209974,14.1695354239991));
#81825=CARTESIAN_POINT('Ctrl Pts',(4.32288506011634,138.195483563498,14.1602530566789));
#81826=CARTESIAN_POINT('Ctrl Pts',(4.32522824159195,138.170697503094,14.1365275567089));
#81827=CARTESIAN_POINT('Ctrl Pts',(4.32665432097801,138.156167400717,14.1218682590884));
#81828=CARTESIAN_POINT('Ctrl Pts',(4.32981767871815,138.125159018708,14.0888947001723));
#81829=CARTESIAN_POINT('Ctrl Pts',(4.33156106352158,138.108855347333,14.0704301746894));
#81830=CARTESIAN_POINT('Ctrl Pts',(4.33730411268014,138.057653330605,14.0086407010644));
#81831=CARTESIAN_POINT('Ctrl Pts',(4.34137844510893,138.025244732418,13.9633551692109));
#81832=CARTESIAN_POINT('Ctrl Pts',(4.34967225567738,137.966194692202,13.867119329472));
#81833=CARTESIAN_POINT('Ctrl Pts',(4.35388127828011,137.939831059775,13.8161594791115));
#81834=CARTESIAN_POINT('Ctrl Pts',(4.35897900498236,137.911511664804,13.7500034285213));
#81835=CARTESIAN_POINT('Ctrl Pts',(4.36000695149036,137.905994771712,13.7364201540833));
#81836=CARTESIAN_POINT('Ctrl Pts',(4.36159098162245,137.897778735615,13.7150555054399));
#81837=CARTESIAN_POINT('Ctrl Pts',(4.36215621281117,137.89490532634,13.7073432959549));
#81838=CARTESIAN_POINT('Ctrl Pts',(4.36312428911873,137.89008165393,13.693969755074));
#81839=CARTESIAN_POINT('Ctrl Pts',(4.36352933703883,137.888093373265,13.6883227493715));
#81840=CARTESIAN_POINT('Ctrl Pts',(4.36393196101569,137.88614821267,13.68266076146));
#81841=CARTESIAN_POINT('Origin',(1.13913288526384,139.,13.3));
#81842=CARTESIAN_POINT('',(4.96216798774592,137.886148228644,13.6826608079585));
#81843=CARTESIAN_POINT('',(4.86231567683355,137.88614821265,13.6826607614027));
#81844=CARTESIAN_POINT('',(1.13913288526384,137.88614821265,13.6826607614027));
#81845=CARTESIAN_POINT('Ctrl Pts',(4.96216799084082,137.886148228708,13.6826608081431));
#81846=CARTESIAN_POINT('Ctrl Pts',(4.9613252995471,137.89048591061,13.6952869631277));
#81847=CARTESIAN_POINT('Ctrl Pts',(4.96047762550991,137.8950399563,13.7078442468175));
#81848=CARTESIAN_POINT('Ctrl Pts',(4.95792916134544,137.909276554256,13.7451080279077));
#81849=CARTESIAN_POINT('Ctrl Pts',(4.95621286131286,137.919578019688,13.7695604010044));
#81850=CARTESIAN_POINT('Ctrl Pts',(4.95350210532465,137.936863001935,13.807002265906));
#81851=CARTESIAN_POINT('Ctrl Pts',(4.95252681100481,137.943279953068,13.8202444465315));
#81852=CARTESIAN_POINT('Ctrl Pts',(4.95067059480853,137.955850200518,13.8449921117628));
#81853=CARTESIAN_POINT('Ctrl Pts',(4.94979165683997,137.961949909538,13.8565224089485));
#81854=CARTESIAN_POINT('Ctrl Pts',(4.94777226926544,137.976289436622,13.8825722215191));
#81855=CARTESIAN_POINT('Ctrl Pts',(4.94662768265399,137.984648825597,13.8970223224393));
#81856=CARTESIAN_POINT('Ctrl Pts',(4.94291149710467,138.012511706058,13.9429076759284));
#81857=CARTESIAN_POINT('Ctrl Pts',(4.9402986399165,138.033188292644,13.973600797449));
#81858=CARTESIAN_POINT('Ctrl Pts',(4.93627484675891,138.066660717844,14.0185656259162));
#81859=CARTESIAN_POINT('Ctrl Pts',(4.93489550304426,138.078418169034,14.0335841144089));
#81860=CARTESIAN_POINT('Ctrl Pts',(4.92866410203643,138.132853176199,14.0997421921198));
#81861=CARTESIAN_POINT('Ctrl Pts',(4.92372821192867,138.179456688207,14.1474901430497));
#81862=CARTESIAN_POINT('Ctrl Pts',(4.91732836829574,138.246143999636,14.205129992097));
#81863=CARTESIAN_POINT('Ctrl Pts',(4.91577667980507,138.262827191691,14.2187684830071));
#81864=CARTESIAN_POINT('Ctrl Pts',(4.91311936018036,138.292427893299,14.2416413313572));
#81865=CARTESIAN_POINT('Ctrl Pts',(4.91200430023662,138.305175196318,14.2510863440971));
#81866=CARTESIAN_POINT('Ctrl Pts',(4.9103199526921,138.324989139761,14.2651562472053));
#81867=CARTESIAN_POINT('Ctrl Pts',(4.90973960676602,138.331920707704,14.269967171942));
#81868=CARTESIAN_POINT('Ctrl Pts',(4.90864787105764,138.345171151997,14.2789543374092));
#81869=CARTESIAN_POINT('Ctrl Pts',(4.90813565327589,138.351479523497,14.283144755104));
#81870=CARTESIAN_POINT('Ctrl Pts',(4.90685641495799,138.367454352868,14.2935355747707));
#81871=CARTESIAN_POINT('Ctrl Pts',(4.90609439039589,138.377172187341,14.2996561782074));
#81872=CARTESIAN_POINT('Ctrl Pts',(4.90265881191537,138.421819303103,14.3268724874282));
#81873=CARTESIAN_POINT('Ctrl Pts',(4.90007373103673,138.457744163936,14.3462883582678));
#81874=CARTESIAN_POINT('Ctrl Pts',(4.89321998972087,138.556833765062,14.3933639494403));
#81875=CARTESIAN_POINT('Ctrl Pts',(4.88902376597599,138.621533098448,14.4174095427146));
#81876=CARTESIAN_POINT('Ctrl Pts',(4.88211734985537,138.727804245728,14.446608742687));
#81877=CARTESIAN_POINT('Ctrl Pts',(4.87949152513504,138.768189360058,14.4554503232474));
#81878=CARTESIAN_POINT('Ctrl Pts',(4.87568232269473,138.825895553563,14.4649367022087));
#81879=CARTESIAN_POINT('Ctrl Pts',(4.87455338219,138.842896466133,14.4673509789729));
#81880=CARTESIAN_POINT('Ctrl Pts',(4.87254245815222,138.872951369964,14.4709506150809));
#81881=CARTESIAN_POINT('Ctrl Pts',(4.87166549338506,138.885983972806,14.4722913542373));
#81882=CARTESIAN_POINT('Ctrl Pts',(4.86980605784833,138.913442240746,14.4746539486601));
#81883=CARTESIAN_POINT('Ctrl Pts',(4.86882224137559,138.927869704442,14.4756280588304));
#81884=CARTESIAN_POINT('Ctrl Pts',(4.86610451712464,138.967428420489,14.4775680709763));
#81885=CARTESIAN_POINT('Ctrl Pts',(4.86435434618052,138.992577150795,14.4779949933377));
#81886=CARTESIAN_POINT('Ctrl Pts',(4.85927096061618,139.064659954666,14.4769104184862));
#81887=CARTESIAN_POINT('Ctrl Pts',(4.85588360827625,139.111512114175,14.4733981652422));
#81888=CARTESIAN_POINT('Ctrl Pts',(4.84632440991366,139.241212121811,14.4558367887005));
#81889=CARTESIAN_POINT('Ctrl Pts',(4.84007526894427,139.322958176544,14.4357117140014));
#81890=CARTESIAN_POINT('Ctrl Pts',(4.83318649233745,139.414616168242,14.4024392536724));
#81891=CARTESIAN_POINT('Ctrl Pts',(4.83223797125018,139.427280092607,14.3975931108697));
#81892=CARTESIAN_POINT('Ctrl Pts',(4.83075012865868,139.447255080425,14.3895510720333));
#81893=CARTESIAN_POINT('Ctrl Pts',(4.83020322980795,139.454621835428,14.3864978792897));
#81894=CARTESIAN_POINT('Ctrl Pts',(4.8291259101538,139.469193014806,14.3802846165405));
#81895=CARTESIAN_POINT('Ctrl Pts',(4.82859541619746,139.476397882888,14.3771267348045));
#81896=CARTESIAN_POINT('Ctrl Pts',(4.82719670964036,139.495454913528,14.3685454414609));
#81897=CARTESIAN_POINT('Ctrl Pts',(4.82633562724428,139.507249995601,14.3629968996757));
#81898=CARTESIAN_POINT('Ctrl Pts',(4.82440814501577,139.53372266143,14.3500028343377));
#81899=CARTESIAN_POINT('Ctrl Pts',(4.82334737870692,139.54834136322,14.3424431087491));
#81900=CARTESIAN_POINT('Ctrl Pts',(4.81980990964581,139.597041397762,14.3159509259341));
#81901=CARTESIAN_POINT('Ctrl Pts',(4.8173843326595,139.630341466459,14.2956328269391));
#81902=CARTESIAN_POINT('Ctrl Pts',(4.80968108270087,139.733207006002,14.2256358049688));
#81903=CARTESIAN_POINT('Ctrl Pts',(4.80445221475622,139.798393634498,14.1700346312013));
#81904=CARTESIAN_POINT('Ctrl Pts',(4.79761052412415,139.871002775977,14.0930110123185));
#81905=CARTESIAN_POINT('Ctrl Pts',(4.79627607992906,139.884624445623,14.077786481273));
#81906=CARTESIAN_POINT('Ctrl Pts',(4.79402749124873,139.906628177206,14.0518674686578));
#81907=CARTESIAN_POINT('Ctrl Pts',(4.79312267046347,139.915233716945,14.0413680323928));
#81908=CARTESIAN_POINT('Ctrl Pts',(4.79129765868563,139.932083064938,14.0200699435258));
#81909=CARTESIAN_POINT('Ctrl Pts',(4.790377598455,139.940325325732,14.0092727390762));
#81910=CARTESIAN_POINT('Ctrl Pts',(4.78805230267445,139.960517041506,13.9818512694132));
#81911=CARTESIAN_POINT('Ctrl Pts',(4.78663803717632,139.972222797628,13.9650540436754));
#81912=CARTESIAN_POINT('Ctrl Pts',(4.78097552468065,140.016812226229,13.8973756040288));
#81913=CARTESIAN_POINT('Ctrl Pts',(4.77660621608246,140.04618308808,13.8443011909821));
#81914=CARTESIAN_POINT('Ctrl Pts',(4.76682337943164,140.101715711064,13.7226884379973));
#81915=CARTESIAN_POINT('Ctrl Pts',(4.76139931737264,140.12583128198,13.6534795450859));
#81916=CARTESIAN_POINT('Ctrl Pts',(4.75496914222423,140.147484467288,13.5658352417451));
#81917=CARTESIAN_POINT('Ctrl Pts',(4.75376120304258,140.151232750708,13.5491028030434));
#81918=CARTESIAN_POINT('Ctrl Pts',(4.75196854485953,140.156326798652,13.5237828407258));
#81919=CARTESIAN_POINT('Ctrl Pts',(4.75137061678066,140.157944945356,13.5152532007076));
#81920=CARTESIAN_POINT('Ctrl Pts',(4.75026676002308,140.160782935531,13.4993341715396));
#81921=CARTESIAN_POINT('Ctrl Pts',(4.74975966750834,140.162026783495,13.4919502356081));
#81922=CARTESIAN_POINT('Ctrl Pts',(4.74852142361377,140.164913631506,13.4737551502107));
#81923=CARTESIAN_POINT('Ctrl Pts',(4.74779457164697,140.166476647137,13.4629321162488));
#81924=CARTESIAN_POINT('Ctrl Pts',(4.74485017356674,140.172251567791,13.4185864259944));
#81925=CARTESIAN_POINT('Ctrl Pts',(4.74269258476664,140.175171213505,13.384908955409));
#81926=CARTESIAN_POINT('Ctrl Pts',(4.73554572198398,140.180105707555,13.2713964457361));
#81927=CARTESIAN_POINT('Ctrl Pts',(4.73070949697103,140.175455430474,13.1914965531398));
#81928=CARTESIAN_POINT('Ctrl Pts',(4.72321844326576,140.15647967358,13.0737081938852));
#81929=CARTESIAN_POINT('Ctrl Pts',(4.72070459667175,140.148246756207,13.035080877252));
#81930=CARTESIAN_POINT('Ctrl Pts',(4.71703321833284,140.133757077295,12.9806669095727));
#81931=CARTESIAN_POINT('Ctrl Pts',(4.71592490155441,140.1290747447,12.964487099358));
#81932=CARTESIAN_POINT('Ctrl Pts',(4.71393715717662,140.120148383291,12.9359488486083));
#81933=CARTESIAN_POINT('Ctrl Pts',(4.7130623511339,140.116042556198,12.9235499625691));
#81934=CARTESIAN_POINT('Ctrl Pts',(4.71119308973944,140.106902386145,12.8974131340711));
#81935=CARTESIAN_POINT('Ctrl Pts',(4.71019705197139,140.101816572499,12.8836956835069));
#81936=CARTESIAN_POINT('Ctrl Pts',(4.70740270616179,140.086962644944,12.8458121831326));
#81937=CARTESIAN_POINT('Ctrl Pts',(4.70558653630758,140.07664638402,12.8218716244175));
#81938=CARTESIAN_POINT('Ctrl Pts',(4.69702201018986,140.024987822691,12.712156798395));
#81939=CARTESIAN_POINT('Ctrl Pts',(4.68996517977603,139.974138513674,12.6312633341923));
#81940=CARTESIAN_POINT('Ctrl Pts',(4.68244742533774,139.909202371822,12.5513298344739));
#81941=CARTESIAN_POINT('Ctrl Pts',(4.68187890052142,139.904221332689,12.5453214232013));
#81942=CARTESIAN_POINT('Ctrl Pts',(4.6790217057882,139.878820360923,12.5152938740889));
#81943=CARTESIAN_POINT('Ctrl Pts',(4.67675761584631,139.857499753496,12.4920498436192));
#81944=CARTESIAN_POINT('Ctrl Pts',(4.67377944302391,139.827546088066,12.461917322213));
#81945=CARTESIAN_POINT('Ctrl Pts',(4.67301813342315,139.819713506166,12.454254829944));
#81946=CARTESIAN_POINT('Ctrl Pts',(4.67174970788768,139.806347543848,12.441539276432));
#81947=CARTESIAN_POINT('Ctrl Pts',(4.67123843646845,139.800870977784,12.4364278459563));
#81948=CARTESIAN_POINT('Ctrl Pts',(4.67014415123697,139.78895099407,12.4255135426399));
#81949=CARTESIAN_POINT('Ctrl Pts',(4.66956241667986,139.782491701871,12.4197290284814));
#81950=CARTESIAN_POINT('Ctrl Pts',(4.66784838941719,139.76311613002,12.4027593730804));
#81951=CARTESIAN_POINT('Ctrl Pts',(4.66672986621822,139.750019157291,12.3917828967142));
#81952=CARTESIAN_POINT('Ctrl Pts',(4.6640785088692,139.718019701095,12.3661289065347));
#81953=CARTESIAN_POINT('Ctrl Pts',(4.66255962362434,139.698899397505,12.3517345962688));
#81954=CARTESIAN_POINT('Ctrl Pts',(4.65555368993483,139.607801821801,12.2874071340989));
#81955=CARTESIAN_POINT('Ctrl Pts',(4.65026248277115,139.530838404914,12.2450219357949));
#81956=CARTESIAN_POINT('Ctrl Pts',(4.64260116432481,139.418888895284,12.198749778483));
#81957=CARTESIAN_POINT('Ctrl Pts',(4.64045004234308,139.387362140476,12.187269026011));
#81958=CARTESIAN_POINT('Ctrl Pts',(4.63721540920876,139.340232943176,12.1723522828684));
#81959=CARTESIAN_POINT('Ctrl Pts',(4.63616584470166,139.32498044869,12.1678624212858));
#81960=CARTESIAN_POINT('Ctrl Pts',(4.63424175816761,139.297128528458,12.1602728733271));
#81961=CARTESIAN_POINT('Ctrl Pts',(4.63337073457056,139.28455969946,12.1570699758933));
#81962=CARTESIAN_POINT('Ctrl Pts',(4.63144491741864,139.256874525638,12.1504999687944));
#81963=CARTESIAN_POINT('Ctrl Pts',(4.63038743311304,139.241739707553,12.1472221734113));
#81964=CARTESIAN_POINT('Ctrl Pts',(4.62718781068581,139.196173571643,12.1382905377861));
#81965=CARTESIAN_POINT('Ctrl Pts',(4.62501822496883,139.165581647883,12.1335372445353));
#81966=CARTESIAN_POINT('Ctrl Pts',(4.61964954794539,139.090630107562,12.1248992589631));
#81967=CARTESIAN_POINT('Ctrl Pts',(4.61641907960809,139.04617038347,12.1223144581953));
#81968=CARTESIAN_POINT('Ctrl Pts',(4.60750829287687,138.924494747572,12.1221414500323));
#81969=CARTESIAN_POINT('Ctrl Pts',(4.60178273094873,138.847487272822,12.1296184158409));
#81970=CARTESIAN_POINT('Ctrl Pts',(4.59538602336788,138.758620544359,12.1471728450399));
#81971=CARTESIAN_POINT('Ctrl Pts',(4.59444923097471,138.74552392104,12.1499928459592));
#81972=CARTESIAN_POINT('Ctrl Pts',(4.59297532076422,138.724744761439,12.1548394585048));
#81973=CARTESIAN_POINT('Ctrl Pts',(4.59243085200732,138.717030087759,12.1567213155882));
#81974=CARTESIAN_POINT('Ctrl Pts',(4.59135391983659,138.701681644032,12.1606301785878));
#81975=CARTESIAN_POINT('Ctrl Pts',(4.59082144396414,138.694048065588,12.1626562288044));
#81976=CARTESIAN_POINT('Ctrl Pts',(4.58941076345201,138.673724598745,12.1682697717036));
#81977=CARTESIAN_POINT('Ctrl Pts',(4.58853991019236,138.661073209767,12.1719939654237));
#81978=CARTESIAN_POINT('Ctrl Pts',(4.58407605119098,138.595859410489,12.1923873027835));
#81979=CARTESIAN_POINT('Ctrl Pts',(4.58064013229017,138.544446853908,12.2125220829568));
#81980=CARTESIAN_POINT('Ctrl Pts',(4.57193430950254,138.417435340018,12.2728596702846));
#81981=CARTESIAN_POINT('Ctrl Pts',(4.56670385088533,138.344469215051,12.3178204197468));
#81982=CARTESIAN_POINT('Ctrl Pts',(4.55986055406412,138.260889796805,12.382815028404));
#81983=CARTESIAN_POINT('Ctrl Pts',(4.55852632032026,138.245097389695,12.395768761651));
#81984=CARTESIAN_POINT('Ctrl Pts',(4.55627798356501,138.219382540497,12.4180047009295));
#81985=CARTESIAN_POINT('Ctrl Pts',(4.55537319956294,138.209269269964,12.427060017984));
#81986=CARTESIAN_POINT('Ctrl Pts',(4.55354818068691,138.189353378723,12.4455225950455));
#81987=CARTESIAN_POINT('Ctrl Pts',(4.55262807525838,138.179552537963,12.454928692182));
#81988=CARTESIAN_POINT('Ctrl Pts',(4.55030249735283,138.155392075785,12.4789325648475));
#81989=CARTESIAN_POINT('Ctrl Pts',(4.54888799024572,138.14124686072,12.4937387315138));
#81990=CARTESIAN_POINT('Ctrl Pts',(4.54272492976738,138.081995900503,12.559087076731));
#81991=CARTESIAN_POINT('Ctrl Pts',(4.53781971062446,138.040917127637,12.6130931730742));
#81992=CARTESIAN_POINT('Ctrl Pts',(4.52753839709693,137.965961330011,12.7315704520613));
#81993=CARTESIAN_POINT('Ctrl Pts',(4.5221752102372,137.932945399868,12.7962698811426));
#81994=CARTESIAN_POINT('Ctrl Pts',(4.51611600925115,137.901146070876,12.8759801560607));
#81995=CARTESIAN_POINT('Ctrl Pts',(4.51518381645701,137.896416639259,12.8884461283159));
#81996=CARTESIAN_POINT('Ctrl Pts',(4.51371537260885,137.889213996671,12.9084487797378));
#81997=CARTESIAN_POINT('Ctrl Pts',(4.51317185874504,137.886603606834,12.9159344011284));
#81998=CARTESIAN_POINT('Ctrl Pts',(4.51209504567939,137.881539828194,12.9309410914345));
#81999=CARTESIAN_POINT('Ctrl Pts',(4.51156175816356,137.879086234145,12.938461658508));
#82000=CARTESIAN_POINT('Ctrl Pts',(4.51014620188852,137.872726347014,12.9586428481712));
#82001=CARTESIAN_POINT('Ctrl Pts',(4.50927137505273,137.868957478702,12.9713460096499));
#82002=CARTESIAN_POINT('Ctrl Pts',(4.50730704624036,137.860891289261,13.0003177730212));
#82003=CARTESIAN_POINT('Ctrl Pts',(4.50622350755357,137.856726541701,13.0166204862463));
#82004=CARTESIAN_POINT('Ctrl Pts',(4.50256585321356,137.843719040175,13.072505022373));
#82005=CARTESIAN_POINT('Ctrl Pts',(4.50004657915196,137.836571316656,13.112453402786));
#82006=CARTESIAN_POINT('Ctrl Pts',(4.49244192208725,137.821198628009,13.234396142371));
#82007=CARTESIAN_POINT('Ctrl Pts',(4.48739240194791,137.819496763251,13.3169459879458));
#82008=CARTESIAN_POINT('Ctrl Pts',(4.48073255667064,137.828164430568,13.4197005283594));
#82009=CARTESIAN_POINT('Ctrl Pts',(4.47937598140029,137.830458521735,13.4403547783222));
#82010=CARTESIAN_POINT('Ctrl Pts',(4.47710085707123,137.835161371434,13.4744478740848));
#82011=CARTESIAN_POINT('Ctrl Pts',(4.47619212898237,137.837259635268,13.4879252756146));
#82012=CARTESIAN_POINT('Ctrl Pts',(4.47436759543913,137.841903277184,13.5146855496282));
#82013=CARTESIAN_POINT('Ctrl Pts',(4.4734520562467,137.844444332442,13.5279670530128));
#82014=CARTESIAN_POINT('Ctrl Pts',(4.47115513176393,137.851336379611,13.5609065787977));
#82015=CARTESIAN_POINT('Ctrl Pts',(4.46976518431913,137.855963689517,13.580501673713));
#82016=CARTESIAN_POINT('Ctrl Pts',(4.46669507625253,137.8671641113,13.6230271568453));
#82017=CARTESIAN_POINT('Ctrl Pts',(4.46500937475407,137.873936130758,13.645895540348));
#82018=CARTESIAN_POINT('Ctrl Pts',(4.46295069534819,137.882951217905,13.6732582824354));
#82019=CARTESIAN_POINT('Ctrl Pts',(4.46259508558876,137.884534942957,13.6779648440736));
#82020=CARTESIAN_POINT('Ctrl Pts',(4.46223878927246,137.886148214676,13.6826607672995));
#82021=CARTESIAN_POINT('Ctrl Pts',(4.36393196101569,137.88614821267,13.68266076146));
#82022=CARTESIAN_POINT('Ctrl Pts',(4.36405144554922,137.885570957912,13.6809804840216));
#82023=CARTESIAN_POINT('Ctrl Pts',(4.36417071710138,137.884997500726,13.6792988871397));
#82024=CARTESIAN_POINT('Ctrl Pts',(4.36511745336918,137.880467884761,13.6659172675373));
#82025=CARTESIAN_POINT('Ctrl Pts',(4.36593501476838,137.876691993988,13.6541564027392));
#82026=CARTESIAN_POINT('Ctrl Pts',(4.36774537884669,137.868659432261,13.6277150273824));
#82027=CARTESIAN_POINT('Ctrl Pts',(4.36873355853044,137.864502055418,13.6130065211228));
#82028=CARTESIAN_POINT('Ctrl Pts',(4.37190087553844,137.851974119104,13.5651428538918));
#82029=CARTESIAN_POINT('Ctrl Pts',(4.37403970187651,137.844760289681,13.5317016580991));
#82030=CARTESIAN_POINT('Ctrl Pts',(4.38212051367179,137.822880257343,13.4034012443494));
#82031=CARTESIAN_POINT('Ctrl Pts',(4.38795625824047,137.818370028255,13.3072028793761));
#82032=CARTESIAN_POINT('Ctrl Pts',(4.39541264590132,137.827006824096,13.1925575619454));
#82033=CARTESIAN_POINT('Ctrl Pts',(4.39665886850501,137.828894951517,13.1736284566379));
#82034=CARTESIAN_POINT('Ctrl Pts',(4.39879815104802,137.832875922405,13.1415945001671));
#82035=CARTESIAN_POINT('Ctrl Pts',(4.39968372209413,137.834733406378,13.1284638339523));
#82036=CARTESIAN_POINT('Ctrl Pts',(4.40151837989025,137.839005956364,13.1015466574256));
#82037=CARTESIAN_POINT('Ctrl Pts',(4.40246812080317,137.841445848996,13.0877662885772));
#82038=CARTESIAN_POINT('Ctrl Pts',(4.40495594458373,137.848421139151,13.0520861656815));
#82039=CARTESIAN_POINT('Ctrl Pts',(4.40650573473733,137.853335598707,13.0302672166213));
#82040=CARTESIAN_POINT('Ctrl Pts',(4.41000398135935,137.865675142677,12.9819447172741));
#82041=CARTESIAN_POINT('Ctrl Pts',(4.41196102243564,137.873414009073,12.9555354072992));
#82042=CARTESIAN_POINT('Ctrl Pts',(4.41903390439452,137.904350128257,12.8622095710433));
#82043=CARTESIAN_POINT('Ctrl Pts',(4.42427000287582,137.932645617921,12.7971457821304));
#82044=CARTESIAN_POINT('Ctrl Pts',(4.43246509954726,137.98640693346,12.6988116605395));
#82045=CARTESIAN_POINT('Ctrl Pts',(4.43545465610256,138.008096517766,12.6636616749825));
#82046=CARTESIAN_POINT('Ctrl Pts',(4.43918092603017,138.038273979434,12.6200616940964));
#82047=CARTESIAN_POINT('Ctrl Pts',(4.43999893617289,138.045103481009,12.6105032970942));
#82048=CARTESIAN_POINT('Ctrl Pts',(4.44132976945041,138.056571872968,12.5949497583282));
#82049=CARTESIAN_POINT('Ctrl Pts',(4.44184780296393,138.061127541206,12.5888945271764));
#82050=CARTESIAN_POINT('Ctrl Pts',(4.44293118427199,138.070854880423,12.5762217671127));
#82051=CARTESIAN_POINT('Ctrl Pts',(4.44349564910471,138.076039418751,12.5696148696357));
#82052=CARTESIAN_POINT('Ctrl Pts',(4.44508926513067,138.090993969594,12.5509716969043));
#82053=CARTESIAN_POINT('Ctrl Pts',(4.44610748031988,138.10093191704,12.5390716195291));
#82054=CARTESIAN_POINT('Ctrl Pts',(4.44846565436185,138.124767264935,12.5116494425902));
#82055=CARTESIAN_POINT('Ctrl Pts',(4.44979554667951,138.138847483882,12.4962927260749));
#82056=CARTESIAN_POINT('Ctrl Pts',(4.45499881528896,138.196104154233,12.4370786174421));
#82057=CARTESIAN_POINT('Ctrl Pts',(4.45876049827389,138.242283140347,12.3962590278988));
#82058=CARTESIAN_POINT('Ctrl Pts',(4.46618139536436,138.337889763152,12.324250936474));
#82059=CARTESIAN_POINT('Ctrl Pts',(4.46982493899011,138.386858839811,12.2927597084906));
#82060=CARTESIAN_POINT('Ctrl Pts',(4.47480937433507,138.454333158549,12.2561176562691));
#82061=CARTESIAN_POINT('Ctrl Pts',(4.47603184899913,138.470925040854,12.2476111583778));
#82062=CARTESIAN_POINT('Ctrl Pts',(4.47815216226197,138.499717156917,12.233702705061));
#82063=CARTESIAN_POINT('Ctrl Pts',(4.4790431412539,138.511820390467,12.228107520195));
#82064=CARTESIAN_POINT('Ctrl Pts',(4.48089399240221,138.536952672647,12.2170031039055));
#82065=CARTESIAN_POINT('Ctrl Pts',(4.48185460619846,138.549991150139,12.2115207356431));
#82066=CARTESIAN_POINT('Ctrl Pts',(4.48440903809402,138.584628060835,12.1976854423856));
#82067=CARTESIAN_POINT('Ctrl Pts',(4.48601578559118,138.606378616602,12.1897327766417));
#82068=CARTESIAN_POINT('Ctrl Pts',(4.4931325853762,138.702505440369,12.1577655545326));
#82069=CARTESIAN_POINT('Ctrl Pts',(4.49884882926304,138.77892303634,12.140550100256));
#82070=CARTESIAN_POINT('Ctrl Pts',(4.50860860000882,138.91080441141,12.1243571727766));
#82071=CARTESIAN_POINT('Ctrl Pts',(4.51262373042449,138.965543450837,12.1214815909853));
#82072=CARTESIAN_POINT('Ctrl Pts',(4.51752718940067,139.034780684684,12.1226744405384));
#82073=CARTESIAN_POINT('Ctrl Pts',(4.51854330849807,139.049268575211,12.1231916792009));
#82074=CARTESIAN_POINT('Ctrl Pts',(4.52011336535685,139.071928489867,12.1244199145468));
#82075=CARTESIAN_POINT('Ctrl Pts',(4.52067620589444,139.08010842505,12.12494898181));
#82076=CARTESIAN_POINT('Ctrl Pts',(4.52176430268376,139.096045946824,12.1261470063593));
#82077=CARTESIAN_POINT('Ctrl Pts',(4.52228992609296,139.103803579192,12.1268075620268));
#82078=CARTESIAN_POINT('Ctrl Pts',(4.5236467585367,139.123964052179,12.1287257481483));
#82079=CARTESIAN_POINT('Ctrl Pts',(4.52447167108756,139.136354925762,12.1301034983764));
#82080=CARTESIAN_POINT('Ctrl Pts',(4.52630140630557,139.164072242667,12.1336317889699));
#82081=CARTESIAN_POINT('Ctrl Pts',(4.52730145025654,139.17938304448,12.1358882036811));
#82082=CARTESIAN_POINT('Ctrl Pts',(4.53052638323222,139.229093759829,12.1442184000523));
#82083=CARTESIAN_POINT('Ctrl Pts',(4.532709368715,139.263270248595,12.1515209462001));
#82084=CARTESIAN_POINT('Ctrl Pts',(4.54072345642699,139.388240783638,12.1840966097589));
#82085=CARTESIAN_POINT('Ctrl Pts',(4.54645924088612,139.476218579563,12.2187111005218));
#82086=CARTESIAN_POINT('Ctrl Pts',(4.55381453348094,139.576097718916,12.272586698782));
#82087=CARTESIAN_POINT('Ctrl Pts',(4.55507685762903,139.592835939148,12.2821531778624));
#82088=CARTESIAN_POINT('Ctrl Pts',(4.5572350369178,139.620714909347,12.2990079817026));
#82089=CARTESIAN_POINT('Ctrl Pts',(4.558123062895,139.631980867963,12.3060824092028));
#82090=CARTESIAN_POINT('Ctrl Pts',(4.55995520291427,139.654789228345,12.3209494316444));
#82091=CARTESIAN_POINT('Ctrl Pts',(4.56089984990756,139.666318031238,12.3287589376558));
#82092=CARTESIAN_POINT('Ctrl Pts',(4.56335644337155,139.695690389042,12.3494246312138));
#82093=CARTESIAN_POINT('Ctrl Pts',(4.56487953888226,139.713316464095,12.3625789854718));
#82094=CARTESIAN_POINT('Ctrl Pts',(4.56830469299409,139.751646645332,12.3928920044727));
#82095=CARTESIAN_POINT('Ctrl Pts',(4.57021475860546,139.772151814534,12.4102815121178));
#82096=CARTESIAN_POINT('Ctrl Pts',(4.57696380766331,139.841659938885,12.473441964599));
#82097=CARTESIAN_POINT('Ctrl Pts',(4.58191072974019,139.887333722784,12.5226794632737));
#82098=CARTESIAN_POINT('Ctrl Pts',(4.59019301095787,139.956868001116,12.6118027880748));
#82099=CARTESIAN_POINT('Ctrl Pts',(4.59353759076802,139.98302189817,12.6497073321664));
#82100=CARTESIAN_POINT('Ctrl Pts',(4.59761241334511,140.013083434356,12.69925094068));
#82101=CARTESIAN_POINT('Ctrl Pts',(4.59844390567549,140.019118895127,12.709547476215));
#82102=CARTESIAN_POINT('Ctrl Pts',(4.59979041105337,140.028745040424,12.7265572283095));
#82103=CARTESIAN_POINT('Ctrl Pts',(4.60031087778232,140.032428901258,12.7332164897527));
#82104=CARTESIAN_POINT('Ctrl Pts',(4.60139239095569,140.040010484408,12.7472408522745));
#82105=CARTESIAN_POINT('Ctrl Pts',(4.60195266030373,140.043895048661,12.7546124121708));
#82106=CARTESIAN_POINT('Ctrl Pts',(4.60352044291731,140.054630357284,12.7755193180085));
#82107=CARTESIAN_POINT('Ctrl Pts',(4.60451757337406,140.061298553084,12.789147173642));
#82108=CARTESIAN_POINT('Ctrl Pts',(4.60681617704818,140.076233332756,12.8212250652354));
#82109=CARTESIAN_POINT('Ctrl Pts',(4.60810828263103,140.084292041307,12.8397669248675));
#82110=CARTESIAN_POINT('Ctrl Pts',(4.61303441236683,140.113487929548,12.9119723362309));
#82111=CARTESIAN_POINT('Ctrl Pts',(4.61656813258606,140.131150968644,12.9669549354017));
#82112=CARTESIAN_POINT('Ctrl Pts',(4.62369915489038,140.158243925247,13.0789229725753));
#82113=CARTESIAN_POINT('Ctrl Pts',(4.62728745852814,140.167657048175,13.1357437981369));
#82114=CARTESIAN_POINT('Ctrl Pts',(4.63236949198691,140.174811387542,13.2141818495386));
#82115=CARTESIAN_POINT('Ctrl Pts',(4.63375564769825,140.176168330469,13.235389481568));
#82116=CARTESIAN_POINT('Ctrl Pts',(4.63607036238583,140.177458633001,13.2703978877468));
#82117=CARTESIAN_POINT('Ctrl Pts',(4.63698848541258,140.177724449237,13.2841819109652));
#82118=CARTESIAN_POINT('Ctrl Pts',(4.63882469534848,140.177771649256,13.3115248904123));
#82119=CARTESIAN_POINT('Ctrl Pts',(4.63974239199469,140.177560937698,13.3250817097173));
#82120=CARTESIAN_POINT('Ctrl Pts',(4.64203131354055,140.176460626093,13.3586087089169));
#82121=CARTESIAN_POINT('Ctrl Pts',(4.64341083814956,140.175296578742,13.3785649559327));
#82122=CARTESIAN_POINT('Ctrl Pts',(4.64645058016099,140.171654284553,13.4219712288838));
#82123=CARTESIAN_POINT('Ctrl Pts',(4.64811609531217,140.168978497663,13.445395622061));
#82124=CARTESIAN_POINT('Ctrl Pts',(4.65344504089559,140.158288955321,13.5192431442962));
#82125=CARTESIAN_POINT('Ctrl Pts',(4.65717143103521,140.147699848218,13.5692305437004));
#82126=CARTESIAN_POINT('Ctrl Pts',(4.66574541046944,140.116130651548,13.6816673058308));
#82127=CARTESIAN_POINT('Ctrl Pts',(4.67059451055174,140.093087961002,13.7433706977481));
#82128=CARTESIAN_POINT('Ctrl Pts',(4.67622267179672,140.059099350073,13.8153596334413));
#82129=CARTESIAN_POINT('Ctrl Pts',(4.67719247943068,140.052963739254,13.8277825223399));
#82130=CARTESIAN_POINT('Ctrl Pts',(4.67870770080726,140.042911202402,13.8472625908496));
#82131=CARTESIAN_POINT('Ctrl Pts',(4.67926108265696,140.039138703909,13.854392354927));
#82132=CARTESIAN_POINT('Ctrl Pts',(4.68034622370873,140.031533877106,13.8684145496831));
#82133=CARTESIAN_POINT('Ctrl Pts',(4.68087812532943,140.027705017169,13.8753083040336));
#82134=CARTESIAN_POINT('Ctrl Pts',(4.68227426409516,140.017395059978,13.8934396559565));
#82135=CARTESIAN_POINT('Ctrl Pts',(4.68313148917211,140.010796828725,13.9046099063863));
#82136=CARTESIAN_POINT('Ctrl Pts',(4.68774662151028,139.97389519895,13.9647879669938));
#82137=CARTESIAN_POINT('Ctrl Pts',(4.69133062532774,139.940207737117,14.0116360525169));
#82138=CARTESIAN_POINT('Ctrl Pts',(4.70001614916104,139.85012668372,14.1192829645026));
#82139=CARTESIAN_POINT('Ctrl Pts',(4.70508789445232,139.790499139157,14.1769547209795));
#82140=CARTESIAN_POINT('Ctrl Pts',(4.71177352565144,139.708945158725,14.2407039839293));
#82141=CARTESIAN_POINT('Ctrl Pts',(4.71313081911521,139.692231536635,14.2530701117452));
#82142=CARTESIAN_POINT('Ctrl Pts',(4.71541086370179,139.663973860387,14.272841975089));
#82143=CARTESIAN_POINT('Ctrl Pts',(4.7163238406002,139.652611701981,14.2805002475559));
#82144=CARTESIAN_POINT('Ctrl Pts',(4.71816021423738,139.629683740871,14.2953789623037));
#82145=CARTESIAN_POINT('Ctrl Pts',(4.71908339302365,139.618121027329,14.3026002496012));
#82146=CARTESIAN_POINT('Ctrl Pts',(4.7214070166361,139.588944843933,14.3201251657542));
#82147=CARTESIAN_POINT('Ctrl Pts',(4.72281633185988,139.571184650181,14.3301744453635));
#82148=CARTESIAN_POINT('Ctrl Pts',(4.72593503232002,139.531768091603,14.3511449146905));
#82149=CARTESIAN_POINT('Ctrl Pts',(4.72765022542898,139.510017646029,14.3618685404456));
#82150=CARTESIAN_POINT('Ctrl Pts',(4.7332399845748,139.438878371924,14.3942523548073));
#82151=CARTESIAN_POINT('Ctrl Pts',(4.7371847574608,139.388331487331,14.4131936820384));
#82152=CARTESIAN_POINT('Ctrl Pts',(4.74561494293015,139.278345973876,14.446003020223));
#82153=CARTESIAN_POINT('Ctrl Pts',(4.75009272050613,139.218756826673,14.4588554843534));
#82154=CARTESIAN_POINT('Ctrl Pts',(4.75539634104214,139.144466347125,14.4689411098155));
#82155=CARTESIAN_POINT('Ctrl Pts',(4.75638385783457,139.130461806291,14.4705868634003));
#82156=CARTESIAN_POINT('Ctrl Pts',(4.75792006975012,139.10835411962,14.4727831497456));
#82157=CARTESIAN_POINT('Ctrl Pts',(4.75847708591668,139.100269516016,14.4735020092046));
#82158=CARTESIAN_POINT('Ctrl Pts',(4.75956319476192,139.084357557645,14.4747512070803));
#82159=CARTESIAN_POINT('Ctrl Pts',(4.76009251770535,139.076531162586,14.4752870217027));
#82160=CARTESIAN_POINT('Ctrl Pts',(4.76147271160568,139.055954446016,14.4764893373811));
#82161=CARTESIAN_POINT('Ctrl Pts',(4.76231686259653,139.043197181486,14.4770268041078));
#82162=CARTESIAN_POINT('Ctrl Pts',(4.76708106937081,138.970397808263,14.4789085684375));
#82163=CARTESIAN_POINT('Ctrl Pts',(4.77080996691682,138.910324180704,14.4758663584762));
#82164=CARTESIAN_POINT('Ctrl Pts',(4.7794828824598,138.771227878268,14.4580947938973));
#82165=CARTESIAN_POINT('Ctrl Pts',(4.78440450500348,138.692969663893,14.4398469853316));
#82166=CARTESIAN_POINT('Ctrl Pts',(4.79093658881197,138.597271989458,14.4069544203392));
#82167=CARTESIAN_POINT('Ctrl Pts',(4.79230996391295,138.577558127979,14.399582064135));
#82168=CARTESIAN_POINT('Ctrl Pts',(4.79460931270489,138.545309446201,14.3865268445546));
#82169=CARTESIAN_POINT('Ctrl Pts',(4.79552514522176,138.532657413872,14.3811452094138));
#82170=CARTESIAN_POINT('Ctrl Pts',(4.7973613343609,138.507692682811,14.3700061887944));
#82171=CARTESIAN_POINT('Ctrl Pts',(4.79828137594904,138.495379685096,14.3642546920139));
#82172=CARTESIAN_POINT('Ctrl Pts',(4.80058519922273,138.465048114944,14.3494418718262));
#82173=CARTESIAN_POINT('Ctrl Pts',(4.80197752457061,138.447158170469,14.3401286390274));
#82174=CARTESIAN_POINT('Ctrl Pts',(4.80839431260371,138.366747332532,14.295607347492));
#82175=CARTESIAN_POINT('Ctrl Pts',(4.81359856872788,138.307294340155,14.2551956895674));
#82176=CARTESIAN_POINT('Ctrl Pts',(4.82389289207144,138.198952880956,14.1660931398391));
#82177=CARTESIAN_POINT('Ctrl Pts',(4.82895578127485,138.149908999472,14.1180100622798));
#82178=CARTESIAN_POINT('Ctrl Pts',(4.8347690927021,138.096412414699,14.0555212151996));
#82179=CARTESIAN_POINT('Ctrl Pts',(4.83572802351223,138.087682832753,14.0449565477353));
#82180=CARTESIAN_POINT('Ctrl Pts',(4.83723034029155,138.074130023621,14.0279590704146));
#82181=CARTESIAN_POINT('Ctrl Pts',(4.83778148033555,138.069185109359,14.0216254363205));
#82182=CARTESIAN_POINT('Ctrl Pts',(4.83886614018695,138.05950013888,14.0089553425991));
#82183=CARTESIAN_POINT('Ctrl Pts',(4.8393997471927,138.054758377273,14.002620771819));
#82184=CARTESIAN_POINT('Ctrl Pts',(4.84080630864375,138.04233319953,13.9856683723449));
#82185=CARTESIAN_POINT('Ctrl Pts',(4.84167205862026,138.034762301955,13.9749689173073));
#82186=CARTESIAN_POINT('Ctrl Pts',(4.84613570953641,137.996245534011,13.9185617610804));
#82187=CARTESIAN_POINT('Ctrl Pts',(4.84957558321192,137.968359073284,13.8708415493272));
#82188=CARTESIAN_POINT('Ctrl Pts',(4.85609982431312,137.921714791742,13.7763534625273));
#82189=CARTESIAN_POINT('Ctrl Pts',(4.85917930024266,137.902422683108,13.7300326109271));
#82190=CARTESIAN_POINT('Ctrl Pts',(4.86231567683356,137.88614821265,13.6826607614027));
#82191=CARTESIAN_POINT('Origin',(1.13913288526384,139.,13.3));
#82192=CARTESIAN_POINT('',(5.46043320712868,137.886148212654,13.6826607614143));
#82193=CARTESIAN_POINT('',(5.36197089565136,137.88614821265,13.6826607614027));
#82194=CARTESIAN_POINT('',(1.13913288526384,137.88614821265,13.6826607614027));
#82195=CARTESIAN_POINT('Ctrl Pts',(5.46043320712869,137.886148212658,13.6826607614259));
#82196=CARTESIAN_POINT('Ctrl Pts',(5.46002446106101,137.88816324508,13.6885261327719));
#82197=CARTESIAN_POINT('Ctrl Pts',(5.45961795346396,137.890224662102,13.6943757490642));
#82198=CARTESIAN_POINT('Ctrl Pts',(5.45489137935915,137.914852864487,13.7625397852664));
#82199=CARTESIAN_POINT('Ctrl Pts',(5.45080521369556,137.942597297947,13.8228661278637));
#82200=CARTESIAN_POINT('Ctrl Pts',(5.44214953865667,138.011644698042,13.9447428096011));
#82201=CARTESIAN_POINT('Ctrl Pts',(5.43759116393617,138.053964360087,14.0053754723978));
#82202=CARTESIAN_POINT('Ctrl Pts',(5.43151568350696,138.114716689762,14.0770297290376));
#82203=CARTESIAN_POINT('Ctrl Pts',(5.43019758881392,138.128150371337,14.0920731568807));
#82204=CARTESIAN_POINT('Ctrl Pts',(5.42796853572488,138.151229936349,14.1166195299311));
#82205=CARTESIAN_POINT('Ctrl Pts',(5.42706653844709,138.160665667421,14.1263146676485));
#82206=CARTESIAN_POINT('Ctrl Pts',(5.42524078930307,138.179941204172,14.1454492829544));
#82207=CARTESIAN_POINT('Ctrl Pts',(5.42431706408592,138.189782089481,14.154884687505));
#82208=CARTESIAN_POINT('Ctrl Pts',(5.4219690256319,138.215003859897,14.1782405098876));
#82209=CARTESIAN_POINT('Ctrl Pts',(5.42053530355722,138.230592306832,14.1919288311764));
#82210=CARTESIAN_POINT('Ctrl Pts',(5.41330437062935,138.31008937633,14.2581004539301));
#82211=CARTESIAN_POINT('Ctrl Pts',(5.40726178334422,138.379030729362,14.3041543804792));
#82212=CARTESIAN_POINT('Ctrl Pts',(5.39822406142292,138.487953202648,14.36138270757));
#82213=CARTESIAN_POINT('Ctrl Pts',(5.39526166879702,138.524638566486,14.3783120996047));
#82214=CARTESIAN_POINT('Ctrl Pts',(5.39114456469103,138.577701543385,14.399563874362));
#82215=CARTESIAN_POINT('Ctrl Pts',(5.38994572947525,138.593413005586,14.405469933359));
#82216=CARTESIAN_POINT('Ctrl Pts',(5.38782761132128,138.621721748052,14.4154261609528));
#82217=CARTESIAN_POINT('Ctrl Pts',(5.38690309948158,138.634271093557,14.4196036621991));
#82218=CARTESIAN_POINT('Ctrl Pts',(5.38544377375865,138.654430520457,14.42593929359));
#82219=CARTESIAN_POINT('Ctrl Pts',(5.38490184316546,138.661996217212,14.428233579714));
#82220=CARTESIAN_POINT('Ctrl Pts',(5.38382515754415,138.677198661235,14.4326770425865));
#82221=CARTESIAN_POINT('Ctrl Pts',(5.3832904565881,138.684835163802,14.4348255911629));
#82222=CARTESIAN_POINT('Ctrl Pts',(5.3818664506311,138.705386448751,14.4403842856765));
#82223=CARTESIAN_POINT('Ctrl Pts',(5.38098474433417,138.718338897941,14.4436522743087));
#82224=CARTESIAN_POINT('Ctrl Pts',(5.37539625060192,138.801670046327,14.4631755655884));
#82225=CARTESIAN_POINT('Ctrl Pts',(5.37096328308412,138.873371013347,14.4731495620282));
#82226=CARTESIAN_POINT('Ctrl Pts',(5.36226309479941,139.013993082003,14.4796588156711));
#82227=CARTESIAN_POINT('Ctrl Pts',(5.35801364830462,139.08258331411,14.4768472077239));
#82228=CARTESIAN_POINT('Ctrl Pts',(5.35227702900749,139.17056402731,14.4655087941148));
#82229=CARTESIAN_POINT('Ctrl Pts',(5.3509572262854,139.190521077112,14.4624132127218));
#82230=CARTESIAN_POINT('Ctrl Pts',(5.34872614789819,139.223703056358,14.4563888385664));
#82231=CARTESIAN_POINT('Ctrl Pts',(5.34782387136277,139.236975189682,14.4537421449516));
#82232=CARTESIAN_POINT('Ctrl Pts',(5.34599825365736,139.263514417396,14.4479725229121));
#82233=CARTESIAN_POINT('Ctrl Pts',(5.34507495036747,139.276778758361,14.4448468252501));
#82234=CARTESIAN_POINT('Ctrl Pts',(5.34272945845369,139.310060455339,14.4363919186335));
#82235=CARTESIAN_POINT('Ctrl Pts',(5.34129790299485,139.329996284705,14.4307636517813));
#82236=CARTESIAN_POINT('Ctrl Pts',(5.33404962410678,139.429006375878,14.3999699582176));
#82237=CARTESIAN_POINT('Ctrl Pts',(5.32798546452156,139.505402157916,14.3670261015879));
#82238=CARTESIAN_POINT('Ctrl Pts',(5.31773151608493,139.627055005208,14.298552000968));
#82239=CARTESIAN_POINT('Ctrl Pts',(5.31357696525345,139.674355879607,14.2672380012395));
#82240=CARTESIAN_POINT('Ctrl Pts',(5.3086305678388,139.729824927433,14.224461954189));
#82241=CARTESIAN_POINT('Ctrl Pts',(5.30769420943759,139.740287853526,14.2161049402823));
#82242=CARTESIAN_POINT('Ctrl Pts',(5.3062208159242,139.756724393485,14.2025110993704));
#82243=CARTESIAN_POINT('Ctrl Pts',(5.30567643815709,139.762791170154,14.1973893983234));
#82244=CARTESIAN_POINT('Ctrl Pts',(5.30459952369469,139.774789452427,14.1870505924745));
#82245=CARTESIAN_POINT('Ctrl Pts',(5.30406697676924,139.780721181815,14.1818343915343));
#82246=CARTESIAN_POINT('Ctrl Pts',(5.30265585783676,139.796418659861,14.1677478976448));
#82247=CARTESIAN_POINT('Ctrl Pts',(5.30178464546688,139.806088913321,14.1587722606016));
#82248=CARTESIAN_POINT('Ctrl Pts',(5.29610633496943,139.868792904912,14.0985796278385));
#82249=CARTESIAN_POINT('Ctrl Pts',(5.29158645602547,139.917074461824,14.0426356746975));
#82250=CARTESIAN_POINT('Ctrl Pts',(5.28413421484998,139.98694569906,13.944379941946));
#82251=CARTESIAN_POINT('Ctrl Pts',(5.28123303980634,140.011779282716,13.9046400816903));
#82252=CARTESIAN_POINT('Ctrl Pts',(5.27684118012883,140.044936647546,13.8437902210852));
#82253=CARTESIAN_POINT('Ctrl Pts',(5.27540258427144,140.055124874687,13.8237478491097));
#82254=CARTESIAN_POINT('Ctrl Pts',(5.27269643377183,140.072973752593,13.7859980168318));
#82255=CARTESIAN_POINT('Ctrl Pts',(5.27143412006633,140.080784959081,13.7683700985155));
#82256=CARTESIAN_POINT('Ctrl Pts',(5.26927137251866,140.093275667117,13.7382033973851));
#82257=CARTESIAN_POINT('Ctrl Pts',(5.26837869667091,140.098180658948,13.7257618079418));
#82258=CARTESIAN_POINT('Ctrl Pts',(5.2666585518942,140.107149749537,13.701824705116));
#82259=CARTESIAN_POINT('Ctrl Pts',(5.26583240325275,140.111249295488,13.690344265179));
#82260=CARTESIAN_POINT('Ctrl Pts',(5.26361867636485,140.1216796052,13.6596381261013));
#82261=CARTESIAN_POINT('Ctrl Pts',(5.26222098908987,140.127693956648,13.6403101089013));
#82262=CARTESIAN_POINT('Ctrl Pts',(5.25473715352687,140.156889013847,13.5371924231291));
#82263=CARTESIAN_POINT('Ctrl Pts',(5.24837389754839,140.171233318188,13.4511951666371));
#82264=CARTESIAN_POINT('Ctrl Pts',(5.23918242482233,140.178079517161,13.3262192177704));
#82265=CARTESIAN_POINT('Ctrl Pts',(5.23637918385243,140.178309618161,13.287936508896));
#82266=CARTESIAN_POINT('Ctrl Pts',(5.23245462858375,140.175980543361,13.2334424843269));
#82267=CARTESIAN_POINT('Ctrl Pts',(5.23129275563309,140.174948055718,13.2171914202445));
#82268=CARTESIAN_POINT('Ctrl Pts',(5.22923237313752,140.172491529246,13.1880808747246));
#82269=CARTESIAN_POINT('Ctrl Pts',(5.22832901591736,140.171191988838,13.1752136352076));
#82270=CARTESIAN_POINT('Ctrl Pts',(5.2268948228637,140.168763938468,13.1545783176251));
#82271=CARTESIAN_POINT('Ctrl Pts',(5.22635726625967,140.167769292725,13.146795890166));
#82272=CARTESIAN_POINT('Ctrl Pts',(5.22528072541546,140.165603837945,13.1311014771666));
#82273=CARTESIAN_POINT('Ctrl Pts',(5.22474191885508,140.164430065478,13.1231903563779));
#82274=CARTESIAN_POINT('Ctrl Pts',(5.22329330009636,140.161031692572,13.1017895798923));
#82275=CARTESIAN_POINT('Ctrl Pts',(5.22239154968564,140.158652585027,13.0883252760078));
#82276=CARTESIAN_POINT('Ctrl Pts',(5.21703254643454,140.142951649458,13.007688742377));
#82277=CARTESIAN_POINT('Ctrl Pts',(5.2128179361966,140.124024881949,12.9417337691464));
#82278=CARTESIAN_POINT('Ctrl Pts',(5.20402911219146,140.073036587565,12.8089555546234));
#82279=CARTESIAN_POINT('Ctrl Pts',(5.19946635320272,140.040200148925,12.7427619809579));
#82280=CARTESIAN_POINT('Ctrl Pts',(5.19343985944495,139.991255398892,12.6636991460309));
#82281=CARTESIAN_POINT('Ctrl Pts',(5.19217869330606,139.980717500391,12.6475744042077));
#82282=CARTESIAN_POINT('Ctrl Pts',(5.19001729450854,139.962202929968,12.6207067323857));
#82283=CARTESIAN_POINT('Ctrl Pts',(5.18912479540248,139.954429773761,12.609827844783));
#82284=CARTESIAN_POINT('Ctrl Pts',(5.18740457711586,139.939216574442,12.5892848864221));
#82285=CARTESIAN_POINT('Ctrl Pts',(5.18657817167717,139.931808286969,12.579599386985));
#82286=CARTESIAN_POINT('Ctrl Pts',(5.1843627215402,139.911693527125,12.5541310590791));
#82287=CARTESIAN_POINT('Ctrl Pts',(5.18296353854975,139.898728391906,12.5385587656547));
#82288=CARTESIAN_POINT('Ctrl Pts',(5.17548930001018,139.828148157338,12.4581005444611));
#82289=CARTESIAN_POINT('Ctrl Pts',(5.1691384084212,139.763903116814,12.3994051145462));
#82290=CARTESIAN_POINT('Ctrl Pts',(5.15995310227539,139.662832474261,12.325721871847));
#82291=CARTESIAN_POINT('Ctrl Pts',(5.15714400860173,139.630768346918,12.3046626998926));
#82292=CARTESIAN_POINT('Ctrl Pts',(5.15321234242267,139.583687971997,12.2769315243276));
#82293=CARTESIAN_POINT('Ctrl Pts',(5.15204908140638,139.569472242263,12.2689509355662));
#82294=CARTESIAN_POINT('Ctrl Pts',(5.14998652473619,139.543680150179,12.2551677366288));
#82295=CARTESIAN_POINT('Ctrl Pts',(5.14908236737525,139.532165184006,12.2492560654022));
#82296=CARTESIAN_POINT('Ctrl Pts',(5.14764722153498,139.513515163085,12.2400665949988));
#82297=CARTESIAN_POINT('Ctrl Pts',(5.14710949749855,139.506441005316,12.2366683656637));
#82298=CARTESIAN_POINT('Ctrl Pts',(5.14603295479684,139.492092509752,12.2299514312896));
#82299=CARTESIAN_POINT('Ctrl Pts',(5.14549430901002,139.484817326175,12.2266355944024));
#82300=CARTESIAN_POINT('Ctrl Pts',(5.1440466535762,139.465022873531,12.2178561312979));
#82301=CARTESIAN_POINT('Ctrl Pts',(5.14314568740958,139.452441012194,12.2125356117842));
#82302=CARTESIAN_POINT('Ctrl Pts',(5.13777132229715,139.376016312284,12.1817738775187));
#82303=CARTESIAN_POINT('Ctrl Pts',(5.13354246770266,139.310132088449,12.1617389053632));
#82304=CARTESIAN_POINT('Ctrl Pts',(5.12624270275035,139.194537873567,12.137378054485));
#82305=CARTESIAN_POINT('Ctrl Pts',(5.1231891490699,139.14561508974,12.1302433457637));
#82306=CARTESIAN_POINT('Ctrl Pts',(5.11859910323767,139.073335254997,12.1243077918332));
#82307=CARTESIAN_POINT('Ctrl Pts',(5.117120571124,139.050229598418,12.1230942614668));
#82308=CARTESIAN_POINT('Ctrl Pts',(5.11434817995884,139.007420022483,12.1221088004746));
#82309=CARTESIAN_POINT('Ctrl Pts',(5.1130600619896,138.987728580659,12.1221493840044));
#82310=CARTESIAN_POINT('Ctrl Pts',(5.11086673756029,138.954609548468,12.1230482157722));
#82311=CARTESIAN_POINT('Ctrl Pts',(5.10996983981387,138.941178525143,12.1236429945711));
#82312=CARTESIAN_POINT('Ctrl Pts',(5.10814203211504,138.914053806901,12.1253098649754));
#82313=CARTESIAN_POINT('Ctrl Pts',(5.10721094914297,138.900362844717,12.1263918580319));
#82314=CARTESIAN_POINT('Ctrl Pts',(5.10481735263694,138.865506493577,12.1297608443803));
#82315=CARTESIAN_POINT('Ctrl Pts',(5.10334465581804,138.844379268575,12.1323826525394));
#82316=CARTESIAN_POINT('Ctrl Pts',(5.09653517714688,138.748189667766,12.146976345681));
#82317=CARTESIAN_POINT('Ctrl Pts',(5.09099781490139,138.674334791385,12.1656231760198));
#82318=CARTESIAN_POINT('Ctrl Pts',(5.0807052314438,138.542410946377,12.2128833947779));
#82319=CARTESIAN_POINT('Ctrl Pts',(5.07598418768399,138.483882653435,12.2394178119525));
#82320=CARTESIAN_POINT('Ctrl Pts',(5.07058511479857,138.41688720055,12.2766571974022));
#82321=CARTESIAN_POINT('Ctrl Pts',(5.06971362324848,138.406068165333,12.28289821751));
#82322=CARTESIAN_POINT('Ctrl Pts',(5.06831714345676,138.388693213285,12.2932928696371));
#82323=CARTESIAN_POINT('Ctrl Pts',(5.06778602303979,138.382075689661,12.2973411384468));
#82324=CARTESIAN_POINT('Ctrl Pts',(5.06670867198228,138.3686239485,12.3057540118932));
#82325=CARTESIAN_POINT('Ctrl Pts',(5.0661628204404,138.361793916912,12.310124346928));
#82326=CARTESIAN_POINT('Ctrl Pts',(5.06467182065119,138.343117147358,12.3223487380023));
#82327=CARTESIAN_POINT('Ctrl Pts',(5.06373555662262,138.331366201462,12.3303475056441));
#82328=CARTESIAN_POINT('Ctrl Pts',(5.05957846210499,138.279261701283,12.3672123663483));
#82329=CARTESIAN_POINT('Ctrl Pts',(5.05647780331447,138.240607803186,12.3984008790417));
#82330=CARTESIAN_POINT('Ctrl Pts',(5.05060708043993,138.170805706264,12.4624056776712));
#82331=CARTESIAN_POINT('Ctrl Pts',(5.04783747499948,138.139355236226,12.494755946986));
#82332=CARTESIAN_POINT('Ctrl Pts',(5.04292485313103,138.087712923279,12.5543667268897));
#82333=CARTESIAN_POINT('Ctrl Pts',(5.04080139912755,138.066699627232,12.580842943958));
#82334=CARTESIAN_POINT('Ctrl Pts',(5.03698922707229,138.031690088361,12.6290771750032));
#82335=CARTESIAN_POINT('Ctrl Pts',(5.03531732380184,138.01721773161,12.6504614092324));
#82336=CARTESIAN_POINT('Ctrl Pts',(5.03266041366201,137.995687870691,12.6846424682279));
#82337=CARTESIAN_POINT('Ctrl Pts',(5.03169328023659,137.988145504196,12.697125060604));
#82338=CARTESIAN_POINT('Ctrl Pts',(5.0298432118675,137.97428657834,12.7210545138869));
#82339=CARTESIAN_POINT('Ctrl Pts',(5.02896208102689,137.967925001276,12.7324728443154));
#82340=CARTESIAN_POINT('Ctrl Pts',(5.02692405597387,137.953764085184,12.7589159192927));
#82341=CARTESIAN_POINT('Ctrl Pts',(5.02576274515258,137.946096181072,12.7740073572942));
#82342=CARTESIAN_POINT('Ctrl Pts',(5.02180595820455,137.921326529643,12.8254749058475));
#82343=CARTESIAN_POINT('Ctrl Pts',(5.01896016010826,137.905763816309,12.862556216599));
#82344=CARTESIAN_POINT('Ctrl Pts',(5.01519767867307,137.888031356643,12.9117133153927));
#82345=CARTESIAN_POINT('Ctrl Pts',(5.01432451051326,137.884109697194,12.9231318098902));
#82346=CARTESIAN_POINT('Ctrl Pts',(5.008428959518,137.858915564422,13.00033184331));
#82347=CARTESIAN_POINT('Ctrl Pts',(5.00330320730206,137.843296298042,13.0678131511312));
#82348=CARTESIAN_POINT('Ctrl Pts',(4.996691753016,137.830643370314,13.1579467092443));
#82349=CARTESIAN_POINT('Ctrl Pts',(4.99511456189243,137.828205392505,13.1797021648625));
#82350=CARTESIAN_POINT('Ctrl Pts',(4.99241906058703,137.82503353028,13.2175002153568));
#82351=CARTESIAN_POINT('Ctrl Pts',(4.99129097947808,137.824018718384,13.2335131066865));
#82352=CARTESIAN_POINT('Ctrl Pts',(4.9895913875169,137.822968395752,13.2580067050428));
#82353=CARTESIAN_POINT('Ctrl Pts',(4.9890085287092,137.822696766944,13.2664747451221));
#82354=CARTESIAN_POINT('Ctrl Pts',(4.98792111465327,137.822357571273,13.2824157577345));
#82355=CARTESIAN_POINT('Ctrl Pts',(4.98741558349857,137.822269709671,13.289887550912));
#82356=CARTESIAN_POINT('Ctrl Pts',(4.98615363360918,137.822227583227,13.308679943909));
#82357=CARTESIAN_POINT('Ctrl Pts',(4.98540207172252,137.822365413987,13.3200003207807));
#82358=CARTESIAN_POINT('Ctrl Pts',(4.98228754559904,137.823625123722,13.3673572273729));
#82359=CARTESIAN_POINT('Ctrl Pts',(4.97999250369455,137.826238230008,13.4033375990253));
#82360=CARTESIAN_POINT('Ctrl Pts',(4.97249045344082,137.840368030264,13.5220976898578));
#82361=CARTESIAN_POINT('Ctrl Pts',(4.96743625790818,137.859030271177,13.6037256666642));
#82362=CARTESIAN_POINT('Ctrl Pts',(4.96216799084082,137.886148228708,13.6826608081431));
#82363=CARTESIAN_POINT('',(4.88847248670267,137.822250347659,13.2990950627804));
#82364=CARTESIAN_POINT('Ctrl Pts',(4.86231567683356,137.88614821265,13.6826607614027));
#82365=CARTESIAN_POINT('Ctrl Pts',(4.8645148585283,137.874736790429,13.6494443088179));
#82366=CARTESIAN_POINT('Ctrl Pts',(4.86674140775455,137.864808999366,13.6157110894406));
#82367=CARTESIAN_POINT('Ctrl Pts',(4.87034394071392,137.851480583466,13.5615755602647));
#82368=CARTESIAN_POINT('Ctrl Pts',(4.87168818012219,137.847085384947,13.5414672469751));
#82369=CARTESIAN_POINT('Ctrl Pts',(4.8739525826596,137.840652522983,13.5078345245234));
#82370=CARTESIAN_POINT('Ctrl Pts',(4.87486326623803,137.838319446138,13.494370847295));
#82371=CARTESIAN_POINT('Ctrl Pts',(4.87660826881864,137.83433165814,13.4687120827688));
#82372=CARTESIAN_POINT('Ctrl Pts',(4.87744106128916,137.832632809573,13.456525629891));
#82373=CARTESIAN_POINT('Ctrl Pts',(4.87919781499112,137.829475592632,13.4309538852708));
#82374=CARTESIAN_POINT('Ctrl Pts',(4.88012284173155,137.828055219537,13.417565784355));
#82375=CARTESIAN_POINT('Ctrl Pts',(4.88348366316469,137.823762478546,13.3692159067949));
#82376=CARTESIAN_POINT('Ctrl Pts',(4.88595853238333,137.822223399548,13.334167250912));
#82377=CARTESIAN_POINT('Ctrl Pts',(4.88847248670261,137.822250347659,13.2990950627804));
#82378=CARTESIAN_POINT('Ctrl Pts',(4.88847248670253,137.822250347659,13.2990950627817));
#82379=CARTESIAN_POINT('Ctrl Pts',(4.89548691716877,137.822325538226,13.2012367114737));
#82380=CARTESIAN_POINT('Ctrl Pts',(4.90280164485462,137.834594185474,13.1037919136678));
#82381=CARTESIAN_POINT('Ctrl Pts',(4.91101803388777,137.862807609492,12.9931524352178));
#82382=CARTESIAN_POINT('Ctrl Pts',(4.91218400364322,137.867173579335,12.9774068887808));
#82383=CARTESIAN_POINT('Ctrl Pts',(4.9142518460924,137.875593462271,12.9493242876122));
#82384=CARTESIAN_POINT('Ctrl Pts',(4.91515858947528,137.879526417949,12.936953853555));
#82385=CARTESIAN_POINT('Ctrl Pts',(4.91659894685295,137.886176724171,12.9171750130038));
#82386=CARTESIAN_POINT('Ctrl Pts',(4.91713931866423,137.8887653124,12.9097247885511));
#82387=CARTESIAN_POINT('Ctrl Pts',(4.91822312495569,137.894151730001,12.8947103552642));
#82388=CARTESIAN_POINT('Ctrl Pts',(4.91876635462145,137.896952783002,12.8871477999224));
#82389=CARTESIAN_POINT('Ctrl Pts',(4.92023079385646,137.904773381943,12.8666809331957));
#82390=CARTESIAN_POINT('Ctrl Pts',(4.92114370883561,137.909943313797,12.8538349850063));
#82391=CARTESIAN_POINT('Ctrl Pts',(4.92633665979877,137.940976276048,12.780487924144));
#82392=CARTESIAN_POINT('Ctrl Pts',(4.93039460301909,137.971649482345,12.7221407443561));
#82393=CARTESIAN_POINT('Ctrl Pts',(4.93867632660916,138.043721744807,12.6091454758047));
#82394=CARTESIAN_POINT('Ctrl Pts',(4.94288825183901,138.085327219999,12.5549358029972));
#82395=CARTESIAN_POINT('Ctrl Pts',(4.94876112406876,138.147036562156,12.4875436089103));
#82396=CARTESIAN_POINT('Ctrl Pts',(4.95026787409135,138.163185420687,12.4709202338304));
#82397=CARTESIAN_POINT('Ctrl Pts',(4.95272829058628,138.189965726914,12.4449329434705));
#82398=CARTESIAN_POINT('Ctrl Pts',(4.95366859643321,138.200294511792,12.4352651865165));
#82399=CARTESIAN_POINT('Ctrl Pts',(4.95551064907986,138.220690535582,12.4168524685625));
#82400=CARTESIAN_POINT('Ctrl Pts',(4.95641136289903,138.230737116543,12.4080877877379));
#82401=CARTESIAN_POINT('Ctrl Pts',(4.95858815728105,138.255177390207,12.3874861290406));
#82402=CARTESIAN_POINT('Ctrl Pts',(4.95987074853258,138.26970706829,12.3758168745592));
#82403=CARTESIAN_POINT('Ctrl Pts',(4.96518096151397,138.330349347986,12.3294362889367));
#82404=CARTESIAN_POINT('Ctrl Pts',(4.9693216187203,138.378700522267,12.2977968469521));
#82405=CARTESIAN_POINT('Ctrl Pts',(4.97804710156335,138.483309238536,12.2398316819389));
#82406=CARTESIAN_POINT('Ctrl Pts',(4.98262935600328,138.539729166617,12.2141469177833));
#82407=CARTESIAN_POINT('Ctrl Pts',(4.98863411312278,138.617535407589,12.1858850821486));
#82408=CARTESIAN_POINT('Ctrl Pts',(4.99013683475325,138.637352125695,12.1792779873097));
#82409=CARTESIAN_POINT('Ctrl Pts',(4.99272179291685,138.672193915788,12.1686824334877));
#82410=CARTESIAN_POINT('Ctrl Pts',(4.99381279315654,138.687141562379,12.1644578738543));
#82411=CARTESIAN_POINT('Ctrl Pts',(4.99547108090021,138.710299538721,12.1584049217417));
#82412=CARTESIAN_POINT('Ctrl Pts',(4.99604886287629,138.718452651805,12.1563668501076));
#82413=CARTESIAN_POINT('Ctrl Pts',(4.99713793574227,138.733995002267,12.1526579500413));
#82414=CARTESIAN_POINT('Ctrl Pts',(4.9976500276137,138.741379640292,12.1509708658229));
#82415=CARTESIAN_POINT('Ctrl Pts',(4.9989454030387,138.760240847919,12.1468529067516));
#82416=CARTESIAN_POINT('Ctrl Pts',(4.99972331713554,138.771738778229,12.1445219558062));
#82417=CARTESIAN_POINT('Ctrl Pts',(5.00319414739933,138.823703159234,12.1347933164909));
#82418=CARTESIAN_POINT('Ctrl Pts',(5.00579797082261,138.864509372924,12.1293462570487));
#82419=CARTESIAN_POINT('Ctrl Pts',(5.01279583783542,138.97622235101,12.1203556606684));
#82420=CARTESIAN_POINT('Ctrl Pts',(5.01711398169721,139.047292718552,12.1210641516306));
#82421=CARTESIAN_POINT('Ctrl Pts',(5.02329689418963,139.14526284541,12.1309183799633));
#82422=CARTESIAN_POINT('Ctrl Pts',(5.02504297554812,139.17255106472,12.1346334868185));
#82423=CARTESIAN_POINT('Ctrl Pts',(5.02825541464193,139.221732904367,12.1430945677038));
#82424=CARTESIAN_POINT('Ctrl Pts',(5.02971217104078,139.243669192754,12.1475153448818));
#82425=CARTESIAN_POINT('Ctrl Pts',(5.03211206445923,139.27910134506,12.1557127113435));
#82426=CARTESIAN_POINT('Ctrl Pts',(5.03304308536084,139.292679658213,12.1591101941476));
#82427=CARTESIAN_POINT('Ctrl Pts',(5.03487144783709,139.318997470438,12.1661960063663));
#82428=CARTESIAN_POINT('Ctrl Pts',(5.0357678511595,139.331741607803,12.1698591402838));
#82429=CARTESIAN_POINT('Ctrl Pts',(5.03796686386794,139.362603059582,12.1792968291271));
#82430=CARTESIAN_POINT('Ctrl Pts',(5.03927661799051,139.380647072588,12.18529631354));
#82431=CARTESIAN_POINT('Ctrl Pts',(5.04728537750681,139.488893427004,12.22422200111));
#82432=CARTESIAN_POINT('Ctrl Pts',(5.05433785458231,139.57492257982,12.267637470714));
#82433=CARTESIAN_POINT('Ctrl Pts',(5.06388572184568,139.683114468292,12.3399910098731));
#82434=CARTESIAN_POINT('Ctrl Pts',(5.06638171421552,139.710679569353,12.3602141536061));
#82435=CARTESIAN_POINT('Ctrl Pts',(5.06993176157421,139.749240021854,12.3911722778309));
#82436=CARTESIAN_POINT('Ctrl Pts',(5.07101955893555,139.76096592023,12.4009675463331));
#82437=CARTESIAN_POINT('Ctrl Pts',(5.07296449655076,139.78181860446,12.4190872997647));
#82438=CARTESIAN_POINT('Ctrl Pts',(5.07382573824142,139.791011291121,12.4273324322755));
#82439=CARTESIAN_POINT('Ctrl Pts',(5.0752123483365,139.805769389134,12.4409941743897));
#82440=CARTESIAN_POINT('Ctrl Pts',(5.07574363308372,139.811413736149,12.4463237858243));
#82441=CARTESIAN_POINT('Ctrl Pts',(5.07682923786249,139.822933510383,12.4574187024086));
#82442=CARTESIAN_POINT('Ctrl Pts',(5.07738305432876,139.828801935657,12.4631904833319));
#82443=CARTESIAN_POINT('Ctrl Pts',(5.07891143861902,139.844955927516,12.47941510213));
#82444=CARTESIAN_POINT('Ctrl Pts',(5.07987644302062,139.855107871583,12.4899995863565));
#82445=CARTESIAN_POINT('Ctrl Pts',(5.08454913630464,139.903852919213,12.5427597075515));
#82446=CARTESIAN_POINT('Ctrl Pts',(5.08809658011121,139.939541679852,12.5875213628603));
#82447=CARTESIAN_POINT('Ctrl Pts',(5.0950770509931,140.003304030637,12.6806629648027));
#82448=CARTESIAN_POINT('Ctrl Pts',(5.09850278284048,140.031466495772,12.7287961430419));
#82449=CARTESIAN_POINT('Ctrl Pts',(5.10357264011236,140.067024079663,12.8008386589504));
#82450=CARTESIAN_POINT('Ctrl Pts',(5.10514332159243,140.077234741274,12.8232740527716));
#82451=CARTESIAN_POINT('Ctrl Pts',(5.10806943810135,140.094693040769,12.8650648737518));
#82452=CARTESIAN_POINT('Ctrl Pts',(5.10941793304798,140.102149530959,12.8843225465763));
#82453=CARTESIAN_POINT('Ctrl Pts',(5.11168743209757,140.113696748738,12.9166442256051));
#82454=CARTESIAN_POINT('Ctrl Pts',(5.11259886091066,140.118072998512,12.9296017801158));
#82455=CARTESIAN_POINT('Ctrl Pts',(5.11443544278927,140.126366286183,12.9556447325436));
#82456=CARTESIAN_POINT('Ctrl Pts',(5.11536043223832,140.130283295829,12.9687278992948));
#82457=CARTESIAN_POINT('Ctrl Pts',(5.11769542107772,140.139519865744,13.0016521727685));
#82458=CARTESIAN_POINT('Ctrl Pts',(5.11911447977523,140.144549317113,13.0215691848301));
#82459=CARTESIAN_POINT('Ctrl Pts',(5.12648317879188,140.167686637851,13.1244589837867));
#82460=CARTESIAN_POINT('Ctrl Pts',(5.13269443692922,140.177299446669,13.2090708636872));
#82461=CARTESIAN_POINT('Ctrl Pts',(5.1418080795938,140.177935397526,13.3331563898544));
#82462=CARTESIAN_POINT('Ctrl Pts',(5.14468163177423,140.176179790566,13.3723363073986));
#82463=CARTESIAN_POINT('Ctrl Pts',(5.14869329247567,140.170910844511,13.4278126584891));
#82464=CARTESIAN_POINT('Ctrl Pts',(5.14987345516513,140.169001654566,13.4442340748865));
#82465=CARTESIAN_POINT('Ctrl Pts',(5.15196349165263,140.164961933777,13.4735804065548));
#82466=CARTESIAN_POINT('Ctrl Pts',(5.15287838148664,140.162960326218,13.4865201874951));
#82467=CARTESIAN_POINT('Ctrl Pts',(5.1543283981841,140.159403975766,13.5072197935339));
#82468=CARTESIAN_POINT('Ctrl Pts',(5.1548704356357,140.157986145424,13.5150016734491));
#82469=CARTESIAN_POINT('Ctrl Pts',(5.15595419496341,140.154969608166,13.5306618187313));
#82470=CARTESIAN_POINT('Ctrl Pts',(5.1564957613229,140.153368438275,13.5385391489142));
#82471=CARTESIAN_POINT('Ctrl Pts',(5.15795021078446,140.148816766828,13.5598139238433));
#82472=CARTESIAN_POINT('Ctrl Pts',(5.15885499084909,140.145712552598,13.5731776450399));
#82473=CARTESIAN_POINT('Ctrl Pts',(5.16420095360714,140.125776584273,13.6526735253499));
#82474=CARTESIAN_POINT('Ctrl Pts',(5.1684015065631,140.103454654598,13.7173027914359));
#82475=CARTESIAN_POINT('Ctrl Pts',(5.17709537390135,140.046156106398,13.8458022633954));
#82476=CARTESIAN_POINT('Ctrl Pts',(5.18157683249815,140.010616835694,13.9090934417462));
#82477=CARTESIAN_POINT('Ctrl Pts',(5.18755591983171,139.958151133315,13.9851571965144));
#82478=CARTESIAN_POINT('Ctrl Pts',(5.18886197794427,139.94639490831,14.0013063377811));
#82479=CARTESIAN_POINT('Ctrl Pts',(5.19108079996645,139.925980315064,14.027900586971));
#82480=CARTESIAN_POINT('Ctrl Pts',(5.19198493013701,139.917541601826,14.0385094388955));
#82481=CARTESIAN_POINT('Ctrl Pts',(5.19382371495782,139.900152883245,14.0596117391659));
#82482=CARTESIAN_POINT('Ctrl Pts',(5.1947584816693,139.891197933404,14.0700983202328));
#82483=CARTESIAN_POINT('Ctrl Pts',(5.19715427000131,139.867969545495,14.0963517898346));
#82484=CARTESIAN_POINT('Ctrl Pts',(5.19862537963258,139.853449903096,14.1118931369253));
#82485=CARTESIAN_POINT('Ctrl Pts',(5.20552403999925,139.78422887007,14.1820755449686));
#82486=CARTESIAN_POINT('Ctrl Pts',(5.21116027523093,139.724659602014,14.2316314206108));
#82487=CARTESIAN_POINT('Ctrl Pts',(5.22132278042843,139.610124934469,14.309243050884));
#82488=CARTESIAN_POINT('Ctrl Pts',(5.22581329326415,139.556981271851,14.3395177144443));
#82489=CARTESIAN_POINT('Ctrl Pts',(5.23108082421731,139.489510191581,14.3712876033704));
#82490=CARTESIAN_POINT('Ctrl Pts',(5.2320252411473,139.477196293732,14.3768291847769));
#82491=CARTESIAN_POINT('Ctrl Pts',(5.23351032439833,139.457444512307,14.3853126167136));
#82492=CARTESIAN_POINT('Ctrl Pts',(5.23405846243536,139.4500676439,14.3883924307198));
#82493=CARTESIAN_POINT('Ctrl Pts',(5.23507673492042,139.436189982178,14.3940210716225));
#82494=CARTESIAN_POINT('Ctrl Pts',(5.23554792879041,139.429696842429,14.3965876322717));
#82495=CARTESIAN_POINT('Ctrl Pts',(5.23683717483486,139.411746604088,14.4034989470134));
#82496=CARTESIAN_POINT('Ctrl Pts',(5.23764847261467,139.400243568925,14.4077230281826));
#82497=CARTESIAN_POINT('Ctrl Pts',(5.24246520709872,139.330860070976,14.4319796486134));
#82498=CARTESIAN_POINT('Ctrl Pts',(5.24626757305046,139.271547788967,14.4476541219496));
#82499=CARTESIAN_POINT('Ctrl Pts',(5.25351799155964,139.156217720196,14.468684571268));
#82500=CARTESIAN_POINT('Ctrl Pts',(5.25695968664792,139.100512193876,14.4747870199149));
#82501=CARTESIAN_POINT('Ctrl Pts',(5.26204983975474,139.019899740251,14.4778409781601));
#82502=CARTESIAN_POINT('Ctrl Pts',(5.2636241456482,138.995191027162,14.4779992055164));
#82503=CARTESIAN_POINT('Ctrl Pts',(5.26655622101752,138.949818475238,14.4768622413893));
#82504=CARTESIAN_POINT('Ctrl Pts',(5.26790699961545,138.929158572957,14.4757994424078));
#82505=CARTESIAN_POINT('Ctrl Pts',(5.27017923438846,138.894896966168,14.4731306963648));
#82506=CARTESIAN_POINT('Ctrl Pts',(5.27109106375583,138.881275661597,14.4718305266946));
#82507=CARTESIAN_POINT('Ctrl Pts',(5.27292758330604,138.854117010114,14.4687598289257));
#82508=CARTESIAN_POINT('Ctrl Pts',(5.27385209567943,138.840581659259,14.4669906382592));
#82509=CARTESIAN_POINT('Ctrl Pts',(5.27618409523374,138.806798640559,14.4619762121945));
#82510=CARTESIAN_POINT('Ctrl Pts',(5.27760059194484,138.786599950158,14.4584367958131));
#82511=CARTESIAN_POINT('Ctrl Pts',(5.28498690746441,138.682978640334,14.4374772997715));
#82512=CARTESIAN_POINT('Ctrl Pts',(5.29122057227595,138.601545557684,14.4115693959577));
#82513=CARTESIAN_POINT('Ctrl Pts',(5.30034502742721,138.48792490543,14.3613193499744));
#82514=CARTESIAN_POINT('Ctrl Pts',(5.3032075404861,138.453020919967,14.3437594762598));
#82515=CARTESIAN_POINT('Ctrl Pts',(5.30720583402013,138.404704164047,14.3163611549259));
#82516=CARTESIAN_POINT('Ctrl Pts',(5.30838342192403,138.390527780937,14.3079240044388));
#82517=CARTESIAN_POINT('Ctrl Pts',(5.31046943494251,138.365442821813,14.2922716950244));
#82518=CARTESIAN_POINT('Ctrl Pts',(5.31138284959304,138.354468385578,14.2851674475823));
#82519=CARTESIAN_POINT('Ctrl Pts',(5.31283111679029,138.337050207783,14.2734757979603));
#82520=CARTESIAN_POINT('Ctrl Pts',(5.31337285220417,138.330530709874,14.2690038372454));
#82521=CARTESIAN_POINT('Ctrl Pts',(5.31445661808999,138.317470303601,14.2598504882824));
#82522=CARTESIAN_POINT('Ctrl Pts',(5.31499848416948,138.310931361057,14.2551670883812));
#82523=CARTESIAN_POINT('Ctrl Pts',(5.31645472452214,138.293352321636,14.2423019289567));
#82524=CARTESIAN_POINT('Ctrl Pts',(5.31736096164767,138.282406241601,14.2339930968185));
#82525=CARTESIAN_POINT('Ctrl Pts',(5.32266653879621,138.218484935483,14.1836850546494));
#82526=CARTESIAN_POINT('Ctrl Pts',(5.32683006210891,138.169054047073,14.1373745306261));
#82527=CARTESIAN_POINT('Ctrl Pts',(5.33560138245444,138.074191093655,14.031777369083));
#82528=CARTESIAN_POINT('Ctrl Pts',(5.34019818028491,138.029868043393,13.9719096856994));
#82529=CARTESIAN_POINT('Ctrl Pts',(5.34627003764482,137.981472087225,13.8916686045324));
#82530=CARTESIAN_POINT('Ctrl Pts',(5.34753915001645,137.971872167549,13.8748251356476));
#82531=CARTESIAN_POINT('Ctrl Pts',(5.34971417390312,137.956321207567,13.8459035183746));
#82532=CARTESIAN_POINT('Ctrl Pts',(5.35061224843461,137.95015346722,13.8339459760118));
#82533=CARTESIAN_POINT('Ctrl Pts',(5.35234354011832,137.938753398529,13.810882918818));
#82534=CARTESIAN_POINT('Ctrl Pts',(5.35317542956792,137.93348718595,13.7997960618861));
#82535=CARTESIAN_POINT('Ctrl Pts',(5.35540713930006,137.919925425752,13.7700539946723));
#82536=CARTESIAN_POINT('Ctrl Pts',(5.35681726335248,137.911940384338,13.7512627016996));
#82537=CARTESIAN_POINT('Ctrl Pts',(5.35947526120786,137.897974245769,13.7158670586819));
#82538=CARTESIAN_POINT('Ctrl Pts',(5.36071819853113,137.891873122424,13.6993248713083));
#82539=CARTESIAN_POINT('Ctrl Pts',(5.36197089565136,137.88614821265,13.6826607614027));
#82540=CARTESIAN_POINT('Origin',(1.13913288526384,139.,13.3));
#82541=CARTESIAN_POINT('',(5.96182583603507,137.88614821265,13.6826607614027));
#82542=CARTESIAN_POINT('',(5.8638006232474,137.886148212564,13.6826607611511));
#82543=CARTESIAN_POINT('',(1.13913288526384,137.88614821265,13.6826607614027));
#82544=CARTESIAN_POINT('Ctrl Pts',(5.96182583603505,137.88614821265,13.6826607614027));
#82545=CARTESIAN_POINT('Ctrl Pts',(5.96011823121893,137.893737617578,13.7047520576529));
#82546=CARTESIAN_POINT('Ctrl Pts',(5.95840141063008,137.90198616988,13.7266232135534));
#82547=CARTESIAN_POINT('Ctrl Pts',(5.95211510907587,137.934534674042,13.8057074043303));
#82548=CARTESIAN_POINT('Ctrl Pts',(5.9475447436074,137.96269723102,13.8612135973465));
#82549=CARTESIAN_POINT('Ctrl Pts',(5.94228481536763,138.001629159891,13.9249055316043));
#82550=CARTESIAN_POINT('Ctrl Pts',(5.94141243344031,138.008316912279,13.9354651393033));
#82551=CARTESIAN_POINT('Ctrl Pts',(5.94001680258528,138.019411871242,13.9523816028852));
#82552=CARTESIAN_POINT('Ctrl Pts',(5.93948734669202,138.023715684227,13.9588048129372));
#82553=CARTESIAN_POINT('Ctrl Pts',(5.93841366855325,138.032644380719,13.9718507291547));
#82554=CARTESIAN_POINT('Ctrl Pts',(5.93786980837908,138.037274688495,13.9784690712705));
#82555=CARTESIAN_POINT('Ctrl Pts',(5.93639078171179,138.050150845936,13.9964763656915));
#82556=CARTESIAN_POINT('Ctrl Pts',(5.93546426459298,138.058533394493,14.0077664989763));
#82557=CARTESIAN_POINT('Ctrl Pts',(5.9303590919216,138.106358145992,14.0698260967524));
#82558=CARTESIAN_POINT('Ctrl Pts',(5.92639031211371,138.149707998658,14.1174554577033));
#82559=CARTESIAN_POINT('Ctrl Pts',(5.91921569174844,138.234617431066,14.1966426184107));
#82560=CARTESIAN_POINT('Ctrl Pts',(5.91601972492253,138.274789295956,14.2294339716529));
#82561=CARTESIAN_POINT('Ctrl Pts',(5.91124512842704,138.336318920303,14.2732345976469));
#82562=CARTESIAN_POINT('Ctrl Pts',(5.90973019464238,138.356061147215,14.2864080327878));
#82563=CARTESIAN_POINT('Ctrl Pts',(5.90689712771635,138.39320825991,14.3096046499102));
#82564=CARTESIAN_POINT('Ctrl Pts',(5.90558519653706,138.410497602901,14.3197963578745));
#82565=CARTESIAN_POINT('Ctrl Pts',(5.9033626306518,138.439860043723,14.3361086747282));
#82566=CARTESIAN_POINT('Ctrl Pts',(5.90246079971189,138.45179383174,14.3424720273424));
#82567=CARTESIAN_POINT('Ctrl Pts',(5.90063208098384,138.47601249583,14.3548550818232));
#82568=CARTESIAN_POINT('Ctrl Pts',(5.89970516694265,138.488297933249,14.3608690379197));
#82569=CARTESIAN_POINT('Ctrl Pts',(5.89734161949195,138.519631265975,14.3755364082752));
#82570=CARTESIAN_POINT('Ctrl Pts',(5.89589535788382,138.538809453353,14.383898458643));
#82571=CARTESIAN_POINT('Ctrl Pts',(5.88879460938716,138.63293656073,14.4219892592371));
#82572=CARTESIAN_POINT('Ctrl Pts',(5.88290966751907,138.710570835203,14.4444746595592));
#82573=CARTESIAN_POINT('Ctrl Pts',(5.87396041223407,138.830491382721,14.4662184857584));
#82574=CARTESIAN_POINT('Ctrl Pts',(5.87093113828985,138.871465522935,14.4714426660526));
#82575=CARTESIAN_POINT('Ctrl Pts',(5.86673321892935,138.929575724571,14.4757653670297));
#82576=CARTESIAN_POINT('Ctrl Pts',(5.86551913838495,138.946546686428,14.4766590750894));
#82577=CARTESIAN_POINT('Ctrl Pts',(5.86337698717866,138.976875814769,14.4775986440174));
#82578=CARTESIAN_POINT('Ctrl Pts',(5.86244354722315,138.99022654906,14.4777851297341));
#82579=CARTESIAN_POINT('Ctrl Pts',(5.86097283727908,139.011520787886,14.4777204330298));
#82580=CARTESIAN_POINT('Ctrl Pts',(5.86042830871534,139.019463170119,14.4776159565997));
#82581=CARTESIAN_POINT('Ctrl Pts',(5.85934958939536,139.035325980885,14.4772467568723));
#82582=CARTESIAN_POINT('Ctrl Pts',(5.85881541382726,139.04324599714,14.4769824314348));
#82583=CARTESIAN_POINT('Ctrl Pts',(5.85739605001381,139.064444022689,14.4760606910822));
#82584=CARTESIAN_POINT('Ctrl Pts',(5.8565183556189,139.077714997452,14.4752583533737));
#82585=CARTESIAN_POINT('Ctrl Pts',(5.85089284080241,139.163593226909,14.4686051832654));
#82586=CARTESIAN_POINT('Ctrl Pts',(5.84642396385226,139.235547158018,14.4562530173298));
#82587=CARTESIAN_POINT('Ctrl Pts',(5.83900115377145,139.351512807176,14.4250619092679));
#82588=CARTESIAN_POINT('Ctrl Pts',(5.83607563632052,139.396338858637,14.4100633690781));
#82589=CARTESIAN_POINT('Ctrl Pts',(5.83165195637274,139.461091345754,14.3839741643022));
#82590=CARTESIAN_POINT('Ctrl Pts',(5.83020674910058,139.481793247242,14.3749327386346));
#82591=CARTESIAN_POINT('Ctrl Pts',(5.82748953566476,139.519722021184,14.3570517580433));
#82592=CARTESIAN_POINT('Ctrl Pts',(5.82622284606153,139.537015685281,14.3483718245154));
#82593=CARTESIAN_POINT('Ctrl Pts',(5.82405458779701,139.565902199651,14.3329709793861));
#82594=CARTESIAN_POINT('Ctrl Pts',(5.82316085990642,139.577608733563,14.3264708810573));
#82595=CARTESIAN_POINT('Ctrl Pts',(5.82143998438085,139.599752720506,14.3136765899579));
#82596=CARTESIAN_POINT('Ctrl Pts',(5.82061417845938,139.610208321068,14.3074171629726));
#82597=CARTESIAN_POINT('Ctrl Pts',(5.8184045395303,139.637721463053,14.2903604840786));
#82598=CARTESIAN_POINT('Ctrl Pts',(5.81701068083554,139.654601059972,14.2792854116494));
#82599=CARTESIAN_POINT('Ctrl Pts',(5.80949571061924,139.743042536861,14.2179485420254));
#82600=CARTESIAN_POINT('Ctrl Pts',(5.80309361467179,139.809113398461,14.1602744838695));
#82601=CARTESIAN_POINT('Ctrl Pts',(5.79388054169744,139.89388896505,14.0677921588766));
#82602=CARTESIAN_POINT('Ctrl Pts',(5.79109352662553,139.918222608693,14.0385186581146));
#82603=CARTESIAN_POINT('Ctrl Pts',(5.7871885583161,139.950856256386,13.9951480957466));
#82604=CARTESIAN_POINT('Ctrl Pts',(5.78603040691135,139.960346211489,13.9819777872256));
#82605=CARTESIAN_POINT('Ctrl Pts',(5.78397579042687,139.976885930995,13.9579934684279));
#82606=CARTESIAN_POINT('Ctrl Pts',(5.78307451665183,139.984035879364,13.9472518438628));
#82607=CARTESIAN_POINT('Ctrl Pts',(5.78164272385419,139.995244693554,13.9297972152336));
#82608=CARTESIAN_POINT('Ctrl Pts',(5.78110552454486,139.999415368156,13.9231576565738));
#82609=CARTESIAN_POINT('Ctrl Pts',(5.78002913189269,140.007707355316,13.9096597055595));
#82610=CARTESIAN_POINT('Ctrl Pts',(5.77949012598819,140.011825689545,13.9028000115705));
#82611=CARTESIAN_POINT('Ctrl Pts',(5.77803953038277,140.022804837136,13.8840830193521));
#82612=CARTESIAN_POINT('Ctrl Pts',(5.7771360497345,140.029529426851,13.8721467535701));
#82613=CARTESIAN_POINT('Ctrl Pts',(5.77182655191937,140.068240233469,13.8005408595235));
#82614=CARTESIAN_POINT('Ctrl Pts',(5.76765739848215,140.095244972066,13.7383138376469));
#82615=CARTESIAN_POINT('Ctrl Pts',(5.76038419398895,140.13263494729,13.626699489664));
#82616=CARTESIAN_POINT('Ctrl Pts',(5.75729523096722,140.145480113471,13.5783332550406));
#82617=CARTESIAN_POINT('Ctrl Pts',(5.7526595334823,140.159745071315,13.5064662959409));
#82618=CARTESIAN_POINT('Ctrl Pts',(5.75117220086569,140.163599090439,13.483504819973));
#82619=CARTESIAN_POINT('Ctrl Pts',(5.74838539174638,140.169464360754,13.4408521229527));
#82620=CARTESIAN_POINT('Ctrl Pts',(5.74709177561977,140.17166456223,13.4211952596649));
#82621=CARTESIAN_POINT('Ctrl Pts',(5.74489229785851,140.174528094547,13.38808980171));
#82622=CARTESIAN_POINT('Ctrl Pts',(5.74399487414104,140.175457664827,13.3746680040289));
#82623=CARTESIAN_POINT('Ctrl Pts',(5.74216870547368,140.176869511108,13.3475497109395));
#82624=CARTESIAN_POINT('Ctrl Pts',(5.74123983092785,140.177343043011,13.333854875685));
#82625=CARTESIAN_POINT('Ctrl Pts',(5.73885796269891,140.177939490723,13.2990074426091));
#82626=CARTESIAN_POINT('Ctrl Pts',(5.73739496875569,140.177731684799,13.2778548660421));
#82627=CARTESIAN_POINT('Ctrl Pts',(5.73044158027849,140.174079960356,13.1785488992596));
#82628=CARTESIAN_POINT('Ctrl Pts',(5.72473632171545,140.163424968954,13.1008699019074));
#82629=CARTESIAN_POINT('Ctrl Pts',(5.71443334966285,140.130656661637,12.9644988971715));
#82630=CARTESIAN_POINT('Ctrl Pts',(5.70987162177614,140.111412196429,12.9053992202477));
#82631=CARTESIAN_POINT('Ctrl Pts',(5.70461132926718,140.082766585667,12.8364591300526));
#82632=CARTESIAN_POINT('Ctrl Pts',(5.70373238358566,140.077748563387,12.8249087627956));
#82633=CARTESIAN_POINT('Ctrl Pts',(5.70232730544245,140.069334244965,12.8063606836711));
#82634=CARTESIAN_POINT('Ctrl Pts',(5.70179489757434,140.066052305493,12.7993124767048));
#82635=CARTESIAN_POINT('Ctrl Pts',(5.70071822097289,140.059218390662,12.7850080414531));
#82636=CARTESIAN_POINT('Ctrl Pts',(5.7001742815189,140.055661111946,12.77775490153));
#82637=CARTESIAN_POINT('Ctrl Pts',(5.698694872363,140.045706583019,12.7579754463378));
#82638=CARTESIAN_POINT('Ctrl Pts',(5.69776805799494,140.039158930058,12.7455258026106));
#82639=CARTESIAN_POINT('Ctrl Pts',(5.6926646769622,140.001465363884,12.6768699253258));
#82640=CARTESIAN_POINT('Ctrl Pts',(5.68869771561106,139.965979740144,12.6231624762119));
#82641=CARTESIAN_POINT('Ctrl Pts',(5.68001394235995,139.879191715745,12.5126428405012));
#82642=CARTESIAN_POINT('Ctrl Pts',(5.67530830155633,139.826390953846,12.4573934737635));
#82643=CARTESIAN_POINT('Ctrl Pts',(5.66909597460168,139.753685133914,12.3947693477996));
#82644=CARTESIAN_POINT('Ctrl Pts',(5.66780612502901,139.738426009796,12.3822795800316));
#82645=CARTESIAN_POINT('Ctrl Pts',(5.66561061823598,139.712242373337,12.3619238963418));
#82646=CARTESIAN_POINT('Ctrl Pts',(5.66471330389447,139.701483214879,12.3538513602601));
#82647=CARTESIAN_POINT('Ctrl Pts',(5.66288526993955,139.679466075503,12.337914014108));
#82648=CARTESIAN_POINT('Ctrl Pts',(5.6619543873137,139.668204104716,12.3300583323489));
#82649=CARTESIAN_POINT('Ctrl Pts',(5.65956262261753,139.639157815825,12.3105433366179));
#82650=CARTESIAN_POINT('Ctrl Pts',(5.65809159474552,139.621191026125,12.2991659432353));
#82651=CARTESIAN_POINT('Ctrl Pts',(5.65125654899255,139.537297079988,12.2491698781763));
#82652=CARTESIAN_POINT('Ctrl Pts',(5.64568953666921,139.46802680662,12.2165427676249));
#82653=CARTESIAN_POINT('Ctrl Pts',(5.63553434896756,139.33781508253,12.1700415315658));
#82654=CARTESIAN_POINT('Ctrl Pts',(5.63098134508052,139.277977521562,12.153852133142));
#82655=CARTESIAN_POINT('Ctrl Pts',(5.62565780568099,139.203897184205,12.1399557943558));
#82656=CARTESIAN_POINT('Ctrl Pts',(5.62471531338484,139.190611436747,12.1376988600848));
#82657=CARTESIAN_POINT('Ctrl Pts',(5.62323453114311,139.169421700438,12.1344723587735));
#82658=CARTESIAN_POINT('Ctrl Pts',(5.62268878413256,139.161541974721,12.1333541262194));
#82659=CARTESIAN_POINT('Ctrl Pts',(5.62161145564149,139.145834716709,12.1312872663778));
#82660=CARTESIAN_POINT('Ctrl Pts',(5.62107983316652,139.138007814677,12.1303371983461));
#82661=CARTESIAN_POINT('Ctrl Pts',(5.61967445894418,139.11713379565,12.1280158594219));
#82662=CARTESIAN_POINT('Ctrl Pts',(5.61880795836829,139.104071892936,12.1267838099828));
#82663=CARTESIAN_POINT('Ctrl Pts',(5.61309025665132,139.016831634641,12.1200235325787));
#82664=CARTESIAN_POINT('Ctrl Pts',(5.6085322527808,138.942284339824,12.1213144954013));
#82665=CARTESIAN_POINT('Ctrl Pts',(5.59978100013999,138.80159967119,12.1371396193206));
#82666=CARTESIAN_POINT('Ctrl Pts',(5.59561024351538,138.735621860578,12.1503436133796));
#82667=CARTESIAN_POINT('Ctrl Pts',(5.58996977868262,138.651902036324,12.1746893929856));
#82668=CARTESIAN_POINT('Ctrl Pts',(5.58866041278935,138.632818138689,12.1807709982124));
#82669=CARTESIAN_POINT('Ctrl Pts',(5.58644177020448,138.601142089389,12.1917627615633));
#82670=CARTESIAN_POINT('Ctrl Pts',(5.58554126267944,138.588462294832,12.1964085443104));
#82671=CARTESIAN_POINT('Ctrl Pts',(5.58371499454321,138.563121207182,12.2061907819345));
#82672=CARTESIAN_POINT('Ctrl Pts',(5.58278920357777,138.550463853287,12.2113315883345));
#82673=CARTESIAN_POINT('Ctrl Pts',(5.5804284017653,138.518679587267,12.2248896189564));
#82674=CARTESIAN_POINT('Ctrl Pts',(5.57898376739546,138.499682673687,12.2335975679513));
#82675=CARTESIAN_POINT('Ctrl Pts',(5.57184231958782,138.408016573631,12.2786046844823));
#82676=CARTESIAN_POINT('Ctrl Pts',(5.5659105059868,138.339014820911,12.3218449599085));
#82677=CARTESIAN_POINT('Ctrl Pts',(5.55563458038244,138.228767722104,12.407957155959));
#82678=CARTESIAN_POINT('Ctrl Pts',(5.55132669574459,138.185275319068,12.4474951161085));
#82679=CARTESIAN_POINT('Ctrl Pts',(5.54626578317972,138.135944832477,12.4995790662128));
#82680=CARTESIAN_POINT('Ctrl Pts',(5.54535485810406,138.127137740602,12.5091924915245));
#82681=CARTESIAN_POINT('Ctrl Pts',(5.54391168352428,138.113274769112,12.5248385263968));
#82682=CARTESIAN_POINT('Ctrl Pts',(5.54337257195953,138.108116800488,12.5307787613485));
#82683=CARTESIAN_POINT('Ctrl Pts',(5.54229607643484,138.097851869321,12.5428425676033));
#82684=CARTESIAN_POINT('Ctrl Pts',(5.54175882467009,138.092746811157,12.5489671859373));
#82685=CARTESIAN_POINT('Ctrl Pts',(5.5403194320846,138.079132384123,12.5656420535104));
#82686=CARTESIAN_POINT('Ctrl Pts',(5.53942517943703,138.070742021189,12.5762884502685));
#82687=CARTESIAN_POINT('Ctrl Pts',(5.53395895523541,138.020036812751,12.6429637024989));
#82688=CARTESIAN_POINT('Ctrl Pts',(5.52964353645112,137.982613808703,12.7025451332079));
#82689=CARTESIAN_POINT('Ctrl Pts',(5.52086388672032,137.918088483729,12.8291234519681));
#82690=CARTESIAN_POINT('Ctrl Pts',(5.51641309961538,137.891387041568,12.8959789339011));
#82691=CARTESIAN_POINT('Ctrl Pts',(5.5105006318927,137.865415890983,12.9834698235924));
#82692=CARTESIAN_POINT('Ctrl Pts',(5.50922904837508,137.860349560329,13.0022261634588));
#82693=CARTESIAN_POINT('Ctrl Pts',(5.50705537625462,137.852576937392,13.0341149227774));
#82694=CARTESIAN_POINT('Ctrl Pts',(5.50616124339647,137.849626714765,13.0471841809013));
#82695=CARTESIAN_POINT('Ctrl Pts',(5.50444158497547,137.844424697014,13.0722090358037));
#82696=CARTESIAN_POINT('Ctrl Pts',(5.50361743191009,137.842133926922,13.0841548200102));
#82697=CARTESIAN_POINT('Ctrl Pts',(5.50141720173685,137.836553502458,13.1159066498313));
#82698=CARTESIAN_POINT('Ctrl Pts',(5.50003124455126,137.833584705413,13.1357642290293));
#82699=CARTESIAN_POINT('Ctrl Pts',(5.49247408934862,137.820319170475,13.2432094903203));
#82700=CARTESIAN_POINT('Ctrl Pts',(5.48601590191447,137.819379492195,13.3316551585687));
#82701=CARTESIAN_POINT('Ctrl Pts',(5.47677675407356,137.832131187445,13.4568321164502));
#82702=CARTESIAN_POINT('Ctrl Pts',(5.47401798799671,137.837744278816,13.494102544814));
#82703=CARTESIAN_POINT('Ctrl Pts',(5.47014753393553,137.848299941047,13.5468652462176));
#82704=CARTESIAN_POINT('Ctrl Pts',(5.46899627388069,137.85179068066,13.5626230886353));
#82705=CARTESIAN_POINT('Ctrl Pts',(5.46695252278782,137.85863990202,13.5907872258973));
#82706=CARTESIAN_POINT('Ctrl Pts',(5.46605529100999,137.861879635933,13.6032196482534));
#82707=CARTESIAN_POINT('Ctrl Pts',(5.46462838066217,137.867419868687,13.6231386417839));
#82708=CARTESIAN_POINT('Ctrl Pts',(5.46409209458997,137.869592658602,13.6306593250235));
#82709=CARTESIAN_POINT('Ctrl Pts',(5.46301552798629,137.874142244438,13.6458376060974));
#82710=CARTESIAN_POINT('Ctrl Pts',(5.46247546231711,137.876522553658,13.6534936669756));
#82711=CARTESIAN_POINT('Ctrl Pts',(5.46143383519277,137.881300782265,13.6683264361376));
#82712=CARTESIAN_POINT('Ctrl Pts',(5.46093185542975,137.883689981072,13.6755053226633));
#82713=CARTESIAN_POINT('Ctrl Pts',(5.46043320712869,137.886148212658,13.6826607614259));
#82714=CARTESIAN_POINT('Ctrl Pts',(5.36197089565136,137.88614821265,13.6826607614027));
#82715=CARTESIAN_POINT('Ctrl Pts',(5.36682188552324,137.863978863903,13.6181300563578));
#82716=CARTESIAN_POINT('Ctrl Pts',(5.37182980528586,137.847451361312,13.5517717427999));
#82717=CARTESIAN_POINT('Ctrl Pts',(5.38086387332755,137.828198566571,13.4302761780259));
#82718=CARTESIAN_POINT('Ctrl Pts',(5.38487227722085,137.823410219707,13.3756838698077));
#82719=CARTESIAN_POINT('Ctrl Pts',(5.38966919771979,137.822201126917,13.3077301872115));
#82720=CARTESIAN_POINT('Ctrl Pts',(5.39059360907863,137.822188565055,13.2945043702931));
#82721=CARTESIAN_POINT('Ctrl Pts',(5.3920549261728,137.822524919861,13.2733450876296));
#82722=CARTESIAN_POINT('Ctrl Pts',(5.39259892193165,137.822731275235,13.2654108603999));
#82723=CARTESIAN_POINT('Ctrl Pts',(5.39368271419258,137.823306963659,13.2494757895673));
#82724=CARTESIAN_POINT('Ctrl Pts',(5.3942224114107,137.823677730356,13.2414754322686));
#82725=CARTESIAN_POINT('Ctrl Pts',(5.39566565615187,137.824896799688,13.2199262831634));
#82726=CARTESIAN_POINT('Ctrl Pts',(5.39656131327966,137.825897805532,13.2063869266585));
#82727=CARTESIAN_POINT('Ctrl Pts',(5.40203800174505,137.833532014225,13.1228092222845));
#82728=CARTESIAN_POINT('Ctrl Pts',(5.4063614819717,137.84619633229,13.0534565422798));
#82729=CARTESIAN_POINT('Ctrl Pts',(5.41503137365049,137.883643820636,12.9182483767596));
#82730=CARTESIAN_POINT('Ctrl Pts',(5.41936322646518,137.908272466742,12.8526578414945));
#82731=CARTESIAN_POINT('Ctrl Pts',(5.42519570062476,137.947359574834,12.7713654548078));
#82732=CARTESIAN_POINT('Ctrl Pts',(5.42652106620689,137.956617779177,12.7533192808238));
#82733=CARTESIAN_POINT('Ctrl Pts',(5.42876289862504,137.972859738674,12.7235772645878));
#82734=CARTESIAN_POINT('Ctrl Pts',(5.429670306822,137.979588973214,12.7117469961956));
#82735=CARTESIAN_POINT('Ctrl Pts',(5.43150781347319,137.993513461199,12.6882252865167));
#82736=CARTESIAN_POINT('Ctrl Pts',(5.43243789553479,138.00071112128,12.6765377622134));
#82737=CARTESIAN_POINT('Ctrl Pts',(5.43480468031454,138.019390766301,12.6473605614756));
#82738=CARTESIAN_POINT('Ctrl Pts',(5.43625097664947,138.031137151095,12.6300467265993));
#82739=CARTESIAN_POINT('Ctrl Pts',(5.44341168610429,138.09086175676,12.546872174651));
#82740=CARTESIAN_POINT('Ctrl Pts',(5.44936274420983,138.145118311036,12.4858089584843));
#82741=CARTESIAN_POINT('Ctrl Pts',(5.45835521298162,138.23546263142,12.4031967946221));
#82742=CARTESIAN_POINT('Ctrl Pts',(5.46136226373166,138.267118942544,12.3771462536125));
#82743=CARTESIAN_POINT('Ctrl Pts',(5.46553499211145,138.31369631189,12.342728155423));
#82744=CARTESIAN_POINT('Ctrl Pts',(5.46674572066487,138.327539309158,12.3329535612546));
#82745=CARTESIAN_POINT('Ctrl Pts',(5.468883428963,138.352644662601,12.3160264638716));
#82746=CARTESIAN_POINT('Ctrl Pts',(5.46981574364695,138.36382663477,12.3087602006212));
#82747=CARTESIAN_POINT('Ctrl Pts',(5.47128644511262,138.381876454392,12.2974623757708));
#82748=CARTESIAN_POINT('Ctrl Pts',(5.4718320716982,138.388665622955,12.2933080437457));
#82749=CARTESIAN_POINT('Ctrl Pts',(5.47291596152569,138.402349558227,12.2851242580265));
#82750=CARTESIAN_POINT('Ctrl Pts',(5.47345417100921,138.409244231173,12.2810954641386));
#82751=CARTESIAN_POINT('Ctrl Pts',(5.47488848877806,138.42786988857,12.2704644819648));
#82752=CARTESIAN_POINT('Ctrl Pts',(5.47577687469264,138.439674327441,12.263992554982));
#82753=CARTESIAN_POINT('Ctrl Pts',(5.48132573606793,138.514898910071,12.224411784423));
#82754=CARTESIAN_POINT('Ctrl Pts',(5.4857185384777,138.581121825655,12.1969330431389));
#82755=CARTESIAN_POINT('Ctrl Pts',(5.49440436971266,138.715298149315,12.1550985405107));
#82756=CARTESIAN_POINT('Ctrl Pts',(5.49868088550042,138.782829577452,12.1403922561227));
#82757=CARTESIAN_POINT('Ctrl Pts',(5.504451557816,138.871356907183,12.1291214330861));
#82758=CARTESIAN_POINT('Ctrl Pts',(5.50577586535948,138.891519599696,12.1270815940121));
#82759=CARTESIAN_POINT('Ctrl Pts',(5.50801644032936,138.925292438844,12.1245430731091));
#82760=CARTESIAN_POINT('Ctrl Pts',(5.50892367270809,138.938877082432,12.123758456197));
#82761=CARTESIAN_POINT('Ctrl Pts',(5.51076125356541,138.966189655999,12.1226553565063));
#82762=CARTESIAN_POINT('Ctrl Pts',(5.51169159263162,138.979915615594,12.1223412469484));
#82763=CARTESIAN_POINT('Ctrl Pts',(5.51405994577189,139.014581725053,12.1221541440527));
#82764=CARTESIAN_POINT('Ctrl Pts',(5.51550757974184,139.035518048069,12.1225995338542));
#82765=CARTESIAN_POINT('Ctrl Pts',(5.52265668607394,139.137627038583,12.1274975702691));
#82766=CARTESIAN_POINT('Ctrl Pts',(5.52859348008077,139.218190073044,12.1397878829998));
#82767=CARTESIAN_POINT('Ctrl Pts',(5.53886463003402,139.353504388969,12.1750291775378));
#82768=CARTESIAN_POINT('Ctrl Pts',(5.54316288031464,139.409002349907,12.1939968366965));
#82769=CARTESIAN_POINT('Ctrl Pts',(5.54821765706877,139.474884686811,12.2221546852387));
#82770=CARTESIAN_POINT('Ctrl Pts',(5.54913123439586,139.486820825186,12.2274928865683));
#82771=CARTESIAN_POINT('Ctrl Pts',(5.55057969761034,139.505828385554,12.2363763783334));
#82772=CARTESIAN_POINT('Ctrl Pts',(5.55112146934786,139.51295699207,12.2397959162087));
#82773=CARTESIAN_POINT('Ctrl Pts',(5.55220525987916,139.527266846377,12.246838371377));
#82774=CARTESIAN_POINT('Ctrl Pts',(5.55274711503062,139.534446466314,12.2504635654175));
#82775=CARTESIAN_POINT('Ctrl Pts',(5.55420323507417,139.553788757455,12.2604799990579));
#82776=CARTESIAN_POINT('Ctrl Pts',(5.55510936576549,139.565878035677,12.2670111765799));
#82777=CARTESIAN_POINT('Ctrl Pts',(5.56041828001316,139.636802180623,12.3069465628515));
#82778=CARTESIAN_POINT('Ctrl Pts',(5.56458486368812,139.692791083732,12.3451623834168));
#82779=CARTESIAN_POINT('Ctrl Pts',(5.57329425858792,139.801936855504,12.4343431609599));
#82780=CARTESIAN_POINT('Ctrl Pts',(5.57782570260514,139.854223497474,12.485896096615));
#82781=CARTESIAN_POINT('Ctrl Pts',(5.58385202193002,139.914147309965,12.5571519076069));
#82782=CARTESIAN_POINT('Ctrl Pts',(5.5851495800213,139.926529019252,12.5726538002598));
#82783=CARTESIAN_POINT('Ctrl Pts',(5.58735831220056,139.946688095044,12.5992433914044));
#82784=CARTESIAN_POINT('Ctrl Pts',(5.58826103824763,139.954676642614,12.6101662113392));
#82785=CARTESIAN_POINT('Ctrl Pts',(5.59010058705978,139.970439696361,12.6325175341307));
#82786=CARTESIAN_POINT('Ctrl Pts',(5.59103758041169,139.978204736135,12.6439500686964));
#82787=CARTESIAN_POINT('Ctrl Pts',(5.59344702684949,139.997492648709,12.6734517847421));
#82788=CARTESIAN_POINT('Ctrl Pts',(5.59492980259,140.008726366072,12.6917029803105));
#82789=CARTESIAN_POINT('Ctrl Pts',(5.60159010376457,140.056365412248,12.7740528516412));
#82790=CARTESIAN_POINT('Ctrl Pts',(5.6069541650649,140.087198753013,12.8411710030868));
#82791=CARTESIAN_POINT('Ctrl Pts',(5.61698541386664,140.132348926649,12.9700929585311));
#82792=CARTESIAN_POINT('Ctrl Pts',(5.621619834382,140.148353484114,13.0310423328067));
#82793=CARTESIAN_POINT('Ctrl Pts',(5.62708408981924,140.161924378232,13.1070468534625));
#82794=CARTESIAN_POINT('Ctrl Pts',(5.62808517315643,140.164179656184,13.1211566293868));
#82795=CARTESIAN_POINT('Ctrl Pts',(5.62963745027156,140.167318029675,13.1433788881588));
#82796=CARTESIAN_POINT('Ctrl Pts',(5.63019723912315,140.168374476613,13.1514649957636));
#82797=CARTESIAN_POINT('Ctrl Pts',(5.63128419683653,140.170278751526,13.1673207724025));
#82798=CARTESIAN_POINT('Ctrl Pts',(5.63181166198327,140.171133381566,13.1750890643912));
#82799=CARTESIAN_POINT('Ctrl Pts',(5.63318032130447,140.173165669468,13.1954217536104));
#82800=CARTESIAN_POINT('Ctrl Pts',(5.63401500409069,140.174218874817,13.207998023348));
#82801=CARTESIAN_POINT('Ctrl Pts',(5.63879696128575,140.179144999282,13.2808918321207));
#82802=CARTESIAN_POINT('Ctrl Pts',(5.64254940791926,140.178572740028,13.3414262097369));
#82803=CARTESIAN_POINT('Ctrl Pts',(5.65123880748795,140.166445947691,13.4813995121271));
#82804=CARTESIAN_POINT('Ctrl Pts',(5.65615372363999,140.151426958968,13.5602238133784));
#82805=CARTESIAN_POINT('Ctrl Pts',(5.66267891362915,140.122509026128,13.6570880227883));
#82806=CARTESIAN_POINT('Ctrl Pts',(5.66405292482351,140.115946369976,13.6770967790771));
#82807=CARTESIAN_POINT('Ctrl Pts',(5.66635299728729,140.104217435125,13.7098633610865));
#82808=CARTESIAN_POINT('Ctrl Pts',(5.6672689013546,140.099357403154,13.7227261429256));
#82809=CARTESIAN_POINT('Ctrl Pts',(5.66910496668744,140.089249430018,13.7481242495252));
#82810=CARTESIAN_POINT('Ctrl Pts',(5.6700248085621,140.084007514727,13.7606596844854));
#82811=CARTESIAN_POINT('Ctrl Pts',(5.67232758836512,140.070453950662,13.7915583552907));
#82812=CARTESIAN_POINT('Ctrl Pts',(5.67371905473031,140.061885815778,13.8098035936312));
#82813=CARTESIAN_POINT('Ctrl Pts',(5.67679041771837,140.042169092015,13.8491330471507));
#82814=CARTESIAN_POINT('Ctrl Pts',(5.67847581454526,140.030839853676,13.8701162895264));
#82815=CARTESIAN_POINT('Ctrl Pts',(5.6839078867832,139.992709798467,13.9358813150836));
#82816=CARTESIAN_POINT('Ctrl Pts',(5.6877203422653,139.963568432228,13.9792295622909));
#82817=CARTESIAN_POINT('Ctrl Pts',(5.69619546502041,139.892964018112,14.0705256025989));
#82818=CARTESIAN_POINT('Ctrl Pts',(5.70085502399822,139.850306624853,14.1173581207714));
#82819=CARTESIAN_POINT('Ctrl Pts',(5.70634091658295,139.793668346083,14.1702810647204));
#82820=CARTESIAN_POINT('Ctrl Pts',(5.70734048050977,139.783068130794,14.1798311901365));
#82821=CARTESIAN_POINT('Ctrl Pts',(5.70889093767647,139.76614352106,14.1945309301579));
#82822=CARTESIAN_POINT('Ctrl Pts',(5.70945039581487,139.759935071139,14.1998111899257));
#82823=CARTESIAN_POINT('Ctrl Pts',(5.71053724938134,139.74766424837,14.2100298672042));
#82824=CARTESIAN_POINT('Ctrl Pts',(5.7110649335467,139.741606621542,14.2149731209203));
#82825=CARTESIAN_POINT('Ctrl Pts',(5.71243486977979,139.725631779048,14.2277463160764));
#82826=CARTESIAN_POINT('Ctrl Pts',(5.71327058834887,139.715636652824,14.2354779094405));
#82827=CARTESIAN_POINT('Ctrl Pts',(5.71807770182441,139.656825463542,14.2794760992685));
#82828=CARTESIAN_POINT('Ctrl Pts',(5.72185189642722,139.605377842012,14.3120832946091));
#82829=CARTESIAN_POINT('Ctrl Pts',(5.73053358443415,139.481345643389,14.3778361135982));
#82830=CARTESIAN_POINT('Ctrl Pts',(5.7354201748421,139.40746773503,14.4078776600163));
#82831=CARTESIAN_POINT('Ctrl Pts',(5.74191623340544,139.310881346831,14.4361747250445));
#82832=CARTESIAN_POINT('Ctrl Pts',(5.74329300544873,139.290479060936,14.4415612309419));
#82833=CARTESIAN_POINT('Ctrl Pts',(5.74559646017639,139.256551573897,14.4495501975841));
#82834=CARTESIAN_POINT('Ctrl Pts',(5.74651292423807,139.243105332055,14.4524687142399));
#82835=CARTESIAN_POINT('Ctrl Pts',(5.74834917249006,139.216290525029,14.4577987437709));
#82836=CARTESIAN_POINT('Ctrl Pts',(5.7492686217734,139.20292524099,14.4602158600819));
#82837=CARTESIAN_POINT('Ctrl Pts',(5.75156856492829,139.169663841002,14.4656389052601));
#82838=CARTESIAN_POINT('Ctrl Pts',(5.75295753760276,139.149727499954,14.4683670079621));
#82839=CARTESIAN_POINT('Ctrl Pts',(5.75916946047362,139.061280563168,14.478169308158));
#82840=CARTESIAN_POINT('Ctrl Pts',(5.76415635910438,138.992305898096,14.4797357087017));
#82841=CARTESIAN_POINT('Ctrl Pts',(5.77449130118481,138.851683660659,14.4705943404318));
#82842=CARTESIAN_POINT('Ctrl Pts',(5.77982313106866,138.780343914151,14.4593280257754));
#82843=CARTESIAN_POINT('Ctrl Pts',(5.78585957697632,138.697482296256,14.4383135992868));
#82844=CARTESIAN_POINT('Ctrl Pts',(5.78679716732042,138.684543177039,14.4347959475824));
#82845=CARTESIAN_POINT('Ctrl Pts',(5.78827417049479,138.664008007576,14.4288348129303));
#82846=CARTESIAN_POINT('Ctrl Pts',(5.78882092268096,138.656372224463,14.4265338943831));
#82847=CARTESIAN_POINT('Ctrl Pts',(5.78990515185667,138.641150085642,14.4217777711124));
#82848=CARTESIAN_POINT('Ctrl Pts',(5.79044260290603,138.63356410951,14.4193227310849));
#82849=CARTESIAN_POINT('Ctrl Pts',(5.79187186642266,138.613302138685,14.4125372981453));
#82850=CARTESIAN_POINT('Ctrl Pts',(5.79275605677644,138.600673720773,14.4080672525052));
#82851=CARTESIAN_POINT('Ctrl Pts',(5.79739757632423,138.534075080732,14.3832069670563));
#82852=CARTESIAN_POINT('Ctrl Pts',(5.80098340406711,138.481575453042,14.3590849292308));
#82853=CARTESIAN_POINT('Ctrl Pts',(5.80960056734649,138.359622209106,14.2917996029529));
#82854=CARTESIAN_POINT('Ctrl Pts',(5.814605247174,138.292488523141,14.2450799999782));
#82855=CARTESIAN_POINT('Ctrl Pts',(5.82122224019893,138.214893499294,14.1781457080737));
#82856=CARTESIAN_POINT('Ctrl Pts',(5.82258689779781,138.199430936439,14.1640724448636));
#82857=CARTESIAN_POINT('Ctrl Pts',(5.82487589799893,138.174451134215,14.1400907700195));
#82858=CARTESIAN_POINT('Ctrl Pts',(5.82579030349428,138.164717750215,14.1304137330231));
#82859=CARTESIAN_POINT('Ctrl Pts',(5.82762693125639,138.145669640668,14.1108021250543));
#82860=CARTESIAN_POINT('Ctrl Pts',(5.82854889259997,138.136353698801,14.1008717052129));
#82861=CARTESIAN_POINT('Ctrl Pts',(5.83086418808924,138.113580343084,14.0757367189011));
#82862=CARTESIAN_POINT('Ctrl Pts',(5.83226624931656,138.100340469371,14.0603419658106));
#82863=CARTESIAN_POINT('Ctrl Pts',(5.83864515977085,138.042590394452,13.9895715476658));
#82864=CARTESIAN_POINT('Ctrl Pts',(5.84379732247673,138.002754144235,13.930586924838));
#82865=CARTESIAN_POINT('Ctrl Pts',(5.85398720208869,137.935738527889,13.8089646980205));
#82866=CARTESIAN_POINT('Ctrl Pts',(5.85899827146271,137.908192168437,13.7468264717829));
#82867=CARTESIAN_POINT('Ctrl Pts',(5.8638006232474,137.886148212477,13.6826607608994));
#82868=CARTESIAN_POINT('Origin',(1.13913288526384,139.,13.3));
#82869=CARTESIAN_POINT('',(6.33649999999995,138.079525356866,14.0347254547431));
#82870=CARTESIAN_POINT('Ctrl Pts',(5.8638006232474,137.886148212477,13.6826607608994));
#82871=CARTESIAN_POINT('Ctrl Pts',(5.86388429847287,137.885764122958,13.6815427502732));
#82872=CARTESIAN_POINT('Ctrl Pts',(5.86396790781912,137.885381703865,13.6804241239518));
#82873=CARTESIAN_POINT('Ctrl Pts',(5.86501791222874,137.880596250179,13.6663568749282));
#82874=CARTESIAN_POINT('Ctrl Pts',(5.86597495468775,137.876417174238,13.653332405962));
#82875=CARTESIAN_POINT('Ctrl Pts',(5.8674750424359,137.870146044216,13.6325501113088));
#82876=CARTESIAN_POINT('Ctrl Pts',(5.86802580447681,137.867904963955,13.624839001515));
#82877=CARTESIAN_POINT('Ctrl Pts',(5.86911002365038,137.863612681198,13.6094858914516));
#82878=CARTESIAN_POINT('Ctrl Pts',(5.86964356156651,137.861559283325,13.6018449894409));
#82879=CARTESIAN_POINT('Ctrl Pts',(5.87105082358635,137.856306395664,13.5814819248007));
#82880=CARTESIAN_POINT('Ctrl Pts',(5.87191731820684,137.853242080742,13.5687255939068));
#82881=CARTESIAN_POINT('Ctrl Pts',(5.87650062730565,137.838001074446,13.500262063147));
#82882=CARTESIAN_POINT('Ctrl Pts',(5.88004814748423,137.829667640453,13.4437709197346));
#82883=CARTESIAN_POINT('Ctrl Pts',(5.88872563356953,137.819321165168,13.3039161097475));
#82884=CARTESIAN_POINT('Ctrl Pts',(5.89382425388596,137.821992770914,13.2205309687608));
#82885=CARTESIAN_POINT('Ctrl Pts',(5.90053741610881,137.83627768483,13.1175841704042));
#82886=CARTESIAN_POINT('Ctrl Pts',(5.90189153896307,137.839670027961,13.0971221230352));
#82887=CARTESIAN_POINT('Ctrl Pts',(5.90416740850559,137.846194945665,13.0633223863018));
#82888=CARTESIAN_POINT('Ctrl Pts',(5.90507943996471,137.849023241986,13.0499302656062));
#82889=CARTESIAN_POINT('Ctrl Pts',(5.90691475243274,137.855132599291,13.0233061707394));
#82890=CARTESIAN_POINT('Ctrl Pts',(5.90783782953162,137.858411285979,13.0100758354617));
#82891=CARTESIAN_POINT('Ctrl Pts',(5.91016281059429,137.867175000761,12.9771691638174));
#82892=CARTESIAN_POINT('Ctrl Pts',(5.91157362505443,137.872943493823,12.9575737032044));
#82893=CARTESIAN_POINT('Ctrl Pts',(5.91469660230516,137.886679352213,12.9150300031026));
#82894=CARTESIAN_POINT('Ctrl Pts',(5.91641460950508,137.894852937134,12.892158617108));
#82895=CARTESIAN_POINT('Ctrl Pts',(5.92202047917009,137.923499488783,12.8192001206648));
#82896=CARTESIAN_POINT('Ctrl Pts',(5.92597906404474,137.946716545242,12.7702690223766));
#82897=CARTESIAN_POINT('Ctrl Pts',(5.93440413821536,138.002898876133,12.6702717100563));
#82898=CARTESIAN_POINT('Ctrl Pts',(5.93886262816819,138.03662278238,12.6197986465558));
#82899=CARTESIAN_POINT('Ctrl Pts',(5.94414752971355,138.08279209635,12.5610661509843));
#82900=CARTESIAN_POINT('Ctrl Pts',(5.94513437790824,138.091697949538,12.5501460136798));
#82901=CARTESIAN_POINT('Ctrl Pts',(5.94666964013626,138.106036766014,12.5331945500879));
#82902=CARTESIAN_POINT('Ctrl Pts',(5.94722636665947,138.1113394724,12.5270554105948));
#82903=CARTESIAN_POINT('Ctrl Pts',(5.94831229026802,138.121894983259,12.5150871400933));
#82904=CARTESIAN_POINT('Ctrl Pts',(5.94884171400997,138.127143379395,12.5092548171225));
#82905=CARTESIAN_POINT('Ctrl Pts',(5.95022221904615,138.141086339032,12.4940685759916));
#82906=CARTESIAN_POINT('Ctrl Pts',(5.95106657794797,138.149875733096,12.4848025385747));
#82907=CARTESIAN_POINT('Ctrl Pts',(5.95583182697117,138.200856274503,12.432778890627));
#82908=CARTESIAN_POINT('Ctrl Pts',(5.95956152283631,138.2461238645,12.3931506946587));
#82909=CARTESIAN_POINT('Ctrl Pts',(5.96823776050969,138.358425199584,12.3090870509977));
#82910=CARTESIAN_POINT('Ctrl Pts',(5.97316187064017,138.427361911429,12.2677157093157));
#82911=CARTESIAN_POINT('Ctrl Pts',(5.97969718534888,138.519025009362,12.2247319724928));
#82912=CARTESIAN_POINT('Ctrl Pts',(5.98107110326613,138.538321106448,12.2163068775723));
#82913=CARTESIAN_POINT('Ctrl Pts',(5.983371425969,138.570580197344,12.2032398227215));
#82914=CARTESIAN_POINT('Ctrl Pts',(5.98428768673723,138.5834177004,12.198299762182));
#82915=CARTESIAN_POINT('Ctrl Pts',(5.98612480738559,138.609111535501,12.188925680898));
#82916=CARTESIAN_POINT('Ctrl Pts',(5.98704535313974,138.621963993435,12.1844872546537));
#82917=CARTESIAN_POINT('Ctrl Pts',(5.98935065813083,138.654076438949,12.1740163353991));
#82918=CARTESIAN_POINT('Ctrl Pts',(5.99074396974486,138.673419445305,12.1682547209062));
#82919=CARTESIAN_POINT('Ctrl Pts',(5.99719328657417,138.762601404431,12.1441671026697));
#82920=CARTESIAN_POINT('Ctrl Pts',(6.00243146976876,138.83387563574,12.1317930686623));
#82921=CARTESIAN_POINT('Ctrl Pts',(6.01271796100407,138.973593038792,12.1205848377712));
#82922=CARTESIAN_POINT('Ctrl Pts',(6.01773769207363,139.041711692283,12.1210263213067));
#82923=CARTESIAN_POINT('Ctrl Pts',(6.0235134845494,139.123086667609,12.1286190809397));
#82924=CARTESIAN_POINT('Ctrl Pts',(6.02447434600472,139.136735052204,12.1301337034884));
#82925=CARTESIAN_POINT('Ctrl Pts',(6.02597925489503,139.158333691631,12.1329137880145));
#82926=CARTESIAN_POINT('Ctrl Pts',(6.02653108535776,139.166302406915,12.1340225974664));
#82927=CARTESIAN_POINT('Ctrl Pts',(6.02761771237501,139.182103367527,12.1363865201235));
#82928=CARTESIAN_POINT('Ctrl Pts',(6.02815259224737,139.189935507188,12.1376392649964));
#82929=CARTESIAN_POINT('Ctrl Pts',(6.02956289708903,139.210710750106,12.1411778511123));
#82930=CARTESIAN_POINT('Ctrl Pts',(6.03043109134659,139.223629679946,12.1436014549905));
#82931=CARTESIAN_POINT('Ctrl Pts',(6.03516709088313,139.294624084771,12.1581544083189));
#82932=CARTESIAN_POINT('Ctrl Pts',(6.03885169377139,139.35176610428,12.1744437060111));
#82933=CARTESIAN_POINT('Ctrl Pts',(6.04746113527142,139.482323087329,12.2225823026564));
#82934=CARTESIAN_POINT('Ctrl Pts',(6.05236386339738,139.554196096006,12.25772858667));
#82935=CARTESIAN_POINT('Ctrl Pts',(6.05887427098244,139.639832034485,12.3109838574783));
#82936=CARTESIAN_POINT('Ctrl Pts',(6.06024780836079,139.657401276196,12.3225740761671));
#82937=CARTESIAN_POINT('Ctrl Pts',(6.06254821060037,139.685929728721,12.342511175626));
#82938=CARTESIAN_POINT('Ctrl Pts',(6.06346496497236,139.697070232362,12.3505909703074));
#82939=CARTESIAN_POINT('Ctrl Pts',(6.0653037997633,139.718945455063,12.3670488504726));
#82940=CARTESIAN_POINT('Ctrl Pts',(6.06622557742651,139.7296815297,12.3754215809716));
#82941=CARTESIAN_POINT('Ctrl Pts',(6.06853559039883,139.756004406844,12.3966940316266));
#82942=CARTESIAN_POINT('Ctrl Pts',(6.06993243201465,139.771407984662,12.4098123969246));
#82943=CARTESIAN_POINT('Ctrl Pts',(6.07643963134985,139.840781980793,12.4720474844551));
#82944=CARTESIAN_POINT('Ctrl Pts',(6.08173647831567,139.890444298323,12.5257096608265));
#82945=CARTESIAN_POINT('Ctrl Pts',(6.09202481613722,139.975699416828,12.6369592013763));
#82946=CARTESIAN_POINT('Ctrl Pts',(6.09698564163917,140.011943350347,12.6937125725571));
#82947=CARTESIAN_POINT('Ctrl Pts',(6.10270897611318,140.049534863066,12.7654339929871));
#82948=CARTESIAN_POINT('Ctrl Pts',(6.10367162538994,140.055706518563,12.7777280091128));
#82949=CARTESIAN_POINT('Ctrl Pts',(6.1051783486569,140.065144686429,12.7973802763873));
#82950=CARTESIAN_POINT('Ctrl Pts',(6.10573024972679,140.06855339559,12.8046683534998));
#82951=CARTESIAN_POINT('Ctrl Pts',(6.10681154309127,140.075140461854,12.8191365156545));
#82952=CARTESIAN_POINT('Ctrl Pts',(6.10734107359761,140.078322190201,12.8263144888929));
#82953=CARTESIAN_POINT('Ctrl Pts',(6.10873289475328,140.086559034315,12.8454099734943));
#82954=CARTESIAN_POINT('Ctrl Pts',(6.10958814465885,140.091490042094,12.8573803553823));
#82955=CARTESIAN_POINT('Ctrl Pts',(6.11149963342392,140.102181672413,12.8846010537757));
#82956=CARTESIAN_POINT('Ctrl Pts',(6.11255034177036,140.107825143979,12.8998947298897));
#82957=CARTESIAN_POINT('Ctrl Pts',(6.1160336449756,140.125657726872,12.9514944258997));
#82958=CARTESIAN_POINT('Ctrl Pts',(6.11841633888561,140.136394045716,12.9882783405537));
#82959=CARTESIAN_POINT('Ctrl Pts',(6.12619450308222,140.165688472636,13.1105157674858));
#82960=CARTESIAN_POINT('Ctrl Pts',(6.13153281417446,140.176531747214,13.1975040863691));
#82961=CARTESIAN_POINT('Ctrl Pts',(6.13849101411962,140.177912996264,13.3051464559415));
#82962=CARTESIAN_POINT('Ctrl Pts',(6.13981462610736,140.177650175574,13.3254066310971));
#82963=CARTESIAN_POINT('Ctrl Pts',(6.14196154838472,140.176391992006,13.3578435269128));
#82964=CARTESIAN_POINT('Ctrl Pts',(6.14277439314997,140.175729490964,13.37002954761));
#82965=CARTESIAN_POINT('Ctrl Pts',(6.144491614268,140.173943284059,13.3955588173051));
#82966=CARTESIAN_POINT('Ctrl Pts',(6.14539708349905,140.172781149451,13.4088975269846));
#82967=CARTESIAN_POINT('Ctrl Pts',(6.14762574436898,140.169388815348,13.4414124868713));
#82968=CARTESIAN_POINT('Ctrl Pts',(6.14895641344086,140.166914101173,13.4605586998893));
#82969=CARTESIAN_POINT('Ctrl Pts',(6.15546449213715,140.152668980707,13.552862208939));
#82970=CARTESIAN_POINT('Ctrl Pts',(6.16083926999172,140.134484603582,13.6248482794014));
#82971=CARTESIAN_POINT('Ctrl Pts',(6.1712657504787,140.08689667474,13.758658557791));
#82972=CARTESIAN_POINT('Ctrl Pts',(6.17628455711596,140.058629469,13.8205929803066));
#82973=CARTESIAN_POINT('Ctrl Pts',(6.18205739065044,140.018429411803,13.8916793828944));
#82974=CARTESIAN_POINT('Ctrl Pts',(6.18301687708695,140.011473709464,13.9034931109229));
#82975=CARTESIAN_POINT('Ctrl Pts',(6.18451858419541,140.000125392176,13.9220197219643));
#82976=CARTESIAN_POINT('Ctrl Pts',(6.18506860854523,139.99586795791,13.928813450086));
#82977=CARTESIAN_POINT('Ctrl Pts',(6.18615345272547,139.987262114329,13.9422394104626));
#82978=CARTESIAN_POINT('Ctrl Pts',(6.18668835008692,139.982915440471,13.9488722438488));
#82979=CARTESIAN_POINT('Ctrl Pts',(6.18809594195657,139.971212033487,13.9663436236591));
#82980=CARTESIAN_POINT('Ctrl Pts',(6.18896148509673,139.96374069779,13.9771045277775));
#82981=CARTESIAN_POINT('Ctrl Pts',(6.1908979520067,139.946442957386,14.0011517491167));
#82982=CARTESIAN_POINT('Ctrl Pts',(6.19196323820623,139.93651324492,14.0143605836771));
#82983=CARTESIAN_POINT('Ctrl Pts',(6.19551184805883,139.902173847614,14.0580927311291));
#82984=CARTESIAN_POINT('Ctrl Pts',(6.19794411082411,139.876522923783,14.0876104242493));
#82985=CARTESIAN_POINT('Ctrl Pts',(6.20565321818898,139.790303402123,14.1773863973868));
#82986=CARTESIAN_POINT('Ctrl Pts',(6.21088197070647,139.724640383652,14.2323524911233));
#82987=CARTESIAN_POINT('Ctrl Pts',(6.21773137317214,139.636502016156,14.2911525821974));
#82988=CARTESIAN_POINT('Ctrl Pts',(6.21907557877539,139.619093728675,14.3021183215479));
#82989=CARTESIAN_POINT('Ctrl Pts',(6.22125317388596,139.590790530953,14.3189279199268));
#82990=CARTESIAN_POINT('Ctrl Pts',(6.2220758493248,139.5800748715,14.3250661839411));
#82991=CARTESIAN_POINT('Ctrl Pts',(6.22381244859305,139.557422870829,14.3375730299381));
#82992=CARTESIAN_POINT('Ctrl Pts',(6.22472745425368,139.545469413245,14.3439066731371));
#82993=CARTESIAN_POINT('Ctrl Pts',(6.22697818111198,139.516039678553,14.3588567897391));
#82994=CARTESIAN_POINT('Ctrl Pts',(6.22832141127089,139.498454098391,14.3672479020036));
#82995=CARTESIAN_POINT('Ctrl Pts',(6.23126341524257,139.459914175857,14.3844772403081));
#82996=CARTESIAN_POINT('Ctrl Pts',(6.23286681494723,139.438895909499,14.3931524135736));
#82997=CARTESIAN_POINT('Ctrl Pts',(6.23787848328468,139.373146103655,14.4180883670959));
#82998=CARTESIAN_POINT('Ctrl Pts',(6.24134087382142,139.327673173329,14.4322496142402));
#82999=CARTESIAN_POINT('Ctrl Pts',(6.25008232148965,139.211863221704,14.4607531885076));
#83000=CARTESIAN_POINT('Ctrl Pts',(6.25538087482368,139.140831027734,14.4714956345091));
#83001=CARTESIAN_POINT('Ctrl Pts',(6.26139339108035,139.055800987709,14.4765045931462));
#83002=CARTESIAN_POINT('Ctrl Pts',(6.26233584792604,139.042329668211,14.4770662877853));
#83003=CARTESIAN_POINT('Ctrl Pts',(6.26382162079893,139.020819220759,14.4775933807646));
#83004=CARTESIAN_POINT('Ctrl Pts',(6.2643722898191,139.012785277379,14.4777080111588));
#83005=CARTESIAN_POINT('Ctrl Pts',(6.26547263791033,138.996595007922,14.4777733143393));
#83006=CARTESIAN_POINT('Ctrl Pts',(6.26602218910655,138.98843919673,14.4777215000115));
#83007=CARTESIAN_POINT('Ctrl Pts',(6.26749412076351,138.966427977915,14.4773529771649));
#83008=CARTESIAN_POINT('Ctrl Pts',(6.26840842260547,138.952576110722,14.4768764288358));
#83009=CARTESIAN_POINT('Ctrl Pts',(6.27229242752807,138.893139300363,14.4737804212127));
#83010=CARTESIAN_POINT('Ctrl Pts',(6.27516254570757,138.847715446294,14.4687557134296));
#83011=CARTESIAN_POINT('Ctrl Pts',(6.28386509981517,138.709938874972,14.445343439677));
#83012=CARTESIAN_POINT('Ctrl Pts',(6.28960799220818,138.619414917274,14.4185261274396));
#83013=CARTESIAN_POINT('Ctrl Pts',(6.29694413515152,138.515680411153,14.3737259717958));
#83014=CARTESIAN_POINT('Ctrl Pts',(6.29818458587999,138.498497570866,14.365808695567));
#83015=CARTESIAN_POINT('Ctrl Pts',(6.30033228925,138.469417692123,14.3515507408203));
#83016=CARTESIAN_POINT('Ctrl Pts',(6.30123250840675,138.45742488312,14.3454132021188));
#83017=CARTESIAN_POINT('Ctrl Pts',(6.30310052824236,138.432959625793,14.3323582806929));
#83018=CARTESIAN_POINT('Ctrl Pts',(6.30406904216647,138.420502321822,14.325417386115));
#83019=CARTESIAN_POINT('Ctrl Pts',(6.30664165626679,138.388026725982,14.3065420210254));
#83020=CARTESIAN_POINT('Ctrl Pts',(6.30825873548165,138.368232218685,14.2942371275064));
#83021=CARTESIAN_POINT('Ctrl Pts',(6.31401487686354,138.299965394141,14.2489382771781));
#83022=CARTESIAN_POINT('Ctrl Pts',(6.3182578918509,138.253608771117,14.2129243242085));
#83023=CARTESIAN_POINT('Ctrl Pts',(6.32721731896174,138.162912781018,14.1309224802077));
#83024=CARTESIAN_POINT('Ctrl Pts',(6.33192829751966,138.119239112282,14.0844794201302));
#83025=CARTESIAN_POINT('Ctrl Pts',(6.33649999999999,138.079525356866,14.0347254547424));
#83026=CARTESIAN_POINT('',(6.3365,139.383133178262,14.4136893777957));
#83027=CARTESIAN_POINT('Origin',(6.3365,139.,13.3));
#83028=CARTESIAN_POINT('Ctrl Pts',(6.33649999999995,139.383133178262,14.4136893777957));
#83029=CARTESIAN_POINT('Ctrl Pts',(6.33587794040813,139.39183892307,14.4106944137203));
#83030=CARTESIAN_POINT('Ctrl Pts',(6.33526140785785,139.400500155674,14.4076007669009));
#83031=CARTESIAN_POINT('Ctrl Pts',(6.33378043727113,139.42136007669,14.3998730575355));
#83032=CARTESIAN_POINT('Ctrl Pts',(6.33292104407913,139.433510703543,14.3951408829234));
#83033=CARTESIAN_POINT('Ctrl Pts',(6.32882557181164,139.491493715694,14.371442544551));
#83034=CARTESIAN_POINT('Ctrl Pts',(6.32568526225882,139.536179075507,14.3497942400076));
#83035=CARTESIAN_POINT('Ctrl Pts',(6.318988600977,139.628593333067,14.2975781068897));
#83036=CARTESIAN_POINT('Ctrl Pts',(6.31544253077134,139.675749179254,14.2662579152729));
#83037=CARTESIAN_POINT('Ctrl Pts',(6.30987331788833,139.744370761575,14.2131921608729));
#83038=CARTESIAN_POINT('Ctrl Pts',(6.30791276280052,139.767547955054,14.1937995801075));
#83039=CARTESIAN_POINT('Ctrl Pts',(6.30484934575064,139.802011204962,14.162633990819));
#83040=CARTESIAN_POINT('Ctrl Pts',(6.30376892420992,139.81384200014,14.1514813766365));
#83041=CARTESIAN_POINT('Ctrl Pts',(6.30170981439692,139.835747906835,14.1299574825064));
#83042=CARTESIAN_POINT('Ctrl Pts',(6.30073331251273,139.845870329287,14.1196385441256));
#83043=CARTESIAN_POINT('Ctrl Pts',(6.29847275148654,139.868675127387,14.0955185719317));
#83044=CARTESIAN_POINT('Ctrl Pts',(6.29718369276969,139.881222804303,14.0815961731514));
#83045=CARTESIAN_POINT('Ctrl Pts',(6.29280036627322,139.922325179097,14.0337422456227));
#83046=CARTESIAN_POINT('Ctrl Pts',(6.28964809556392,139.949291733903,13.9985025433935));
#83047=CARTESIAN_POINT('Ctrl Pts',(6.2803038503246,140.021832340654,13.8917237514861));
#83048=CARTESIAN_POINT('Ctrl Pts',(6.2739700929141,140.061751209004,13.8166825090063));
#83049=CARTESIAN_POINT('Ctrl Pts',(6.26516849211967,140.106506857402,13.7049750073844));
#83050=CARTESIAN_POINT('Ctrl Pts',(6.2625966176464,140.118242129848,13.6713451527501));
#83051=CARTESIAN_POINT('Ctrl Pts',(6.25930437465062,140.13165283657,13.6264706348102));
#83052=CARTESIAN_POINT('Ctrl Pts',(6.25852192277366,140.134714976903,13.61566305327));
#83053=CARTESIAN_POINT('Ctrl Pts',(6.25722804877182,140.139574209788,13.5975274275939));
#83054=CARTESIAN_POINT('Ctrl Pts',(6.25671206725283,140.141456306223,13.5902231235643));
#83055=CARTESIAN_POINT('Ctrl Pts',(6.25563622157122,140.145264962526,13.5748314592414));
#83056=CARTESIAN_POINT('Ctrl Pts',(6.25507724415385,140.14717632589,13.566740798136));
#83057=CARTESIAN_POINT('Ctrl Pts',(6.25346529163954,140.152483708809,13.5431619907188));
#83058=CARTESIAN_POINT('Ctrl Pts',(6.25242437088168,140.155652981513,13.5276240325921));
#83059=CARTESIAN_POINT('Ctrl Pts',(6.24664106555966,140.171710079176,13.4398881854822));
#83060=CARTESIAN_POINT('Ctrl Pts',(6.24216368030448,140.178147377323,13.3666666991411));
#83061=CARTESIAN_POINT('Ctrl Pts',(6.23367171165806,140.177367646384,13.2292952048428));
#83062=CARTESIAN_POINT('Ctrl Pts',(6.22968485762245,140.171785098228,13.1654188036648));
#83063=CARTESIAN_POINT('Ctrl Pts',(6.22434810456065,140.157970918278,13.0842849758959));
#83064=CARTESIAN_POINT('Ctrl Pts',(6.22315005479749,140.154481336154,13.0663284299189));
#83065=CARTESIAN_POINT('Ctrl Pts',(6.22108935133543,140.147837752813,13.0359397092644));
#83066=CARTESIAN_POINT('Ctrl Pts',(6.22023375211713,140.14489618224,13.0234641920897));
#83067=CARTESIAN_POINT('Ctrl Pts',(6.21847475026451,140.138482613059,12.9981226466729));
#83068=CARTESIAN_POINT('Ctrl Pts',(6.2175709263667,140.134994692483,12.9852626200945));
#83069=CARTESIAN_POINT('Ctrl Pts',(6.21522089935695,140.125438827419,12.9522571413018));
#83070=CARTESIAN_POINT('Ctrl Pts',(6.2137640401135,140.119048149415,12.9322109495601));
#83071=CARTESIAN_POINT('Ctrl Pts',(6.20542411609103,140.079883470612,12.8198525194929));
#83072=CARTESIAN_POINT('Ctrl Pts',(6.19816376487795,140.03623399904,12.7317555443674));
#83073=CARTESIAN_POINT('Ctrl Pts',(6.18729018849101,139.954915097848,12.608857867791));
#83074=CARTESIAN_POINT('Ctrl Pts',(6.18367046043542,139.925054842858,12.5693736222591));
#83075=CARTESIAN_POINT('Ctrl Pts',(6.17936549517341,139.885210100701,12.5230614720746));
#83076=CARTESIAN_POINT('Ctrl Pts',(6.17855351202164,139.877492241763,12.5143551744783));
#83077=CARTESIAN_POINT('Ctrl Pts',(6.17724071745705,139.864659934817,12.5003044754389));
#83078=CARTESIAN_POINT('Ctrl Pts',(6.17673445690185,139.859622224225,12.4948916978854));
#83079=CARTESIAN_POINT('Ctrl Pts',(6.17568476850692,139.848986849656,12.4836781540236));
#83080=CARTESIAN_POINT('Ctrl Pts',(6.17514201853855,139.843380189957,12.4778869348197));
#83081=CARTESIAN_POINT('Ctrl Pts',(6.17366403807553,139.827830937322,12.4621523369892));
#83082=CARTESIAN_POINT('Ctrl Pts',(6.17273751171188,139.817768713229,12.4523283996942));
#83083=CARTESIAN_POINT('Ctrl Pts',(6.16786670119043,139.763349017796,12.401068657847));
#83084=CARTESIAN_POINT('Ctrl Pts',(6.16410924810126,139.716009098028,12.3629237241216));
#83085=CARTESIAN_POINT('Ctrl Pts',(6.15698739044969,139.620939412451,12.2977498813693));
#83086=CARTESIAN_POINT('Ctrl Pts',(6.15363002542191,139.573857077063,12.2700685817626));
#83087=CARTESIAN_POINT('Ctrl Pts',(6.14864347910845,139.503146395696,12.2348538474898));
#83088=CARTESIAN_POINT('Ctrl Pts',(6.14708496247102,139.480931893025,12.2246409792109));
#83089=CARTESIAN_POINT('Ctrl Pts',(6.14417688147737,139.439480426757,12.207125521602));
#83090=CARTESIAN_POINT('Ctrl Pts',(6.14283403650462,139.420338883423,12.1996215143352));
#83091=CARTESIAN_POINT('Ctrl Pts',(6.14056946290329,139.388140348323,12.1879615434827));
#83092=CARTESIAN_POINT('Ctrl Pts',(6.13965710046634,139.375189223157,12.1835254238978));
#83093=CARTESIAN_POINT('Ctrl Pts',(6.13781463795178,139.349098664167,12.1750939060503));
#83094=CARTESIAN_POINT('Ctrl Pts',(6.13688463648514,139.33596082673,12.1711005833429));
#83095=CARTESIAN_POINT('Ctrl Pts',(6.13452672103908,139.302749010543,12.161636741288));
#83096=CARTESIAN_POINT('Ctrl Pts',(6.13308952080128,139.282595000403,12.1564669468993));
#83097=CARTESIAN_POINT('Ctrl Pts',(6.12611070324,139.185209126124,12.1342176891967));
#83098=CARTESIAN_POINT('Ctrl Pts',(6.12035125975786,139.106535278959,12.1244161565));
#83099=CARTESIAN_POINT('Ctrl Pts',(6.11037352358319,138.97033370826,12.1212365702705));
#83100=CARTESIAN_POINT('Ctrl Pts',(6.10618894148885,138.913154572245,12.1240653671204));
#83101=CARTESIAN_POINT('Ctrl Pts',(6.10120983535162,138.843082076121,12.1326731580598));
#83102=CARTESIAN_POINT('Ctrl Pts',(6.10027221132328,138.829789255615,12.1345372031516));
#83103=CARTESIAN_POINT('Ctrl Pts',(6.09879126409641,138.808594429436,12.1378797316031));
#83104=CARTESIAN_POINT('Ctrl Pts',(6.09824079294063,138.80067104579,12.1392125137941));
#83105=CARTESIAN_POINT('Ctrl Pts',(6.09714820740042,138.78484146926,12.1420420549567));
#83106=CARTESIAN_POINT('Ctrl Pts',(6.09660616383184,138.776935779286,12.1435389513021));
#83107=CARTESIAN_POINT('Ctrl Pts',(6.09515253223934,138.755613655991,12.1478029614718));
#83108=CARTESIAN_POINT('Ctrl Pts',(6.09424892139357,138.742228675843,12.1507234080612));
#83109=CARTESIAN_POINT('Ctrl Pts',(6.0888727288714,138.662042145758,12.1696906621856));
#83110=CARTESIAN_POINT('Ctrl Pts',(6.08464196497185,138.596690819988,12.1913257080514));
#83111=CARTESIAN_POINT('Ctrl Pts',(6.07599618407227,138.468326522112,12.246686028101));
#83112=CARTESIAN_POINT('Ctrl Pts',(6.07159376738645,138.405749282804,12.2806807813327));
#83113=CARTESIAN_POINT('Ctrl Pts',(6.0656847280062,138.329749861848,12.3313560979192));
#83114=CARTESIAN_POINT('Ctrl Pts',(6.06435902184899,138.313172757481,12.3430389158782));
#83115=CARTESIAN_POINT('Ctrl Pts',(6.06211712410808,138.285993203161,12.363263966436));
#83116=CARTESIAN_POINT('Ctrl Pts',(6.06120994534497,138.275222078557,12.3715728132982));
#83117=CARTESIAN_POINT('Ctrl Pts',(6.05937326178053,138.253885178608,12.3886296973627));
#83118=CARTESIAN_POINT('Ctrl Pts',(6.05844377825641,138.243323523094,12.397379461259));
#83119=CARTESIAN_POINT('Ctrl Pts',(6.05607937311395,138.21706407043,12.4199188189206));
#83120=CARTESIAN_POINT('Ctrl Pts',(6.05463493662559,138.201576527818,12.4339449107868));
#83121=CARTESIAN_POINT('Ctrl Pts',(6.04743259840784,138.127101750642,12.5050881606315));
#83122=CARTESIAN_POINT('Ctrl Pts',(6.04143480755699,138.073834723535,12.5678457268086));
#83123=CARTESIAN_POINT('Ctrl Pts',(6.03112116172141,137.994628320282,12.6837814662704));
#83124=CARTESIAN_POINT('Ctrl Pts',(6.02684136351919,137.965344031437,12.7343271797954));
#83125=CARTESIAN_POINT('Ctrl Pts',(6.02181025751106,137.934265838573,12.7985277616593));
#83126=CARTESIAN_POINT('Ctrl Pts',(6.02090293458051,137.928800917957,12.8103100262251));
#83127=CARTESIAN_POINT('Ctrl Pts',(6.01946269897096,137.920336708624,12.8293788583717));
#83128=CARTESIAN_POINT('Ctrl Pts',(6.01892303046263,137.917213847464,12.8366089786531));
#83129=CARTESIAN_POINT('Ctrl Pts',(6.01784651703916,137.911078749687,12.851213837669));
#83130=CARTESIAN_POINT('Ctrl Pts',(6.01730980898099,137.908068336218,12.8585888996861));
#83131=CARTESIAN_POINT('Ctrl Pts',(6.0158674917216,137.900118689835,12.8786434851459));
#83132=CARTESIAN_POINT('Ctrl Pts',(6.01496990071557,137.895323824892,12.8913793976777));
#83133=CARTESIAN_POINT('Ctrl Pts',(6.00956463698503,137.867479259642,12.9694144516724));
#83134=CARTESIAN_POINT('Ctrl Pts',(6.00530681642411,137.850002139698,13.0365662976106));
#83135=CARTESIAN_POINT('Ctrl Pts',(5.9979945997241,137.830389763774,13.153306239501));
#83136=CARTESIAN_POINT('Ctrl Pts',(5.99495875092827,137.825290680581,13.2022002515034));
#83137=CARTESIAN_POINT('Ctrl Pts',(5.99039335744201,137.822305560256,13.2742816498389));
#83138=CARTESIAN_POINT('Ctrl Pts',(5.98892135908821,137.822027871612,13.2973177590696));
#83139=CARTESIAN_POINT('Ctrl Pts',(5.98616117183293,137.822764447314,13.3399484609698));
#83140=CARTESIAN_POINT('Ctrl Pts',(5.98487869485107,137.823592522017,13.359538215335));
#83141=CARTESIAN_POINT('Ctrl Pts',(5.98269547525246,137.82580757907,13.3924457060391));
#83142=CARTESIAN_POINT('Ctrl Pts',(5.98180301197179,137.82693343009,13.4057773481816));
#83143=CARTESIAN_POINT('Ctrl Pts',(5.97998507793252,137.829666723415,13.4326707298876));
#83144=CARTESIAN_POINT('Ctrl Pts',(5.97905944708958,137.831283427442,13.4462294306781));
#83145=CARTESIAN_POINT('Ctrl Pts',(5.97668281431759,137.836000444955,13.4806826231297));
#83146=CARTESIAN_POINT('Ctrl Pts',(5.97522176016338,137.839427690418,13.5015266432647));
#83147=CARTESIAN_POINT('Ctrl Pts',(5.96986450289777,137.853874809079,13.5767038446651));
#83148=CARTESIAN_POINT('Ctrl Pts',(5.96587313711761,137.868160088882,13.6303007970922));
#83149=CARTESIAN_POINT('Ctrl Pts',(5.96182583603505,137.88614821265,13.6826607614027));
#83150=CARTESIAN_POINT('Origin',(4.2,139.,13.3));
#83151=CARTESIAN_POINT('',(6.33581728267915,139.984084034254,12.216529393001));
#83152=CARTESIAN_POINT('Ctrl Pts',(6.1539436045687,137.5365,13.30000001305));
#83153=CARTESIAN_POINT('Ctrl Pts',(6.1554786574661,137.536499999732,13.2699840581504));
#83154=CARTESIAN_POINT('Ctrl Pts',(6.15698912438489,137.537423421588,13.2399696452689));
#83155=CARTESIAN_POINT('Ctrl Pts',(6.16301247270492,137.544873150686,13.1190592179742));
#83156=CARTESIAN_POINT('Ctrl Pts',(6.16735318751567,137.558955974813,13.0288441755545));
#83157=CARTESIAN_POINT('Ctrl Pts',(6.17441326870151,137.594203252006,12.8897411341594));
#83158=CARTESIAN_POINT('Ctrl Pts',(6.17703614862449,137.609787875827,12.8396890894236));
#83159=CARTESIAN_POINT('Ctrl Pts',(6.18046202158408,137.632490066651,12.7785465162853));
#83160=CARTESIAN_POINT('Ctrl Pts',(6.18114415247651,137.637118028538,12.7665678460758));
#83161=CARTESIAN_POINT('Ctrl Pts',(6.18225778792567,137.644829249767,12.7473643497358));
#83162=CARTESIAN_POINT('Ctrl Pts',(6.18268371592634,137.647814198765,12.7401004747614));
#83163=CARTESIAN_POINT('Ctrl Pts',(6.18354056333019,137.653885016315,12.7256588648311));
#83164=CARTESIAN_POINT('Ctrl Pts',(6.1839714168684,137.656970178306,12.7184811429848));
#83165=CARTESIAN_POINT('Ctrl Pts',(6.18509851049286,137.665129330271,12.6999099235027));
#83166=CARTESIAN_POINT('Ctrl Pts',(6.18579971501334,137.670291667982,12.6885561879562));
#83167=CARTESIAN_POINT('Ctrl Pts',(6.18925072263128,137.696149901868,12.633561726867));
#83168=CARTESIAN_POINT('Ctrl Pts',(6.19209590039935,137.718851069005,12.5909007773802));
#83169=CARTESIAN_POINT('Ctrl Pts',(6.19857832719303,137.77451708012,12.4977194534767));
#83170=CARTESIAN_POINT('Ctrl Pts',(6.20222981230084,137.808581485361,12.4479528045884));
#83171=CARTESIAN_POINT('Ctrl Pts',(6.2105982694274,137.894424984897,12.3377934616047));
#83172=CARTESIAN_POINT('Ctrl Pts',(6.21526610569149,137.948255083061,12.2792291732169));
#83173=CARTESIAN_POINT('Ctrl Pts',(6.22091590879112,138.021923785183,12.211130919032));
#83174=CARTESIAN_POINT('Ctrl Pts',(6.22207936157765,138.037571949193,12.1972755249741));
#83175=CARTESIAN_POINT('Ctrl Pts',(6.22398660281612,138.064015143859,12.1748536864594));
#83176=CARTESIAN_POINT('Ctrl Pts',(6.22473809064365,138.074643620022,12.1660963595008));
#83177=CARTESIAN_POINT('Ctrl Pts',(6.22621473616527,138.095938219664,12.1490495390382));
#83178=CARTESIAN_POINT('Ctrl Pts',(6.22694004981319,138.106598630742,12.1407551266783));
#83179=CARTESIAN_POINT('Ctrl Pts',(6.22869876679474,138.132928346004,12.1208480569078));
#83180=CARTESIAN_POINT('Ctrl Pts',(6.22972583123008,138.148718081361,12.1093985972315));
#83181=CARTESIAN_POINT('Ctrl Pts',(6.2338556578144,138.213811823827,12.0641549984346));
#83182=CARTESIAN_POINT('Ctrl Pts',(6.23685873488663,138.264937137236,12.0330792284287));
#83183=CARTESIAN_POINT('Ctrl Pts',(6.24271668789267,138.370046182637,11.9777009997802));
#83184=CARTESIAN_POINT('Ctrl Pts',(6.24556792817733,138.423885940875,11.9533711964888));
#83185=CARTESIAN_POINT('Ctrl Pts',(6.25158895180208,138.539193975956,11.9094488321205));
#83186=CARTESIAN_POINT('Ctrl Pts',(6.25475813478067,138.600781412457,11.8905327782686));
#83187=CARTESIAN_POINT('Ctrl Pts',(6.25894564638718,138.679168607552,11.8720077897916));
#83188=CARTESIAN_POINT('Ctrl Pts',(6.25979860346928,138.694989784608,11.8685450543358));
#83189=CARTESIAN_POINT('Ctrl Pts',(6.26113117679804,138.71940425859,11.8636246419722));
#83190=CARTESIAN_POINT('Ctrl Pts',(6.26160116768587,138.727958979957,11.8619798975694));
#83191=CARTESIAN_POINT('Ctrl Pts',(6.26248606736094,138.743946714965,11.8590538346815));
#83192=CARTESIAN_POINT('Ctrl Pts',(6.26289995063702,138.75137574914,11.8577534507989));
#83193=CARTESIAN_POINT('Ctrl Pts',(6.26390376041198,138.769284295069,11.8547611980756));
#83194=CARTESIAN_POINT('Ctrl Pts',(6.26449662373628,138.779772705817,11.8531258324743));
#83195=CARTESIAN_POINT('Ctrl Pts',(6.26666758929046,138.817901695638,11.8476048940681));
#83196=CARTESIAN_POINT('Ctrl Pts',(6.26827632551352,138.845632915376,11.8443963614928));
#83197=CARTESIAN_POINT('Ctrl Pts',(6.27268950693175,138.920828653854,11.8378690112076));
#83198=CARTESIAN_POINT('Ctrl Pts',(6.27553469976765,138.968390696068,11.8360684402671));
#83199=CARTESIAN_POINT('Ctrl Pts',(6.28488460824947,139.124206895131,11.8377671044424));
#83200=CARTESIAN_POINT('Ctrl Pts',(6.29136819594589,139.232011520982,11.8509556525554));
#83201=CARTESIAN_POINT('Ctrl Pts',(6.29877276116309,139.359532179131,11.8811670544271));
#83202=CARTESIAN_POINT('Ctrl Pts',(6.30004325818092,139.38155552074,11.8869303695283));
#83203=CARTESIAN_POINT('Ctrl Pts',(6.30207853915382,139.417059412984,11.8971120691932));
#83204=CARTESIAN_POINT('Ctrl Pts',(6.3028531305527,139.43062531054,11.9012166136492));
#83205=CARTESIAN_POINT('Ctrl Pts',(6.30434486547773,139.456846794755,11.9095679150505));
#83206=CARTESIAN_POINT('Ctrl Pts',(6.30506265447024,139.469508073344,11.9137920206932));
#83207=CARTESIAN_POINT('Ctrl Pts',(6.30675423957324,139.499437623015,11.9242343577401));
#83208=CARTESIAN_POINT('Ctrl Pts',(6.30772293539835,139.516650382419,11.9306054389544));
#83209=CARTESIAN_POINT('Ctrl Pts',(6.31119487038767,139.578533603564,11.954843698852));
#83210=CARTESIAN_POINT('Ctrl Pts',(6.31363640017759,139.622437722751,11.974587443636));
#83211=CARTESIAN_POINT('Ctrl Pts',(6.32248788948386,139.780818738265,12.0554209057177));
#83212=CARTESIAN_POINT('Ctrl Pts',(6.3285183382369,139.887978107783,12.1294691105776));
#83213=CARTESIAN_POINT('Ctrl Pts',(6.33515505794404,139.983968635079,12.2166542679363));
#83214=CARTESIAN_POINT('',(6.3365,138.768242272558,11.854966918797));
#83215=CARTESIAN_POINT('Origin',(6.3365,139.,13.3));
#83216=CARTESIAN_POINT('Ctrl Pts',(6.3365,138.768242272558,11.854966918797));
#83217=CARTESIAN_POINT('Ctrl Pts',(6.333427091055,138.712441868313,11.8639163159052));
#83218=CARTESIAN_POINT('Ctrl Pts',(6.33035418211001,138.657111795352,11.8761099408742));
#83219=CARTESIAN_POINT('Ctrl Pts',(6.32728127316501,138.602642967625,11.8914760780085));
#83220=CARTESIAN_POINT('Ctrl Pts',(6.32421010161006,138.548204935994,11.9068335272924));
#83221=CARTESIAN_POINT('Ctrl Pts',(6.3211389300551,138.494627660216,11.9253597967244));
#83222=CARTESIAN_POINT('Ctrl Pts',(6.31806775850014,138.442289751673,11.9469325482774));
#83223=CARTESIAN_POINT('Ctrl Pts',(6.31499745988565,138.389966719498,11.9684991680571));
#83224=CARTESIAN_POINT('Ctrl Pts',(6.31192716127116,138.338882813531,11.9931103620133));
#83225=CARTESIAN_POINT('Ctrl Pts',(6.30885686265668,138.289397569585,12.0205952806525));
#83226=CARTESIAN_POINT('Ctrl Pts',(6.30578645390265,138.239910550476,12.0480811852466));
#83227=CARTESIAN_POINT('Ctrl Pts',(6.30271604514863,138.192022740535,12.0784407778119));
#83228=CARTESIAN_POINT('Ctrl Pts',(6.2996456363946,138.146068226617,12.1114577094582));
#83229=CARTESIAN_POINT('Ctrl Pts',(6.29657413458961,138.100097353109,12.1444863949758));
#83230=CARTESIAN_POINT('Ctrl Pts',(6.29350263278462,138.056061544296,12.1801740077873));
#83231=CARTESIAN_POINT('Ctrl Pts',(6.29043113097963,138.014263541637,12.2182625620544));
#83232=CARTESIAN_POINT('Ctrl Pts',(6.2873549864972,137.972402359902,12.2564086884418));
#83233=CARTESIAN_POINT('Ctrl Pts',(6.28427884201478,137.932786103428,12.2969626653084));
#83234=CARTESIAN_POINT('Ctrl Pts',(6.28120269753236,137.895681512845,12.3396287546333));
#83235=CARTESIAN_POINT('Ctrl Pts',(6.27812408406556,137.858547141263,12.3823290887437));
#83236=CARTESIAN_POINT('Ctrl Pts',(6.27504547059876,137.823928754659,12.4271445193177));
#83237=CARTESIAN_POINT('Ctrl Pts',(6.27196685713195,137.792051561807,12.4737477257723));
#83238=CARTESIAN_POINT('Ctrl Pts',(6.2688817646213,137.760107282348,12.5204490102162));
#83239=CARTESIAN_POINT('Ctrl Pts',(6.26579667211064,137.730915976882,12.5689451607239));
#83240=CARTESIAN_POINT('Ctrl Pts',(6.26271157959998,137.704658045929,12.6188821893213));
#83241=CARTESIAN_POINT('Ctrl Pts',(6.26089118497487,137.68916424916,12.6483481123491));
#83242=CARTESIAN_POINT('Ctrl Pts',(6.25907079034975,137.674690878593,12.6783152763757));
#83243=CARTESIAN_POINT('Ctrl Pts',(6.25725039572463,137.661267039855,12.7087079305276));
#83244=CARTESIAN_POINT('Ctrl Pts',(6.25400139029006,137.637308429776,12.7629521571078));
#83245=CARTESIAN_POINT('Ctrl Pts',(6.2507523848555,137.616608298453,12.8187501037437));
#83246=CARTESIAN_POINT('Ctrl Pts',(6.24750337942093,137.599354462676,12.8757072605205));
#83247=CARTESIAN_POINT('Ctrl Pts',(6.24426477152369,137.582155842998,12.9324821417746));
#83248=CARTESIAN_POINT('Ctrl Pts',(6.24102616362645,137.568381705114,12.9904084882188));
#83249=CARTESIAN_POINT('Ctrl Pts',(6.23778755572921,137.558172270461,13.0490716270891));
#83250=CARTESIAN_POINT('Ctrl Pts',(6.23456397913116,137.548010220693,13.1074624936685));
#83251=CARTESIAN_POINT('Ctrl Pts',(6.23134040253311,137.541380020528,13.1665829659533));
#83252=CARTESIAN_POINT('Ctrl Pts',(6.22811682593506,137.538371771148,13.2260056041077));
#83253=CARTESIAN_POINT('Ctrl Pts',(6.22679639588331,137.537139542671,13.2503460951079));
#83254=CARTESIAN_POINT('Ctrl Pts',(6.22547596583156,137.536514449846,13.2747370999646));
#83255=CARTESIAN_POINT('Ctrl Pts',(6.22415553577981,137.536500247676,13.2991485609046));
#83256=CARTESIAN_POINT('Origin',(6.3365,139.,13.3));
#83257=CARTESIAN_POINT('',(6.3365,140.003135769676,12.2343777040633));
#83258=CARTESIAN_POINT('',(6.3365,137.5365,13.3));
#83259=CARTESIAN_POINT('Origin',(6.3365,139.,13.3));
#83260=CARTESIAN_POINT('Ctrl Pts',(6.33650000000013,140.003135769676,12.2343777040634));
#83261=CARTESIAN_POINT('Ctrl Pts',(6.33650010571933,140.023669124737,12.2575147919222));
#83262=CARTESIAN_POINT('Ctrl Pts',(6.33649999999991,140.043388634716,12.281323949763));
#83263=CARTESIAN_POINT('Ctrl Pts',(6.33649999999995,140.062245685488,12.3057933133457));
#83264=CARTESIAN_POINT('Ctrl Pts',(6.33650000000002,140.097351486145,12.3513474464139));
#83265=CARTESIAN_POINT('Ctrl Pts',(6.33649999999986,140.129470426597,12.3991893725647));
#83266=CARTESIAN_POINT('Ctrl Pts',(6.33649999999998,140.158546998602,12.4489806897978));
#83267=CARTESIAN_POINT('Ctrl Pts',(6.33650000000002,140.168444534924,12.4659294336432));
#83268=CARTESIAN_POINT('Ctrl Pts',(6.33649999999992,140.177989140738,12.4831041762642));
#83269=CARTESIAN_POINT('Ctrl Pts',(6.33649999999992,140.187177335336,12.5004918282147));
#83270=CARTESIAN_POINT('Ctrl Pts',(6.33649999999991,140.193295770393,12.5120702964443));
#83271=CARTESIAN_POINT('Ctrl Pts',(6.33649999999975,140.199256942011,12.5237447867508));
#83272=CARTESIAN_POINT('Ctrl Pts',(6.33649999999976,140.205057168636,12.5355063710712));
#83273=CARTESIAN_POINT('Ctrl Pts',(6.33649999999984,140.230497025639,12.5870928077041));
#83274=CARTESIAN_POINT('Ctrl Pts',(6.3365000000001,140.252774622926,12.6402088612707));
#83275=CARTESIAN_POINT('Ctrl Pts',(6.33650000000003,140.271842328215,12.694511980783));
#83276=CARTESIAN_POINT('Ctrl Pts',(6.33649999999999,140.284881330078,12.7316458920614));
#83277=CARTESIAN_POINT('Ctrl Pts',(6.33649999999986,140.296418268899,12.7693353313234));
#83278=CARTESIAN_POINT('Ctrl Pts',(6.33649999999978,140.306423950697,12.8074719159752));
#83279=CARTESIAN_POINT('Ctrl Pts',(6.33649999999973,140.312377619302,12.8301642813083));
#83280=CARTESIAN_POINT('Ctrl Pts',(6.3365,140.317788915002,12.8530149598051));
#83281=CARTESIAN_POINT('Ctrl Pts',(6.33649999999981,140.322649755792,12.8760008063365));
#83282=CARTESIAN_POINT('Ctrl Pts',(6.33649999999971,140.325116583677,12.8876658926093));
#83283=CARTESIAN_POINT('Ctrl Pts',(6.33649999999987,140.32744178589,12.8993673010087));
#83284=CARTESIAN_POINT('Ctrl Pts',(6.3364999999999,140.329621093748,12.911083574289));
#83285=CARTESIAN_POINT('Ctrl Pts',(6.33650000000003,140.339905172661,12.9663722653945));
#83286=CARTESIAN_POINT('Ctrl Pts',(6.33650000000014,140.346964990818,13.02208316699));
#83287=CARTESIAN_POINT('Ctrl Pts',(6.33649999999991,140.35074615215,13.077899282583));
#83288=CARTESIAN_POINT('Ctrl Pts',(6.33649999999968,140.354434057332,13.1323387851239));
#83289=CARTESIAN_POINT('Ctrl Pts',(6.33650000000022,140.355002858764,13.1868794089901));
#83290=CARTESIAN_POINT('Ctrl Pts',(6.33650000000013,140.352354170508,13.2412187064025));
#83291=CARTESIAN_POINT('Ctrl Pts',(6.33650000000008,140.350787573337,13.2733583096162));
#83292=CARTESIAN_POINT('Ctrl Pts',(6.33650000000018,140.348094513887,13.3054272487336));
#83293=CARTESIAN_POINT('Ctrl Pts',(6.33650000000003,140.344246789072,13.3373593705737));
#83294=CARTESIAN_POINT('Ctrl Pts',(6.33649999999992,140.34158830054,13.3594220657457));
#83295=CARTESIAN_POINT('Ctrl Pts',(6.33650000000016,140.338378479852,13.3814193878785));
#83296=CARTESIAN_POINT('Ctrl Pts',(6.33649999999988,140.334606388925,13.4033284402217));
#83297=CARTESIAN_POINT('Ctrl Pts',(6.33649999999974,140.332808145722,13.413772993446));
#83298=CARTESIAN_POINT('Ctrl Pts',(6.3364999999999,140.330881741628,13.4241986892914));
#83299=CARTESIAN_POINT('Ctrl Pts',(6.33649999999994,140.328829643233,13.4345857047938));
#83300=CARTESIAN_POINT('Ctrl Pts',(6.33650000000012,140.318607036849,13.4863290184844));
#83301=CARTESIAN_POINT('Ctrl Pts',(6.33650000000002,140.305253098095,13.5372133729786));
#83302=CARTESIAN_POINT('Ctrl Pts',(6.3365000000001,140.288686037652,13.5869599067306));
#83303=CARTESIAN_POINT('Ctrl Pts',(6.33650000000012,140.285264455959,13.5972340184094));
#83304=CARTESIAN_POINT('Ctrl Pts',(6.33649999999969,140.281705658798,13.6074595259337));
#83305=CARTESIAN_POINT('Ctrl Pts',(6.33649999999975,140.278008672999,13.617633847654));
#83306=CARTESIAN_POINT('Ctrl Pts',(6.33650000000007,140.258790862416,13.6705223893568));
#83307=CARTESIAN_POINT('Ctrl Pts',(6.33650000000009,140.235842698297,13.7220312770223));
#83308=CARTESIAN_POINT('Ctrl Pts',(6.33650000000012,140.209434727541,13.7718972245888));
#83309=CARTESIAN_POINT('Ctrl Pts',(6.33650000000013,140.198177428881,13.7931542863272));
#83310=CARTESIAN_POINT('Ctrl Pts',(6.33649999999972,140.186290854219,13.8141122491807));
#83311=CARTESIAN_POINT('Ctrl Pts',(6.33649999999995,140.173793812567,13.8347480026074));
#83312=CARTESIAN_POINT('Ctrl Pts',(6.33650000000012,140.164796388131,13.8496050093537));
#83313=CARTESIAN_POINT('Ctrl Pts',(6.33649999999985,140.155482503734,13.8642949643968));
#83314=CARTESIAN_POINT('Ctrl Pts',(6.33649999999996,140.145858880467,13.8788086379537));
#83315=CARTESIAN_POINT('Ctrl Pts',(6.33650000000002,140.140281862567,13.8872195051469));
#83316=CARTESIAN_POINT('Ctrl Pts',(6.3365000000001,140.134605724196,13.8955637071506));
#83317=CARTESIAN_POINT('Ctrl Pts',(6.33650000000005,140.12883463953,13.9038364795333));
#83318=CARTESIAN_POINT('Ctrl Pts',(6.33649999999979,140.098780117204,13.9469192337569));
#83319=CARTESIAN_POINT('Ctrl Pts',(6.33649999999984,140.066133347015,13.9880983065987));
#83320=CARTESIAN_POINT('Ctrl Pts',(6.33649999999986,140.031132767185,14.0271737952641));
#83321=CARTESIAN_POINT('Ctrl Pts',(6.33649999999987,139.996314247044,14.0660460281165));
#83322=CARTESIAN_POINT('Ctrl Pts',(6.33650000000004,139.959165325295,14.1028371364767));
#83323=CARTESIAN_POINT('Ctrl Pts',(6.33650000000007,139.919892602426,14.1373077738618));
#83324=CARTESIAN_POINT('Ctrl Pts',(6.33650000000009,139.90024019132,14.1545571797462));
#83325=CARTESIAN_POINT('Ctrl Pts',(6.33649999999998,139.880055615327,14.1712247927656));
#83326=CARTESIAN_POINT('Ctrl Pts',(6.33650000000002,139.85936328841,14.1872758437228));
#83327=CARTESIAN_POINT('Ctrl Pts',(6.33650000000005,139.844113211276,14.1991053381126));
#83328=CARTESIAN_POINT('Ctrl Pts',(6.3364999999999,139.82858732605,14.2105998760627));
#83329=CARTESIAN_POINT('Ctrl Pts',(6.33649999999999,139.812795253445,14.2217443028877));
#83330=CARTESIAN_POINT('Ctrl Pts',(6.33650000000003,139.805156698168,14.2271348125736));
#83331=CARTESIAN_POINT('Ctrl Pts',(6.33650000000006,139.797456635723,14.2324427334948));
#83332=CARTESIAN_POINT('Ctrl Pts',(6.33650000000006,139.789706961736,14.2376594028882));
#83333=CARTESIAN_POINT('Ctrl Pts',(6.33650000000004,139.747876492251,14.2658174557627));
#83334=CARTESIAN_POINT('Ctrl Pts',(6.33649999999994,139.704520414613,14.2913790256126));
#83335=CARTESIAN_POINT('Ctrl Pts',(6.33649999999996,139.659834778768,14.3141386345366));
#83336=CARTESIAN_POINT('Ctrl Pts',(6.33649999999999,139.616041415194,14.3364437849408));
#83337=CARTESIAN_POINT('Ctrl Pts',(6.33649999999992,139.570970180933,14.3560581029554));
#83338=CARTESIAN_POINT('Ctrl Pts',(6.33649999999999,139.524795264372,14.3727395718669));
#83339=CARTESIAN_POINT('Ctrl Pts',(6.33650000000005,139.47862034781,14.3894210407783));
#83340=CARTESIAN_POINT('Ctrl Pts',(6.33650000000002,139.431340955144,14.4031701381045));
#83341=CARTESIAN_POINT('Ctrl Pts',(6.33649999999999,139.383133178262,14.4136893777957));
#83342=CARTESIAN_POINT('Ctrl Pts',(6.3365,138.079525356882,14.0347254547586));
#83343=CARTESIAN_POINT('Ctrl Pts',(6.3365,137.962361692323,13.9203814964881));
#83344=CARTESIAN_POINT('Ctrl Pts',(6.3364999999999,137.883433374858,13.7925889625522));
#83345=CARTESIAN_POINT('Ctrl Pts',(6.3364999999999,137.767824722722,13.5228369694544));
#83346=CARTESIAN_POINT('Ctrl Pts',(6.3364999999999,137.733244296092,13.3670757711572));
#83347=CARTESIAN_POINT('Ctrl Pts',(6.3364999999999,137.719950578003,13.0662072487722));
#83348=CARTESIAN_POINT('Ctrl Pts',(6.3364999999999,137.736602493462,12.9093813376879));
#83349=CARTESIAN_POINT('Ctrl Pts',(6.3364999999999,137.838995140157,12.6008328994218));
#83350=CARTESIAN_POINT('Ctrl Pts',(6.3364999999999,137.919392261343,12.4595666959715));
#83351=CARTESIAN_POINT('Ctrl Pts',(6.3364999999999,138.114949192507,12.2208706205168));
#83352=CARTESIAN_POINT('Ctrl Pts',(6.3364999999999,138.227112966334,12.1207931450485));
#83353=CARTESIAN_POINT('Ctrl Pts',(6.3364999999999,138.479316622589,11.9564560277444));
#83354=CARTESIAN_POINT('Ctrl Pts',(6.3365,138.620334945868,11.8931959685327));
#83355=CARTESIAN_POINT('Ctrl Pts',(6.3365,138.768242272558,11.854966918797));
#83356=CARTESIAN_POINT('Origin',(6.3365,139.,13.3));
#83357=CARTESIAN_POINT('Ctrl Pts',(1.89724981368824,138.491031839177,14.3596959507936));
#83358=CARTESIAN_POINT('Ctrl Pts',(1.92367413820389,138.139145735096,14.1906964941018));
#83359=CARTESIAN_POINT('Ctrl Pts',(1.97651499747799,137.623293427453,13.4770766030293));
#83360=CARTESIAN_POINT('Ctrl Pts',(2.05577239151056,138.103026646,12.2387996208986));
#83361=CARTESIAN_POINT('Ctrl Pts',(2.13502199578593,139.402779510252,11.971181393986));
#83362=CARTESIAN_POINT('Ctrl Pts',(2.21427160006131,140.334245953224,12.9149808566737));
#83363=CARTESIAN_POINT('Ctrl Pts',(2.29352120433668,140.048621811314,14.2106232938627));
#83364=CARTESIAN_POINT('Ctrl Pts',(2.37277080861206,138.805982047616,14.6750947012087));
#83365=CARTESIAN_POINT('Ctrl Pts',(2.45202041288743,137.740464633512,13.8849554560984));
#83366=CARTESIAN_POINT('Ctrl Pts',(2.5312700171628,137.824194363192,12.5610019680181));
#83367=CARTESIAN_POINT('Ctrl Pts',(2.61051962143818,138.980832587105,11.9113913495609));
#83368=CARTESIAN_POINT('Ctrl Pts',(2.68976922571355,140.154950676288,12.5288314630997));
#83369=CARTESIAN_POINT('Ctrl Pts',(2.76901882998892,140.275214890819,13.8499470203793));
#83370=CARTESIAN_POINT('Ctrl Pts',(2.8482684342643,139.231880590669,14.6692487692842));
#83371=CARTESIAN_POINT('Ctrl Pts',(2.92751803853967,137.976963165223,14.2391527366441));
#83372=CARTESIAN_POINT('Ctrl Pts',(3.00676764281505,137.655536323194,12.9521065933296));
#83373=CARTESIAN_POINT('Ctrl Pts',(3.08601724709042,138.560893438705,11.9825033575352));
#83374=CARTESIAN_POINT('Ctrl Pts',(3.16526685136579,139.866922293386,12.2150770092107));
#83375=CARTESIAN_POINT('Ctrl Pts',(3.24451645564117,140.381910028251,13.4376111754579));
#83376=CARTESIAN_POINT('Ctrl Pts',(3.32376605991654,139.635945339619,14.5345791356308));
#83377=CARTESIAN_POINT('Ctrl Pts',(3.40301566419192,138.309699184017,14.5050298433538));
#83378=CARTESIAN_POINT('Ctrl Pts',(3.48226526846729,137.613332281705,13.3759261313631));
#83379=CARTESIAN_POINT('Ctrl Pts',(3.56151487274267,138.182259029248,12.1775420548631));
#83380=CARTESIAN_POINT('Ctrl Pts',(3.64076447701804,139.497350441074,12.003367949123));
#83381=CARTESIAN_POINT('Ctrl Pts',(3.72001408129341,140.358624154713,13.0123325836223));
#83382=CARTESIAN_POINT('Ctrl Pts',(3.79926368556878,139.980193151235,14.2837853028199));
#83383=CARTESIAN_POINT('Ctrl Pts',(3.87851328984416,138.707364629187,14.657562770499));
#83384=CARTESIAN_POINT('Ctrl Pts',(3.95776289411953,137.701557305092,13.7926040032988));
#83385=CARTESIAN_POINT('Ctrl Pts',(4.03701249839491,137.880540879759,12.478158522525));
#83386=CARTESIAN_POINT('Ctrl Pts',(4.11626210267028,139.080998087674,11.9136192998211));
#83387=CARTESIAN_POINT('Ctrl Pts',(4.19551170694565,140.207546914827,12.6141118280076));
#83388=CARTESIAN_POINT('Ctrl Pts',(4.27476131122103,140.232244578235,13.9404572081215));
#83389=CARTESIAN_POINT('Ctrl Pts',(4.3540109154964,139.132555183917,14.682404159178));
#83390=CARTESIAN_POINT('Ctrl Pts',(4.43326051977178,137.911913069879,14.1629478363558));
#83391=CARTESIAN_POINT('Ctrl Pts',(4.51251012404715,137.684118384997,12.8560769081125));
#83392=CARTESIAN_POINT('Ctrl Pts',(4.59175972832253,138.657027102691,11.9542727883001));
#83393=CARTESIAN_POINT('Ctrl Pts',(4.6710093325979,139.942888534928,12.2804053037847));
#83394=CARTESIAN_POINT('Ctrl Pts',(4.75025893687327,140.368391819196,13.5368880907559));
#83395=CARTESIAN_POINT('Ctrl Pts',(4.82950854114865,139.545277675295,14.5772174430167));
#83396=CARTESIAN_POINT('Ctrl Pts',(4.90875814542402,138.224613644119,14.4521233077368));
#83397=CARTESIAN_POINT('Ctrl Pts',(4.9880077496994,137.611466917631,13.2757504441729));
#83398=CARTESIAN_POINT('Ctrl Pts',(5.06725735397477,138.265315962094,12.121504551065));
#83399=CARTESIAN_POINT('Ctrl Pts',(5.14650695825016,139.589542584736,12.0426012900189));
#83400=CARTESIAN_POINT('Ctrl Pts',(5.22575656252551,140.375829026531,13.1110373306486));
#83401=CARTESIAN_POINT('Ctrl Pts',(5.30500616680089,139.906711507075,14.3518966066086));
#83402=CARTESIAN_POINT('Ctrl Pts',(5.38425577107627,138.61024694163,14.6329303635249));
#83403=CARTESIAN_POINT('Ctrl Pts',(5.46350537535164,137.669419323723,13.6977056787498));
#83404=CARTESIAN_POINT('Ctrl Pts',(5.54275497962702,137.942710242223,12.3995832381271));
#83405=CARTESIAN_POINT('Ctrl Pts',(5.62200458390239,139.180741555268,11.9230708573093));
#83406=CARTESIAN_POINT('Ctrl Pts',(5.70125418817776,140.253862892755,12.7029532405301));
#83407=CARTESIAN_POINT('Ctrl Pts',(5.78050379245314,140.182847559272,14.0276495561597));
#83408=CARTESIAN_POINT('Ctrl Pts',(5.85975339672852,139.032567105703,14.6883327363301));
#83409=CARTESIAN_POINT('Ctrl Pts',(5.93900300100388,137.852469738973,14.0823150174432));
#83410=CARTESIAN_POINT('Ctrl Pts',(6.01825260527925,137.719667412237,12.762226377427));
#83411=CARTESIAN_POINT('Ctrl Pts',(6.09750220955463,138.754702766038,11.9333180733695));
#83412=CARTESIAN_POINT('Ctrl Pts',(6.17675181383001,140.014448367052,12.3504727739682));
#83413=CARTESIAN_POINT('Ctrl Pts',(6.25600804413745,140.34671451531,13.636171520518));
#83414=CARTESIAN_POINT('Ctrl Pts',(6.30884773968643,139.751301345624,14.2848551797266));
#83415=CARTESIAN_POINT('Ctrl Pts',(6.33527090047694,139.382151741646,14.4117392436421));
#83416=CARTESIAN_POINT('Ctrl Pts',(1.9531481975811,138.449114295271,14.4469702735566));
#83417=CARTESIAN_POINT('Ctrl Pts',(1.97957252209675,138.068247594067,14.2640523781665));
#83418=CARTESIAN_POINT('Ctrl Pts',(2.03241338137086,137.509910778712,13.4916602584589));
#83419=CARTESIAN_POINT('Ctrl Pts',(2.11167077540342,138.029153812998,12.1514013965941));
#83420=CARTESIAN_POINT('Ctrl Pts',(2.19092037967879,139.435951580932,11.8617426971333));
#83421=CARTESIAN_POINT('Ctrl Pts',(2.27016998395417,140.444131634942,12.8832714923419));
#83422=CARTESIAN_POINT('Ctrl Pts',(2.34941958822954,140.134984091314,14.2856203071142));
#83423=CARTESIAN_POINT('Ctrl Pts',(2.42866919250492,138.790003138397,14.7883445996285));
#83424=CARTESIAN_POINT('Ctrl Pts',(2.50791879678029,137.636731958093,13.933131153325));
#83425=CARTESIAN_POINT('Ctrl Pts',(2.58716840105567,137.727357491656,12.5001396492404));
#83426=CARTESIAN_POINT('Ctrl Pts',(2.66641800533104,138.979253999418,11.7970284707942));
#83427=CARTESIAN_POINT('Ctrl Pts',(2.74566760960641,140.250069977274,12.4653196494102));
#83428=CARTESIAN_POINT('Ctrl Pts',(2.82491721388179,140.380238898782,13.8952394967008));
#83429=CARTESIAN_POINT('Ctrl Pts',(2.90416681815716,139.250977786895,14.7820172090845));
#83430=CARTESIAN_POINT('Ctrl Pts',(2.98341642243253,137.892708009911,14.3164993746116));
#83431=CARTESIAN_POINT('Ctrl Pts',(3.06266602670791,137.544809131318,12.9234548263411));
#83432=CARTESIAN_POINT('Ctrl Pts',(3.14191563098328,138.524729548743,11.8739971137133));
#83433=CARTESIAN_POINT('Ctrl Pts',(3.22116523525866,139.938320184439,12.1257250406574));
#83434=CARTESIAN_POINT('Ctrl Pts',(3.30041483953403,140.495721222627,13.4489445415368));
#83435=CARTESIAN_POINT('Ctrl Pts',(3.3796644438094,139.688320456074,14.6362564685289));
#83436=CARTESIAN_POINT('Ctrl Pts',(3.45891404808478,138.252847465207,14.6042735588831));
#83437=CARTESIAN_POINT('Ctrl Pts',(3.53816365236015,137.499129254014,13.3821792473534));
#83438=CARTESIAN_POINT('Ctrl Pts',(3.61741325663553,138.114911608165,12.0850987866609));
#83439=CARTESIAN_POINT('Ctrl Pts',(3.6966628609109,139.538311174092,11.8965800690441));
#83440=CARTESIAN_POINT('Ctrl Pts',(3.77591246518627,140.470517573672,12.9886409021295));
#83441=CARTESIAN_POINT('Ctrl Pts',(3.85516206946165,140.060919791161,14.3648077847721));
#83442=CARTESIAN_POINT('Ctrl Pts',(3.93441167373702,138.683263797448,14.7693687760942));
#83443=CARTESIAN_POINT('Ctrl Pts',(4.01366127801239,137.594620304191,13.8331738297156));
#83444=CARTESIAN_POINT('Ctrl Pts',(4.09291088228777,137.788344588448,12.4104733923595));
#83445=CARTESIAN_POINT('Ctrl Pts',(4.17216048656314,139.087668919285,11.7994399103375));
#83446=CARTESIAN_POINT('Ctrl Pts',(4.25141009083852,140.306997931053,12.5576235252477));
#83447=CARTESIAN_POINT('Ctrl Pts',(4.33065969511389,140.333729641912,13.9932039125471));
#83448=CARTESIAN_POINT('Ctrl Pts',(4.40990929938927,139.1434721492,14.7962560491346));
#83449=CARTESIAN_POINT('Ctrl Pts',(4.48915890366464,137.822300525957,14.2340183995126));
#83450=CARTESIAN_POINT('Ctrl Pts',(4.56840850794001,137.57574515143,12.8195163388526));
#83451=CARTESIAN_POINT('Ctrl Pts',(4.64765811221539,138.628780578472,11.8434415343569));
#83452=CARTESIAN_POINT('Ctrl Pts',(4.72690771649076,140.02054284536,12.1964336357431));
#83453=CARTESIAN_POINT('Ctrl Pts',(4.80615732076614,140.481089682396,13.5563976941245));
#83454=CARTESIAN_POINT('Ctrl Pts',(4.88540692504151,139.590185594206,14.6824063769528));
#83455=CARTESIAN_POINT('Ctrl Pts',(4.96465652931688,138.160754459757,14.5470097526149));
#83456=CARTESIAN_POINT('Ctrl Pts',(5.04390613359226,137.49711026249,13.2737533019168));
#83457=CARTESIAN_POINT('Ctrl Pts',(5.12315573786763,138.204808934767,12.0244461522779));
#83458=CARTESIAN_POINT('Ctrl Pts',(5.202405342143,139.638096068199,11.939044585122));
#83459=CARTESIAN_POINT('Ctrl Pts',(5.28165494641838,140.489139402435,13.0954747638737));
#83460=CARTESIAN_POINT('Ctrl Pts',(5.36090455069375,139.98138635382,14.4385285918397));
#83461=CARTESIAN_POINT('Ctrl Pts',(5.44015415496912,138.578147702043,14.7427076960513));
#83462=CARTESIAN_POINT('Ctrl Pts',(5.5194037592445,137.55983550648,13.7304598793731));
#83463=CARTESIAN_POINT('Ctrl Pts',(5.59865336351987,137.85563408844,12.3254268133166));
#83464=CARTESIAN_POINT('Ctrl Pts',(5.67790296779525,139.195627048432,11.8096698781595));
#83465=CARTESIAN_POINT('Ctrl Pts',(5.75715257207062,140.357128395206,12.6537817290681));
#83466=CARTESIAN_POINT('Ctrl Pts',(5.836402176346,140.280264388684,14.0875772384116));
#83467=CARTESIAN_POINT('Ctrl Pts',(5.91565178062137,139.035249263818,14.8026728913928));
#83468=CARTESIAN_POINT('Ctrl Pts',(5.99490138489674,137.757961567731,14.1467448317533));
#83469=CARTESIAN_POINT('Ctrl Pts',(6.07415098917212,137.614221921552,12.7179364764654));
#83470=CARTESIAN_POINT('Ctrl Pts',(6.1534005934475,138.734500603377,11.8207610333147));
#83471=CARTESIAN_POINT('Ctrl Pts',(6.23265019772286,140.097996194282,12.2722717149427));
#83472=CARTESIAN_POINT('Ctrl Pts',(6.31190642803031,140.457627081495,13.6638578976939));
#83473=CARTESIAN_POINT('Ctrl Pts',(6.36474612357929,139.813176939356,14.3659657744835));
#83474=CARTESIAN_POINT('Ctrl Pts',(6.39116928436981,139.413624952825,14.5032997422034));
#83475=CARTESIAN_POINT('Ctrl Pts',(2.00904658147396,138.407196751365,14.5342445963199));
#83476=CARTESIAN_POINT('Ctrl Pts',(2.03547090598961,137.997349453038,14.3374082622313));
#83477=CARTESIAN_POINT('Ctrl Pts',(2.08831176526372,137.396528129969,13.5062439138887));
#83478=CARTESIAN_POINT('Ctrl Pts',(2.16756915929628,137.955280979994,12.0640031722895));
#83479=CARTESIAN_POINT('Ctrl Pts',(2.24681876357166,139.469123651614,11.7523040002805));
#83480=CARTESIAN_POINT('Ctrl Pts',(2.32606836784703,140.55401731666,12.8515621280101));
#83481=CARTESIAN_POINT('Ctrl Pts',(2.4053179721224,140.221346371314,14.3606173203656));
#83482=CARTESIAN_POINT('Ctrl Pts',(2.48456757639778,138.774024229176,14.9015944980482));
#83483=CARTESIAN_POINT('Ctrl Pts',(2.56381718067315,137.532999282673,13.9813068505515));
#83484=CARTESIAN_POINT('Ctrl Pts',(2.64306678494853,137.630520620122,12.4392773304629));
#83485=CARTESIAN_POINT('Ctrl Pts',(2.7223163892239,138.977675411732,11.6826655920275));
#83486=CARTESIAN_POINT('Ctrl Pts',(2.80156599349928,140.345189278261,12.4018078357209));
#83487=CARTESIAN_POINT('Ctrl Pts',(2.88081559777465,140.485262906743,13.940531973022));
#83488=CARTESIAN_POINT('Ctrl Pts',(2.96006520205002,139.270074983123,14.8947856488846));
#83489=CARTESIAN_POINT('Ctrl Pts',(3.0393148063254,137.8084528546,14.3938460125793));
#83490=CARTESIAN_POINT('Ctrl Pts',(3.11856441060077,137.434081939444,12.8948030593524));
#83491=CARTESIAN_POINT('Ctrl Pts',(3.19781401487614,138.48856565878,11.7654908698915));
#83492=CARTESIAN_POINT('Ctrl Pts',(3.27706361915152,140.009718075492,12.0363730721043));
#83493=CARTESIAN_POINT('Ctrl Pts',(3.35631322342689,140.609532417002,13.4602779076157));
#83494=CARTESIAN_POINT('Ctrl Pts',(3.43556282770226,139.740695572528,14.7379338014271));
#83495=CARTESIAN_POINT('Ctrl Pts',(3.51481243197764,138.195995746398,14.7035172744123));
#83496=CARTESIAN_POINT('Ctrl Pts',(3.59406203625301,137.384926226324,13.3884323633436));
#83497=CARTESIAN_POINT('Ctrl Pts',(3.67331164052839,138.047564187082,11.9926555184588));
#83498=CARTESIAN_POINT('Ctrl Pts',(3.75256124480376,139.57927190711,11.7897921889655));
#83499=CARTESIAN_POINT('Ctrl Pts',(3.83181084907914,140.582410992633,12.9649492206368));
#83500=CARTESIAN_POINT('Ctrl Pts',(3.91106045335451,140.141646431087,14.4458302667241));
#83501=CARTESIAN_POINT('Ctrl Pts',(3.99031005762989,138.659162965709,14.8811747816896));
#83502=CARTESIAN_POINT('Ctrl Pts',(4.06955966190525,137.48768330329,13.8737436561324));
#83503=CARTESIAN_POINT('Ctrl Pts',(4.14880926618063,137.696148297138,12.3427882621941));
#83504=CARTESIAN_POINT('Ctrl Pts',(4.228058870456,139.094339750897,11.6852605208537));
#83505=CARTESIAN_POINT('Ctrl Pts',(4.30730847473138,140.406448947278,12.5011352224877));
#83506=CARTESIAN_POINT('Ctrl Pts',(4.38655807900675,140.435214705589,14.0459506169728));
#83507=CARTESIAN_POINT('Ctrl Pts',(4.46580768328213,139.154389114483,14.9101079390912));
#83508=CARTESIAN_POINT('Ctrl Pts',(4.5450572875575,137.732687982037,14.3050889626694));
#83509=CARTESIAN_POINT('Ctrl Pts',(4.62430689183287,137.467371917862,12.7829557695927));
#83510=CARTESIAN_POINT('Ctrl Pts',(4.70355649610825,138.600534054253,11.7326102804137));
#83511=CARTESIAN_POINT('Ctrl Pts',(4.78280610038362,140.098197155792,12.1124619677015));
#83512=CARTESIAN_POINT('Ctrl Pts',(4.862055704659,140.593787545595,13.5759072974933));
#83513=CARTESIAN_POINT('Ctrl Pts',(4.94130530893437,139.635093513118,14.7875953108892));
#83514=CARTESIAN_POINT('Ctrl Pts',(5.02055491320974,138.096895275395,14.6418961974928));
#83515=CARTESIAN_POINT('Ctrl Pts',(5.09980451748512,137.382753607351,13.2717561596606));
#83516=CARTESIAN_POINT('Ctrl Pts',(5.17905412176049,138.14430190744,11.9273877534907));
#83517=CARTESIAN_POINT('Ctrl Pts',(5.25830372603587,139.686649551662,11.835487880225));
#83518=CARTESIAN_POINT('Ctrl Pts',(5.33755333031124,140.60244977834,13.0799121970989));
#83519=CARTESIAN_POINT('Ctrl Pts',(5.41680293458661,140.056061200564,14.5251605770708));
#83520=CARTESIAN_POINT('Ctrl Pts',(5.49605253886199,138.546048462455,14.8524850285775));
#83521=CARTESIAN_POINT('Ctrl Pts',(5.57530214313737,137.45025168924,13.7632140799964));
#83522=CARTESIAN_POINT('Ctrl Pts',(5.65455174741274,137.768557934658,12.251270388506));
#83523=CARTESIAN_POINT('Ctrl Pts',(5.73380135168811,139.210512541595,11.6962688990097));
#83524=CARTESIAN_POINT('Ctrl Pts',(5.81305095596348,140.460393897656,12.6046102176062));
#83525=CARTESIAN_POINT('Ctrl Pts',(5.89230056023886,140.377681218095,14.1475049206634));
#83526=CARTESIAN_POINT('Ctrl Pts',(5.97155016451423,139.037931421934,14.9170130464555));
#83527=CARTESIAN_POINT('Ctrl Pts',(6.05079976878961,137.663453396491,14.2111746460634));
#83528=CARTESIAN_POINT('Ctrl Pts',(6.13004937306498,137.508776430867,12.673646575504));
#83529=CARTESIAN_POINT('Ctrl Pts',(6.20929897734035,138.714298440715,11.70820399326));
#83530=CARTESIAN_POINT('Ctrl Pts',(6.28854858161573,140.181544021511,12.1940706559173));
#83531=CARTESIAN_POINT('Ctrl Pts',(6.36780481192318,140.56853964768,13.6915442748698));
#83532=CARTESIAN_POINT('Ctrl Pts',(6.42064450747215,139.875052533088,14.4470763692405));
#83533=CARTESIAN_POINT('Ctrl Pts',(6.44706766826268,139.445098164004,14.5948602407648));
#83534=CARTESIAN_POINT('Ctrl Pts',(2.06494496536683,138.36527920746,14.621518919083));
#83535=CARTESIAN_POINT('Ctrl Pts',(2.09136928988247,137.926451312009,14.4107641462959));
#83536=CARTESIAN_POINT('Ctrl Pts',(2.14421014915659,137.283145481227,13.5208275693184));
#83537=CARTESIAN_POINT('Ctrl Pts',(2.22346754318915,137.881408146991,11.976604947985));
#83538=CARTESIAN_POINT('Ctrl Pts',(2.30271714746453,139.502295722294,11.6428653034279));
#83539=CARTESIAN_POINT('Ctrl Pts',(2.3819667517399,140.663902998379,12.8198527636783));
#83540=CARTESIAN_POINT('Ctrl Pts',(2.46121635601528,140.307708651313,14.4356143336172));
#83541=CARTESIAN_POINT('Ctrl Pts',(2.54046596029065,138.758045319957,15.014844396468));
#83542=CARTESIAN_POINT('Ctrl Pts',(2.61971556456603,137.429266607254,14.0294825477779));
#83543=CARTESIAN_POINT('Ctrl Pts',(2.6989651688414,137.533683748586,12.3784150116853));
#83544=CARTESIAN_POINT('Ctrl Pts',(2.77821477311677,138.976096824046,11.5683027132609));
#83545=CARTESIAN_POINT('Ctrl Pts',(2.85746437739215,140.440308579247,12.3382960220315));
#83546=CARTESIAN_POINT('Ctrl Pts',(2.93671398166752,140.590286914707,13.9858244493435));
#83547=CARTESIAN_POINT('Ctrl Pts',(3.0159635859429,139.289172179348,15.0075540886847));
#83548=CARTESIAN_POINT('Ctrl Pts',(3.09521319021827,137.724197699289,14.4711926505468));
#83549=CARTESIAN_POINT('Ctrl Pts',(3.17446279449364,137.323354747568,12.8661512923638));
#83550=CARTESIAN_POINT('Ctrl Pts',(3.25371239876901,138.452401768818,11.6569846260696));
#83551=CARTESIAN_POINT('Ctrl Pts',(3.33296200304439,140.081115966545,11.9470211035511));
#83552=CARTESIAN_POINT('Ctrl Pts',(3.41221160731976,140.72334361138,13.4716112736946));
#83553=CARTESIAN_POINT('Ctrl Pts',(3.49146121159514,139.793070688983,14.8396111343253));
#83554=CARTESIAN_POINT('Ctrl Pts',(3.57071081587051,138.139144027589,14.8027609899417));
#83555=CARTESIAN_POINT('Ctrl Pts',(3.64996042014589,137.270723198634,13.3946854793339));
#83556=CARTESIAN_POINT('Ctrl Pts',(3.72921002442126,137.980216765998,11.9002122502566));
#83557=CARTESIAN_POINT('Ctrl Pts',(3.80845962869663,139.620232640128,11.6830043088867));
#83558=CARTESIAN_POINT('Ctrl Pts',(3.88770923297201,140.694304411592,12.941257539144));
#83559=CARTESIAN_POINT('Ctrl Pts',(3.96695883724738,140.222373071014,14.5268527486763));
#83560=CARTESIAN_POINT('Ctrl Pts',(4.04620844152276,138.63506213397,14.9929807872849));
#83561=CARTESIAN_POINT('Ctrl Pts',(4.12545804579813,137.380746302389,13.9143134825491));
#83562=CARTESIAN_POINT('Ctrl Pts',(4.2047076500735,137.603952005827,12.2751031320286));
#83563=CARTESIAN_POINT('Ctrl Pts',(4.28395725434888,139.101010582507,11.57108113137));
#83564=CARTESIAN_POINT('Ctrl Pts',(4.36320685862425,140.505899963503,12.4446469197279));
#83565=CARTESIAN_POINT('Ctrl Pts',(4.44245646289962,140.536699769265,14.0986973213983));
#83566=CARTESIAN_POINT('Ctrl Pts',(4.521706067175,139.165306079766,15.0239598290478));
#83567=CARTESIAN_POINT('Ctrl Pts',(4.60095567145037,137.643075438114,14.3761595258263));
#83568=CARTESIAN_POINT('Ctrl Pts',(4.68020527572575,137.358998684294,12.7463952003328));
#83569=CARTESIAN_POINT('Ctrl Pts',(4.75945488000112,138.572287530034,11.6217790264705));
#83570=CARTESIAN_POINT('Ctrl Pts',(4.8387044842765,140.175851466226,12.02849029966));
#83571=CARTESIAN_POINT('Ctrl Pts',(4.91795408855187,140.706485408794,13.595416900862));
#83572=CARTESIAN_POINT('Ctrl Pts',(4.99720369282725,139.68000143203,14.8927842448254));
#83573=CARTESIAN_POINT('Ctrl Pts',(5.07645329710261,138.033036091033,14.7367826423707));
#83574=CARTESIAN_POINT('Ctrl Pts',(5.15570290137799,137.268396952211,13.2697590174042));
#83575=CARTESIAN_POINT('Ctrl Pts',(5.23495250565336,138.083794880113,11.8303293547037));
#83576=CARTESIAN_POINT('Ctrl Pts',(5.31420210992873,139.735203035125,11.7319311753281));
#83577=CARTESIAN_POINT('Ctrl Pts',(5.39345171420411,140.715760154244,13.0643496303242));
#83578=CARTESIAN_POINT('Ctrl Pts',(5.47270131847949,140.130736047309,14.6117925623019));
#83579=CARTESIAN_POINT('Ctrl Pts',(5.55195092275486,138.513949222868,14.9622623611039));
#83580=CARTESIAN_POINT('Ctrl Pts',(5.63120052703023,137.340667871997,13.7959682806195));
#83581=CARTESIAN_POINT('Ctrl Pts',(5.71045013130561,137.681481780874,12.1771139636956));
#83582=CARTESIAN_POINT('Ctrl Pts',(5.78969973558099,139.225398034759,11.5828679198597));
#83583=CARTESIAN_POINT('Ctrl Pts',(5.86894933985634,140.563659400107,12.5554387061441));
#83584=CARTESIAN_POINT('Ctrl Pts',(5.94819894413173,140.475098047509,14.2074326029153));
#83585=CARTESIAN_POINT('Ctrl Pts',(6.02744854840711,139.040613580049,15.0313532015183));
#83586=CARTESIAN_POINT('Ctrl Pts',(6.10669815268248,137.568945225249,14.2756044603734));
#83587=CARTESIAN_POINT('Ctrl Pts',(6.18594775695784,137.403330940182,12.6293566745424));
#83588=CARTESIAN_POINT('Ctrl Pts',(6.26519736123323,138.694096278053,11.5956469532053));
#83589=CARTESIAN_POINT('Ctrl Pts',(6.34444696550859,140.265091848741,12.1158695968918));
#83590=CARTESIAN_POINT('Ctrl Pts',(6.42370319581604,140.679452213867,13.7192306520457));
#83591=CARTESIAN_POINT('Ctrl Pts',(6.47654289136502,139.936928126819,14.5281869639975));
#83592=CARTESIAN_POINT('Ctrl Pts',(6.50296605215554,139.476571375183,14.6864207393261));
#83593=CARTESIAN_POINT('Ctrl Pts',(6.33564735913931,139.984553534226,12.2160336743987));
#83594=CARTESIAN_POINT('Ctrl Pts',(6.3357883151664,139.987674636155,12.2190589540515));
#83595=CARTESIAN_POINT('Ctrl Pts',(6.33592973903903,139.990781924426,12.2220984365611));
#83596=CARTESIAN_POINT('Ctrl Pts',(6.33621393093556,139.996976184895,12.2282131236378));
#83597=CARTESIAN_POINT('Ctrl Pts',(6.33635670003917,140.000063059071,12.2312883679801));
#83598=CARTESIAN_POINT('Ctrl Pts',(6.33650000000001,140.003135769676,12.2343777040635));
#83599=CARTESIAN_POINT('',(2.06296787020315,138.314392290401,12.3412366180523));
#83600=CARTESIAN_POINT('Ctrl Pts',(2.06350000000003,138.31381039713,12.3405101317741));
#83601=CARTESIAN_POINT('Ctrl Pts',(2.06349999999999,138.285458471108,12.3559164614661));
#83602=CARTESIAN_POINT('Ctrl Pts',(2.06349999999991,138.257842156157,12.372524187337));
#83603=CARTESIAN_POINT('Ctrl Pts',(2.06349999999993,138.231048120938,12.3903151986867));
#83604=CARTESIAN_POINT('Ctrl Pts',(2.06349999999997,138.190824387068,12.4170234156452));
#83605=CARTESIAN_POINT('Ctrl Pts',(2.06350000000012,138.15245237466,12.4463958230688));
#83606=CARTESIAN_POINT('Ctrl Pts',(2.0635,138.116003297166,12.4781362863144));
#83607=CARTESIAN_POINT('Ctrl Pts',(2.06349999999994,138.097947361144,12.4938596958785));
#83608=CARTESIAN_POINT('Ctrl Pts',(2.06350000000003,138.080363580768,12.5101649876866));
#83609=CARTESIAN_POINT('Ctrl Pts',(2.06349999999992,138.063262566106,12.5270202810066));
#83610=CARTESIAN_POINT('Ctrl Pts',(2.06349999999987,138.055307674324,12.5348608704087));
#83611=CARTESIAN_POINT('Ctrl Pts',(2.06350000000001,138.047460879066,12.542817048106));
#83612=CARTESIAN_POINT('Ctrl Pts',(2.06350000000004,138.039728403076,12.5508795988707));
#83613=CARTESIAN_POINT('Ctrl Pts',(2.06350000000019,138.004683647871,12.5874203030686));
#83614=CARTESIAN_POINT('Ctrl Pts',(2.06350000000007,137.97195072146,12.6261758296458));
#83615=CARTESIAN_POINT('Ctrl Pts',(2.06350000000008,137.941609469643,12.6668229112449));
#83616=CARTESIAN_POINT('Ctrl Pts',(2.06350000000009,137.920229233239,12.6954652434387));
#83617=CARTESIAN_POINT('Ctrl Pts',(2.06350000000024,137.900036955561,12.725047988167));
#83618=CARTESIAN_POINT('Ctrl Pts',(2.06349999999998,137.881068772353,12.7554710709598));
#83619=CARTESIAN_POINT('Ctrl Pts',(2.06349999999989,137.874172837461,12.766531465931));
#83620=CARTESIAN_POINT('Ctrl Pts',(2.06349999999995,137.867438766385,12.777703018237));
#83621=CARTESIAN_POINT('Ctrl Pts',(2.06349999999992,137.860868566423,12.7889812037336));
#83622=CARTESIAN_POINT('Ctrl Pts',(2.0634999999999,137.855417684603,12.7983380051462));
#83623=CARTESIAN_POINT('Ctrl Pts',(2.06350000000018,137.850083786557,12.8077610883057));
#83624=CARTESIAN_POINT('Ctrl Pts',(2.06350000000015,137.844869690817,12.8172435416598));
#83625=CARTESIAN_POINT('Ctrl Pts',(2.06349999999998,137.819549238928,12.863291795451));
#83626=CARTESIAN_POINT('Ctrl Pts',(2.06350000000024,137.797034877009,12.9107653736245));
#83627=CARTESIAN_POINT('Ctrl Pts',(2.06350000000017,137.777411572447,12.9593365650308));
#83628=CARTESIAN_POINT('Ctrl Pts',(2.06350000000009,137.757448351045,13.0087491114608));
#83629=CARTESIAN_POINT('Ctrl Pts',(2.06350000000017,137.740476446572,13.0592985264396));
#83630=CARTESIAN_POINT('Ctrl Pts',(2.06350000000001,137.72662193392,13.1106779323383));
#83631=CARTESIAN_POINT('Ctrl Pts',(2.06349999999992,137.718765064424,13.1398151020845));
#83632=CARTESIAN_POINT('Ctrl Pts',(2.06350000000036,137.711911474736,13.1692198144023));
#83633=CARTESIAN_POINT('Ctrl Pts',(2.06350000000024,137.706090714823,13.1988396596195));
#83634=CARTESIAN_POINT('Ctrl Pts',(2.06350000000017,137.702885402907,13.2151503895351));
#83635=CARTESIAN_POINT('Ctrl Pts',(2.06350000000025,137.699993372106,13.2315263917338));
#83636=CARTESIAN_POINT('Ctrl Pts',(2.06350000000008,137.697420260214,13.2479591140196));
#83637=CARTESIAN_POINT('Ctrl Pts',(2.06349999999997,137.695935004121,13.2574444383731));
#83638=CARTESIAN_POINT('Ctrl Pts',(2.06350000000016,137.694556261355,13.2669477366054));
#83639=CARTESIAN_POINT('Ctrl Pts',(2.06350000000011,137.693286568647,13.2764543915575));
#83640=CARTESIAN_POINT('Ctrl Pts',(2.06349999999986,137.686032340524,13.3307694579084));
#83641=CARTESIAN_POINT('Ctrl Pts',(2.0635000000002,137.682316399564,13.3853020607817));
#83642=CARTESIAN_POINT('Ctrl Pts',(2.06349999999998,137.682252389277,13.4397235925187));
#83643=CARTESIAN_POINT('Ctrl Pts',(2.06349999999994,137.682241271235,13.4491761492556));
#83644=CARTESIAN_POINT('Ctrl Pts',(2.06349999999988,137.682340435788,13.4586254213502));
#83645=CARTESIAN_POINT('Ctrl Pts',(2.06349999999989,137.682550620444,13.4680697618261));
#83646=CARTESIAN_POINT('Ctrl Pts',(2.06349999999994,137.683718804571,13.5205604092094));
#83647=CARTESIAN_POINT('Ctrl Pts',(2.06350000000034,137.688312171862,13.5728980536096));
#83648=CARTESIAN_POINT('Ctrl Pts',(2.0635000000001,137.696128834035,13.6248637376689));
#83649=CARTESIAN_POINT('Ctrl Pts',(2.06349999999998,137.700124807928,13.6514292348389));
#83650=CARTESIAN_POINT('Ctrl Pts',(2.06349999999988,137.704963995215,13.6778976645399));
#83651=CARTESIAN_POINT('Ctrl Pts',(2.06350000000013,137.710624501111,13.7042400680577));
#83652=CARTESIAN_POINT('Ctrl Pts',(2.06350000000029,137.714078239673,13.7203127966335));
#83653=CARTESIAN_POINT('Ctrl Pts',(2.06349999999984,137.717837803142,13.7363386079794));
#83654=CARTESIAN_POINT('Ctrl Pts',(2.0634999999999,137.721898811607,13.7523108670406));
#83655=CARTESIAN_POINT('Ctrl Pts',(2.06349999999993,137.724577776208,13.7628474411447));
#83656=CARTESIAN_POINT('Ctrl Pts',(2.0635,137.727388445803,13.7733621159339));
#83657=CARTESIAN_POINT('Ctrl Pts',(2.06350000000002,137.730324276325,13.7838350181237));
#83658=CARTESIAN_POINT('Ctrl Pts',(2.06350000000014,137.745127646236,13.8366426458083));
#83659=CARTESIAN_POINT('Ctrl Pts',(2.06350000000013,137.76313364273,13.8884900800757));
#83660=CARTESIAN_POINT('Ctrl Pts',(2.06350000000001,137.784102793348,13.9391405178824));
#83661=CARTESIAN_POINT('Ctrl Pts',(2.06349999999989,137.805528956221,13.9908948569041));
#83662=CARTESIAN_POINT('Ctrl Pts',(2.06350000000002,137.830049059367,14.0414004131965));
#83663=CARTESIAN_POINT('Ctrl Pts',(2.06349999999993,137.857462565103,14.090404990338));
#83664=CARTESIAN_POINT('Ctrl Pts',(2.06349999999988,137.8728625944,14.1179341918534));
#83665=CARTESIAN_POINT('Ctrl Pts',(2.06349999999982,137.88917669756,14.1449896367826));
#83666=CARTESIAN_POINT('Ctrl Pts',(2.06349999999995,137.906376242815,14.1715248807554));
#83667=CARTESIAN_POINT('Ctrl Pts',(2.06350000000004,137.917641306872,14.1889044811272));
#83668=CARTESIAN_POINT('Ctrl Pts',(2.06349999999991,137.929286303867,14.2060608964028));
#83669=CARTESIAN_POINT('Ctrl Pts',(2.06349999999999,137.941304251294,14.222980560379));
#83670=CARTESIAN_POINT('Ctrl Pts',(2.06350000000003,137.947363355696,14.2315109696768));
#83671=CARTESIAN_POINT('Ctrl Pts',(2.06350000000009,137.953518778308,14.2399832102723));
#83672=CARTESIAN_POINT('Ctrl Pts',(2.06350000000006,137.959764791964,14.2483889110011));
#83673=CARTESIAN_POINT('Ctrl Pts',(2.0634999999999,137.994493741366,14.2951261055335));
#83674=CARTESIAN_POINT('Ctrl Pts',(2.06350000000023,138.031910482614,14.3396636613191));
#83675=CARTESIAN_POINT('Ctrl Pts',(2.0635000000002,138.071787386868,14.3817421533142));
#83676=CARTESIAN_POINT('Ctrl Pts',(2.06350000000016,138.111761295662,14.42392300543));
#83677=CARTESIAN_POINT('Ctrl Pts',(2.06349999999991,138.154207834877,14.46363388879));
#83678=CARTESIAN_POINT('Ctrl Pts',(2.06350000000003,138.198946759824,14.500595934106));
#83679=CARTESIAN_POINT('Ctrl Pts',(2.06350000000015,138.24264340849,14.536696879984));
#83680=CARTESIAN_POINT('Ctrl Pts',(2.06349999999996,138.288527497966,14.5701764701555));
#83681=CARTESIAN_POINT('Ctrl Pts',(2.06349999999993,138.336469361946,14.6007438022739));
#83682=CARTESIAN_POINT('Ctrl Pts',(2.06349999999992,138.346225523483,14.606964249398));
#83683=CARTESIAN_POINT('Ctrl Pts',(2.06350000000002,138.356067013842,14.6130639630822));
#83684=CARTESIAN_POINT('Ctrl Pts',(2.06350000000003,138.365992905425,14.6190402776369));
#83685=CARTESIAN_POINT('Ctrl Pts',(2.06296787020315,138.314932905069,12.3419926211435));
#83686=CARTESIAN_POINT('Ctrl Pts',(2.06314524680209,138.318975915862,12.3391014809294));
#83687=CARTESIAN_POINT('Ctrl Pts',(2.06332262340104,138.323037228809,12.3362359347072));
#83688=CARTESIAN_POINT('Ctrl Pts',(2.06349999999998,138.327116518419,12.3333962121349));
#83689=CARTESIAN_POINT('Origin',(2.0635,139.,13.3));
#83690=CARTESIAN_POINT('',(2.0635,137.5365,13.3));
#83691=CARTESIAN_POINT('Origin',(2.0635,139.,13.3));
#83692=CARTESIAN_POINT('',(2.0635,139.657803339705,14.6073358467787));
#83693=CARTESIAN_POINT('Origin',(2.0635,139.,13.3));
#83694=CARTESIAN_POINT('Ctrl Pts',(2.06350000000018,139.657803339705,14.6073358467788));
#83695=CARTESIAN_POINT('Ctrl Pts',(2.06349989428253,139.684079946574,14.591010615939));
#83696=CARTESIAN_POINT('Ctrl Pts',(2.06350000000023,139.709768001976,14.5738092016242));
#83697=CARTESIAN_POINT('Ctrl Pts',(2.06350000000016,139.73481752449,14.5557291197204));
#83698=CARTESIAN_POINT('Ctrl Pts',(2.06350000000004,139.781451017712,14.5220702994189));
#83699=CARTESIAN_POINT('Ctrl Pts',(2.06350000000018,139.82587360943,14.4853672608473));
#83700=CARTESIAN_POINT('Ctrl Pts',(2.06350000000009,139.867935641536,14.4459285506673));
#83701=CARTESIAN_POINT('Ctrl Pts',(2.06350000000007,139.882253364624,14.4325037943481));
#83702=CARTESIAN_POINT('Ctrl Pts',(2.06349999999999,139.896297210705,14.4187618210828));
#83703=CARTESIAN_POINT('Ctrl Pts',(2.0635,139.910060112663,14.4047141853808));
#83704=CARTESIAN_POINT('Ctrl Pts',(2.0635,139.919224857191,14.3953598360718));
#83705=CARTESIAN_POINT('Ctrl Pts',(2.06350000000004,139.928266229555,14.3858686242349));
#83706=CARTESIAN_POINT('Ctrl Pts',(2.06350000000003,139.937178156248,14.3762480582926));
#83707=CARTESIAN_POINT('Ctrl Pts',(2.0635,139.976265965014,14.3340521499645));
#83708=CARTESIAN_POINT('Ctrl Pts',(2.06350000000006,140.012758651286,14.289488762563));
#83709=CARTESIAN_POINT('Ctrl Pts',(2.06349999999999,140.046512923681,14.2428726644843));
#83710=CARTESIAN_POINT('Ctrl Pts',(2.06349999999994,140.069594989694,14.2109953412078));
#83711=CARTESIAN_POINT('Ctrl Pts',(2.06349999999989,140.091395632075,14.1781574148101));
#83712=CARTESIAN_POINT('Ctrl Pts',(2.06350000000002,140.111855976246,14.1444544521514));
#83713=CARTESIAN_POINT('Ctrl Pts',(2.06350000000009,140.124030465247,14.124400227025));
#83714=CARTESIAN_POINT('Ctrl Pts',(2.06350000000023,140.135730200644,14.1040396688165));
#83715=CARTESIAN_POINT('Ctrl Pts',(2.06350000000009,140.146940838788,14.0833926592231));
#83716=CARTESIAN_POINT('Ctrl Pts',(2.06350000000002,140.152630135659,14.0729144896885));
#83717=CARTESIAN_POINT('Ctrl Pts',(2.0635000000001,140.158194033354,14.062361138362));
#83718=CARTESIAN_POINT('Ctrl Pts',(2.06350000000009,140.163622324462,14.051751955927));
#83719=CARTESIAN_POINT('Ctrl Pts',(2.06350000000008,140.189238203462,14.0016876671563));
#83720=CARTESIAN_POINT('Ctrl Pts',(2.06350000000014,140.21188389594,13.9502997058246));
#83721=CARTESIAN_POINT('Ctrl Pts',(2.06350000000001,140.231416910877,13.8978764178243));
#83722=CARTESIAN_POINT('Ctrl Pts',(2.06349999999989,140.250468168828,13.846746083592));
#83723=CARTESIAN_POINT('Ctrl Pts',(2.06350000000013,140.266558520148,13.7946298218694));
#83724=CARTESIAN_POINT('Ctrl Pts',(2.06350000000017,140.279507455499,13.7417894949803));
#83725=CARTESIAN_POINT('Ctrl Pts',(2.06350000000019,140.287166257202,13.7105364556663));
#83726=CARTESIAN_POINT('Ctrl Pts',(2.06349999999981,140.29372517824,13.6790300876173));
#83727=CARTESIAN_POINT('Ctrl Pts',(2.06349999999983,140.299138330151,13.6473257620931));
#83728=CARTESIAN_POINT('Ctrl Pts',(2.06349999999983,140.302878403847,13.6254204995194));
#83729=CARTESIAN_POINT('Ctrl Pts',(2.06350000000023,140.306071382412,13.6034207594909));
#83730=CARTESIAN_POINT('Ctrl Pts',(2.0635000000002,140.308700255454,13.5813453715114));
#83731=CARTESIAN_POINT('Ctrl Pts',(2.06350000000018,140.309953510264,13.5708214375904));
#83732=CARTESIAN_POINT('Ctrl Pts',(2.06349999999984,140.3110785436,13.5602790505158));
#83733=CARTESIAN_POINT('Ctrl Pts',(2.06349999999987,140.312072069745,13.5497379143829));
#83734=CARTESIAN_POINT('Ctrl Pts',(2.06350000000001,140.317021324794,13.497227196353));
#83735=CARTESIAN_POINT('Ctrl Pts',(2.06350000000023,140.318724308353,13.4446473264495));
#83736=CARTESIAN_POINT('Ctrl Pts',(2.0635000000002,140.31702314186,13.3922422893445));
#83737=CARTESIAN_POINT('Ctrl Pts',(2.0635000000002,140.316671800718,13.3814191008754));
#83738=CARTESIAN_POINT('Ctrl Pts',(2.06350000000014,140.316175081863,13.37060339188));
#83739=CARTESIAN_POINT('Ctrl Pts',(2.06350000000011,140.315531316653,13.3597973595764));
#83740=CARTESIAN_POINT('Ctrl Pts',(2.06349999999993,140.312184859518,13.3036248244557));
#83741=CARTESIAN_POINT('Ctrl Pts',(2.06349999999996,140.304869503365,13.2477115081018));
#83742=CARTESIAN_POINT('Ctrl Pts',(2.0635,140.293769535929,13.1923868892441));
#83743=CARTESIAN_POINT('Ctrl Pts',(2.06350000000001,140.289037860702,13.168803204878));
#83744=CARTESIAN_POINT('Ctrl Pts',(2.06350000000024,140.283617773,13.1453268573598));
#83745=CARTESIAN_POINT('Ctrl Pts',(2.06350000000001,140.277520714535,13.1219853586564));
#83746=CARTESIAN_POINT('Ctrl Pts',(2.06349999999984,140.273131016534,13.1051801843606));
#83747=CARTESIAN_POINT('Ctrl Pts',(2.06350000000026,140.268390372215,13.088444936072));
#83748=CARTESIAN_POINT('Ctrl Pts',(2.06350000000014,140.263302593258,13.0717903762639));
#83749=CARTESIAN_POINT('Ctrl Pts',(2.06350000000007,140.260354166497,13.0621388661973));
#83750=CARTESIAN_POINT('Ctrl Pts',(2.06349999999997,140.257291730647,13.0525230050277));
#83751=CARTESIAN_POINT('Ctrl Pts',(2.06349999999996,140.25411792868,13.0429485488959));
#83752=CARTESIAN_POINT('Ctrl Pts',(2.0634999999999,140.237589408932,12.9930867147718));
#83753=CARTESIAN_POINT('Ctrl Pts',(2.06349999999985,140.21803357519,12.9443107641048));
#83754=CARTESIAN_POINT('Ctrl Pts',(2.06350000000003,140.195622000842,12.8968802651591));
#83755=CARTESIAN_POINT('Ctrl Pts',(2.06350000000021,140.173326992335,12.849696459103));
#83756=CARTESIAN_POINT('Ctrl Pts',(2.06350000000015,140.148205079085,12.8038432496687));
#83757=CARTESIAN_POINT('Ctrl Pts',(2.06350000000018,140.120386075282,12.7596089388244));
#83758=CARTESIAN_POINT('Ctrl Pts',(2.06350000000019,140.106465222191,12.7374737341553));
#83759=CARTESIAN_POINT('Ctrl Pts',(2.06349999999988,140.091868456507,12.7157445125586));
#83760=CARTESIAN_POINT('Ctrl Pts',(2.06349999999998,140.076609269789,12.6944615591124));
#83761=CARTESIAN_POINT('Ctrl Pts',(2.06350000000006,140.06536335881,12.678776175334));
#83762=CARTESIAN_POINT('Ctrl Pts',(2.06349999999983,140.053757610563,12.6633332439248));
#83763=CARTESIAN_POINT('Ctrl Pts',(2.06349999999981,140.041796927407,12.6481500329652));
#83764=CARTESIAN_POINT('Ctrl Pts',(2.0634999999998,140.036011601584,12.6408059856978));
#83765=CARTESIAN_POINT('Ctrl Pts',(2.06349999999992,140.030143780519,12.6335235707603));
#83766=CARTESIAN_POINT('Ctrl Pts',(2.06349999999991,140.024202397352,12.62631448201));
#83767=CARTESIAN_POINT('Ctrl Pts',(2.06349999999989,139.992132527971,12.5874019042322));
#83768=CARTESIAN_POINT('Ctrl Pts',(2.06350000000001,139.957860281516,12.5505432833733));
#83769=CARTESIAN_POINT('Ctrl Pts',(2.06350000000002,139.921515012406,12.5159914507611));
#83770=CARTESIAN_POINT('Ctrl Pts',(2.06350000000004,139.885895513455,12.4821295755946));
#83771=CARTESIAN_POINT('Ctrl Pts',(2.06350000000002,139.84828421327,12.4504826970841));
#83772=CARTESIAN_POINT('Ctrl Pts',(2.06349999999996,139.808779096866,12.4213324380416));
#83773=CARTESIAN_POINT('Ctrl Pts',(2.0634999999999,139.769273980462,12.392182178999));
#83774=CARTESIAN_POINT('Ctrl Pts',(2.06349999999984,139.727874423062,12.3655278554708));
#83775=CARTESIAN_POINT('Ctrl Pts',(2.06349999999994,139.684664424539,12.3417048010816));
#83776=CARTESIAN_POINT('Ctrl Pts',(1.89596885983369,139.853032748447,12.1054162410973));
#83777=CARTESIAN_POINT('Ctrl Pts',(1.92239202009947,140.249693546547,12.3886532696619));
#83778=CARTESIAN_POINT('Ctrl Pts',(1.97523171512371,140.731457227216,13.376929657557));
#83779=CARTESIAN_POINT('Ctrl Pts',(2.05448794490642,139.876218985649,14.7974726129258));
#83780=CARTESIAN_POINT('Ctrl Pts',(2.13373754918179,138.220031131084,14.8484165931406));
#83781=CARTESIAN_POINT('Ctrl Pts',(2.21298715345717,137.276245446404,13.4879812017709));
#83782=CARTESIAN_POINT('Ctrl Pts',(2.29223675773254,137.904992849519,11.9552937639631));
#83783=CARTESIAN_POINT('Ctrl Pts',(2.37148636200791,139.533067892115,11.6499624106074));
#83784=CARTESIAN_POINT('Ctrl Pts',(2.45073596628329,140.674653851833,12.8500720032827));
#83785=CARTESIAN_POINT('Ctrl Pts',(2.52998557055866,140.28820612476,14.4608100243095));
#83786=CARTESIAN_POINT('Ctrl Pts',(2.60923517483404,138.72628924818,15.0123030597136));
#83787=CARTESIAN_POINT('Ctrl Pts',(2.68848477910941,137.414134523873,14.0013890496938));
#83788=CARTESIAN_POINT('Ctrl Pts',(2.76773438338479,137.549031147364,12.3504687424606));
#83789=CARTESIAN_POINT('Ctrl Pts',(2.84698398766016,139.00789645503,11.5659724020108));
#83790=CARTESIAN_POINT('Ctrl Pts',(2.92623359193554,140.459555443865,12.3637232239451));
#83791=CARTESIAN_POINT('Ctrl Pts',(3.0054831962109,140.579413374398,14.0158002212712));
#83792=CARTESIAN_POINT('Ctrl Pts',(3.08473280048628,139.258102654343,15.0147299843183));
#83793=CARTESIAN_POINT('Ctrl Pts',(3.16398240476165,137.701280945341,14.4490191483896));
#83794=CARTESIAN_POINT('Ctrl Pts',(3.24323200903703,137.329502248306,12.8348618994128));
#83795=CARTESIAN_POINT('Ctrl Pts',(3.3224816133124,138.482003811076,11.6451295913287));
#83796=CARTESIAN_POINT('Ctrl Pts',(3.40173121758777,140.107161699214,11.9654179947715));
#83797=CARTESIAN_POINT('Ctrl Pts',(3.48098082186315,140.722066996773,13.5034733719682));
#83798=CARTESIAN_POINT('Ctrl Pts',(3.56023042613852,139.765636634447,14.8558652548918));
#83799=CARTESIAN_POINT('Ctrl Pts',(3.6394800304139,138.110585287296,14.7885757019759));
#83800=CARTESIAN_POINT('Ctrl Pts',(3.71872963468927,137.267098793937,13.363004453076));
#83801=CARTESIAN_POINT('Ctrl Pts',(3.79797923896465,138.00483385609,11.8799434883052));
#83802=CARTESIAN_POINT('Ctrl Pts',(3.87722884324002,139.650628853749,11.6926424649233));
#83803=CARTESIAN_POINT('Ctrl Pts',(3.95647844751539,140.702744093894,12.9720080770802));
#83804=CARTESIAN_POINT('Ctrl Pts',(4.03572805179077,140.201155259721,14.5506567046047));
#83805=CARTESIAN_POINT('Ctrl Pts',(4.11497765606614,138.603547459727,14.9881177488894));
#83806=CARTESIAN_POINT('Ctrl Pts',(4.19422726034152,137.36769098179,13.8852208299455));
#83807=CARTESIAN_POINT('Ctrl Pts',(4.27347686461689,137.621268636156,12.2483270579015));
#83808=CARTESIAN_POINT('Ctrl Pts',(4.35272646889227,139.13289824627,11.5710540184731));
#83809=CARTESIAN_POINT('Ctrl Pts',(4.43197607316764,140.523262102069,12.4713935078738));
#83810=CARTESIAN_POINT('Ctrl Pts',(4.51122567744301,140.523693940408,14.1278121327004));
#83811=CARTESIAN_POINT('Ctrl Pts',(4.59047528171839,139.133799720494,15.0288764520582));
#83812=CARTESIAN_POINT('Ctrl Pts',(4.66972488599376,137.621817178961,14.3523916852465));
#83813=CARTESIAN_POINT('Ctrl Pts',(4.74897449026913,137.367386061086,12.715630355902));
#83814=CARTESIAN_POINT('Ctrl Pts',(4.82822409454451,138.602667312506,11.612089193016));
#83815=CARTESIAN_POINT('Ctrl Pts',(4.90747369881989,140.200502982632,12.0487171742856));
#83816=CARTESIAN_POINT('Ctrl Pts',(4.98672330309525,140.702914895189,13.6271040366256));
#83817=CARTESIAN_POINT('Ctrl Pts',(5.06597290737063,139.651466831615,14.9070180937402));
#83818=CARTESIAN_POINT('Ctrl Pts',(5.14522251164601,138.005574484851,14.7205751631362));
#83819=CARTESIAN_POINT('Ctrl Pts',(5.22447211592137,137.267066055636,13.2378992071656));
#83820=CARTESIAN_POINT('Ctrl Pts',(5.30372172019676,138.109809500551,11.8118880519989));
#83821=CARTESIAN_POINT('Ctrl Pts',(5.38297132447213,139.764824761192,11.7437361569266));
#83822=CARTESIAN_POINT('Ctrl Pts',(5.4622209287475,140.721961748847,13.0956278985068));
#83823=CARTESIAN_POINT('Ctrl Pts',(5.54147053302288,140.107855186128,14.6340062945752));
#83824=CARTESIAN_POINT('Ctrl Pts',(5.62072013729825,138.482871353761,14.9551366430618));
#83825=CARTESIAN_POINT('Ctrl Pts',(5.69996974157362,137.329735497801,13.7660165502442));
#83826=CARTESIAN_POINT('Ctrl Pts',(5.779219345849,137.700701639676,12.1516426964784));
#83827=CARTESIAN_POINT('Ctrl Pts',(5.85846895012437,139.257168003577,11.585167634447));
#83828=CARTESIAN_POINT('Ctrl Pts',(5.93771855439974,140.579123638415,12.5833103492865));
#83829=CARTESIAN_POINT('Ctrl Pts',(6.01696815867512,140.45987057973,14.2356519565008));
#83830=CARTESIAN_POINT('Ctrl Pts',(6.09621776295049,139.009157629426,15.0337420570016));
#83831=CARTESIAN_POINT('Ctrl Pts',(6.17546736722587,137.54878859506,14.2508782232481));
#83832=CARTESIAN_POINT('Ctrl Pts',(6.25472476122387,137.415305990955,12.5981114806508));
#83833=CARTESIAN_POINT('Ctrl Pts',(6.30756562046341,138.286672883565,11.9276015280158));
#83834=CARTESIAN_POINT('Ctrl Pts',(6.33398994494448,138.767973032967,11.8505660727666));
#83835=CARTESIAN_POINT('Ctrl Pts',(1.95222224061816,139.796411161913,12.1847088917025));
#83836=CARTESIAN_POINT('Ctrl Pts',(1.97864540088395,140.166742884434,12.4491455518734));
#83837=CARTESIAN_POINT('Ctrl Pts',(2.03148509590819,140.61652863227,13.371823312847));
#83838=CARTESIAN_POINT('Ctrl Pts',(2.1107413256909,139.818058370819,14.6980751685837));
#83839=CARTESIAN_POINT('Ctrl Pts',(2.18999092996627,138.271802970893,14.7456376502693));
#83840=CARTESIAN_POINT('Ctrl Pts',(2.26924053424165,137.390662762501,13.4755036106089));
#83841=CARTESIAN_POINT('Ctrl Pts',(2.34849013851702,137.977675923223,12.0445510646305));
#83842=CARTESIAN_POINT('Ctrl Pts',(2.42773974279239,139.497684549755,11.7594866303082));
#83843=CARTESIAN_POINT('Ctrl Pts',(2.50698934706777,140.563495683334,12.8799367851997));
#83844=CARTESIAN_POINT('Ctrl Pts',(2.58623895134316,140.202699120838,14.3837591662256));
#83845=CARTESIAN_POINT('Ctrl Pts',(2.66548855561852,138.744457292782,14.8986458571674));
#83846=CARTESIAN_POINT('Ctrl Pts',(2.74473815989389,137.519399203867,13.954833087049));
#83847=CARTESIAN_POINT('Ctrl Pts',(2.82398776416927,137.645341820781,12.4134955915047));
#83848=CARTESIAN_POINT('Ctrl Pts',(2.90323736844464,139.007372313592,11.6810716099503));
#83849=CARTESIAN_POINT('Ctrl Pts',(2.98248697272001,140.362674819976,12.4258702828854));
#83850=CARTESIAN_POINT('Ctrl Pts',(3.06173657699539,140.47457696429,13.9682876911322));
#83851=CARTESIAN_POINT('Ctrl Pts',(3.14098618127076,139.24097062535,14.9009116902761));
#83852=CARTESIAN_POINT('Ctrl Pts',(3.22023578554614,137.787485763937,14.3727509309516));
#83853=CARTESIAN_POINT('Ctrl Pts',(3.29948538982151,137.440384548166,12.8657362793951));
#83854=CARTESIAN_POINT('Ctrl Pts',(3.37873499409688,138.516386741965,11.754974598122));
#83855=CARTESIAN_POINT('Ctrl Pts',(3.45798459837226,140.033671845426,12.054003281367));
#83856=CARTESIAN_POINT('Ctrl Pts',(3.53723420264763,140.607761695303,13.48996746008));
#83857=CARTESIAN_POINT('Ctrl Pts',(3.616483806923,139.714816122536,14.7525918936683));
#83858=CARTESIAN_POINT('Ctrl Pts',(3.69573341119839,138.169621792299,14.6897688061374));
#83859=CARTESIAN_POINT('Ctrl Pts',(3.77498301547375,137.382123235581,13.3588224189182));
#83860=CARTESIAN_POINT('Ctrl Pts',(3.85423261974913,138.070889802988,11.9742022993617));
#83861=CARTESIAN_POINT('Ctrl Pts',(3.9334822240245,139.607442190621,11.799333719075));
#83862=CARTESIAN_POINT('Ctrl Pts',(4.01273182829988,140.589721384936,12.9937791322712));
#83863=CARTESIAN_POINT('Ctrl Pts',(4.09198143257525,140.121426413903,14.4676421111397));
#83864=CARTESIAN_POINT('Ctrl Pts',(4.17123103685062,138.629862711817,14.8760658899505));
#83865=CARTESIAN_POINT('Ctrl Pts',(4.250480641126,137.476038435618,13.8463757423157));
#83866=CARTESIAN_POINT('Ctrl Pts',(4.32973024540137,137.712784416022,12.3181337454002));
#83867=CARTESIAN_POINT('Ctrl Pts',(4.40897984967675,139.124076885584,11.6858159249589));
#83868=CARTESIAN_POINT('Ctrl Pts',(4.48822945395212,140.422152833892,12.5263937576091));
#83869=CARTESIAN_POINT('Ctrl Pts',(4.5674790582275,140.422556008183,14.0728646100041));
#83870=CARTESIAN_POINT('Ctrl Pts',(4.64672866250288,139.124918522831,14.9141191607164));
#83871=CARTESIAN_POINT('Ctrl Pts',(4.72597826677826,137.713296548309,14.2825372898755));
#83872=CARTESIAN_POINT('Ctrl Pts',(4.80522787105361,137.475753754575,12.7544189445367));
#83873=CARTESIAN_POINT('Ctrl Pts',(4.88447747532899,138.629040985953,11.7241273158127));
#83874=CARTESIAN_POINT('Ctrl Pts',(4.96372707960436,140.120817432881,12.1317733276681));
#83875=CARTESIAN_POINT('Ctrl Pts',(5.04297668387974,140.589880848987,13.6053919164879));
#83876=CARTESIAN_POINT('Ctrl Pts',(5.12222628815512,139.608224546196,14.8003493706192));
#83877=CARTESIAN_POINT('Ctrl Pts',(5.2014758924305,138.07158127118,14.6262819256554));
#83878=CARTESIAN_POINT('Ctrl Pts',(5.28072549670586,137.382092670345,13.2420212592459));
#83879=CARTESIAN_POINT('Ctrl Pts',(5.35997510098123,138.168897499796,11.9106641653312));
#83880=CARTESIAN_POINT('Ctrl Pts',(5.43922470525661,139.714058138834,11.8470359751594));
#83881=CARTESIAN_POINT('Ctrl Pts',(5.51847430953198,140.607663433396,13.1091934651874));
#83882=CARTESIAN_POINT('Ctrl Pts',(5.59772391380736,140.034319300897,14.5454592218123));
#83883=CARTESIAN_POINT('Ctrl Pts',(5.67697351808273,138.51719669994,14.845273964481));
#83884=CARTESIAN_POINT('Ctrl Pts',(5.75622312235812,137.440602315305,13.7350838615822));
#83885=CARTESIAN_POINT('Ctrl Pts',(5.83547272663349,137.786944910733,12.2278669827701));
#83886=CARTESIAN_POINT('Ctrl Pts',(5.91472233090886,139.240098013714,11.6989927242281));
#83887=CARTESIAN_POINT('Ctrl Pts',(5.99397193518423,140.474306460055,12.6308819169081));
#83888=CARTESIAN_POINT('Ctrl Pts',(6.0732215394596,140.36296903813,14.173546371085));
#83889=CARTESIAN_POINT('Ctrl Pts',(6.15247114373499,139.008549775264,14.91866180236));
#83890=CARTESIAN_POINT('Ctrl Pts',(6.23172074801035,137.645115368322,14.187761966927));
#83891=CARTESIAN_POINT('Ctrl Pts',(6.31097814200836,137.520492912708,12.6447005964944));
#83892=CARTESIAN_POINT('Ctrl Pts',(6.36381900124789,138.334021256911,12.018696950768));
#83893=CARTESIAN_POINT('Ctrl Pts',(6.39024332572898,138.783374241205,11.9467748627412));
#83894=CARTESIAN_POINT('Ctrl Pts',(2.00847562140265,139.739789575378,12.2640015423077));
#83895=CARTESIAN_POINT('Ctrl Pts',(2.03489878166844,140.083792222322,12.509637834085));
#83896=CARTESIAN_POINT('Ctrl Pts',(2.08773847669269,140.501600037324,13.3667169681371));
#83897=CARTESIAN_POINT('Ctrl Pts',(2.16699470647539,139.759897755991,14.5986777242415));
#83898=CARTESIAN_POINT('Ctrl Pts',(2.24624431075077,138.323574810704,14.6428587073981));
#83899=CARTESIAN_POINT('Ctrl Pts',(2.32549391502614,137.505080078599,13.4630260194469));
#83900=CARTESIAN_POINT('Ctrl Pts',(2.40474351930151,138.050358996926,12.1338083652978));
#83901=CARTESIAN_POINT('Ctrl Pts',(2.48399312357689,139.462301207396,11.8690108500091));
#83902=CARTESIAN_POINT('Ctrl Pts',(2.56324272785226,140.452337514835,12.9098015671167));
#83903=CARTESIAN_POINT('Ctrl Pts',(2.64249233212764,140.117192116915,14.3067083081417));
#83904=CARTESIAN_POINT('Ctrl Pts',(2.72174193640301,138.762625337382,14.7849886546212));
#83905=CARTESIAN_POINT('Ctrl Pts',(2.80099154067839,137.624663883859,13.908277124404));
#83906=CARTESIAN_POINT('Ctrl Pts',(2.88024114495376,137.741652494196,12.4765224405487));
#83907=CARTESIAN_POINT('Ctrl Pts',(2.95949074922913,139.006848172153,11.7961708178899));
#83908=CARTESIAN_POINT('Ctrl Pts',(3.03874035350451,140.265794196088,12.4880173418254));
#83909=CARTESIAN_POINT('Ctrl Pts',(3.11798995777988,140.369740554181,13.9207751609933));
#83910=CARTESIAN_POINT('Ctrl Pts',(3.19723956205525,139.223838596359,14.7870933962339));
#83911=CARTESIAN_POINT('Ctrl Pts',(3.27648916633063,137.873690582534,14.2964827135134));
#83912=CARTESIAN_POINT('Ctrl Pts',(3.355738770606,137.551266848025,12.8966106593774));
#83913=CARTESIAN_POINT('Ctrl Pts',(3.43498837488138,138.550769672853,11.864819604915));
#83914=CARTESIAN_POINT('Ctrl Pts',(3.51423797915675,139.960181991637,12.1425885679623));
#83915=CARTESIAN_POINT('Ctrl Pts',(3.59348758343212,140.493456393832,13.4764615481916));
#83916=CARTESIAN_POINT('Ctrl Pts',(3.6727371877075,139.663995610628,14.6493185324447));
#83917=CARTESIAN_POINT('Ctrl Pts',(3.75198679198287,138.2286582973,14.590961910299));
#83918=CARTESIAN_POINT('Ctrl Pts',(3.83123639625824,137.497147677226,13.35464038476));
#83919=CARTESIAN_POINT('Ctrl Pts',(3.91048600053362,138.136945749885,12.0684611104179));
#83920=CARTESIAN_POINT('Ctrl Pts',(3.98973560480899,139.564255527493,11.9060249732265));
#83921=CARTESIAN_POINT('Ctrl Pts',(4.06898520908437,140.476698675979,13.0155501874623));
#83922=CARTESIAN_POINT('Ctrl Pts',(4.14823481335974,140.041697568084,14.3846275176746));
#83923=CARTESIAN_POINT('Ctrl Pts',(4.22748441763512,138.656177963905,14.7640140310118));
#83924=CARTESIAN_POINT('Ctrl Pts',(4.30673402191049,137.584385889446,13.8075306546858));
#83925=CARTESIAN_POINT('Ctrl Pts',(4.38598362618586,137.804300195889,12.3879404328989));
#83926=CARTESIAN_POINT('Ctrl Pts',(4.46523323046124,139.115255524898,11.8005778314444));
#83927=CARTESIAN_POINT('Ctrl Pts',(4.54448283473661,140.321043565714,12.5813940073443));
#83928=CARTESIAN_POINT('Ctrl Pts',(4.62373243901199,140.321418075957,14.0179170873078));
#83929=CARTESIAN_POINT('Ctrl Pts',(4.70298204328736,139.116037325168,14.7993618693745));
#83930=CARTESIAN_POINT('Ctrl Pts',(4.78223164756273,137.804775917658,14.2126828945046));
#83931=CARTESIAN_POINT('Ctrl Pts',(4.86148125183811,137.584121448064,12.7932075331713));
#83932=CARTESIAN_POINT('Ctrl Pts',(4.94073085611348,138.655414659402,11.8361654386095));
#83933=CARTESIAN_POINT('Ctrl Pts',(5.01998046038886,140.041131883128,12.2148294810507));
#83934=CARTESIAN_POINT('Ctrl Pts',(5.09923006466423,140.476846802786,13.5836797963504));
#83935=CARTESIAN_POINT('Ctrl Pts',(5.17847966893961,139.564982260777,14.6936806474984));
#83936=CARTESIAN_POINT('Ctrl Pts',(5.25772927321498,138.137588057508,14.5319886881745));
#83937=CARTESIAN_POINT('Ctrl Pts',(5.33697887749035,137.497119285054,13.2461433113263));
#83938=CARTESIAN_POINT('Ctrl Pts',(5.41622848176573,138.227985499041,12.0094402786633));
#83939=CARTESIAN_POINT('Ctrl Pts',(5.4954780860411,139.663291516476,11.950335793392));
#83940=CARTESIAN_POINT('Ctrl Pts',(5.57472769031648,140.493365117947,13.1227590318682));
#83941=CARTESIAN_POINT('Ctrl Pts',(5.65397729459185,139.960783415665,14.4569121490495));
#83942=CARTESIAN_POINT('Ctrl Pts',(5.73322689886722,138.551522046119,14.7354112859003));
#83943=CARTESIAN_POINT('Ctrl Pts',(5.8124765031426,137.551469132808,13.7041511729202));
#83944=CARTESIAN_POINT('Ctrl Pts',(5.89172610741797,137.873188181787,12.3040912690618));
#83945=CARTESIAN_POINT('Ctrl Pts',(5.97097571169335,139.223028023853,11.8128178140093));
#83946=CARTESIAN_POINT('Ctrl Pts',(6.05022531596872,140.369489281695,12.6784534845299));
#83947=CARTESIAN_POINT('Ctrl Pts',(6.1294749202441,140.266067496531,14.1114407856692));
#83948=CARTESIAN_POINT('Ctrl Pts',(6.20872452451946,139.0079419211,14.8035815477182));
#83949=CARTESIAN_POINT('Ctrl Pts',(6.28797412879484,137.741442141584,14.1246457106057));
#83950=CARTESIAN_POINT('Ctrl Pts',(6.36723152279283,137.625679834461,12.6912897123383));
#83951=CARTESIAN_POINT('Ctrl Pts',(6.42007238203238,138.381369630258,12.1097923735202));
#83952=CARTESIAN_POINT('Ctrl Pts',(6.44649670651346,138.798775449443,12.0429836527158));
#83953=CARTESIAN_POINT('Ctrl Pts',(2.06472900218714,139.683167988843,12.3432941929129));
#83954=CARTESIAN_POINT('Ctrl Pts',(2.09115216245292,140.000841560209,12.5701301162965));
#83955=CARTESIAN_POINT('Ctrl Pts',(2.14399185747717,140.386671442379,13.3616106234272));
#83956=CARTESIAN_POINT('Ctrl Pts',(2.22324808725986,139.701737141161,14.4992802798993));
#83957=CARTESIAN_POINT('Ctrl Pts',(2.30249769153524,138.375346650514,14.5400797645268));
#83958=CARTESIAN_POINT('Ctrl Pts',(2.38174729581061,137.619497394696,13.4505484282849));
#83959=CARTESIAN_POINT('Ctrl Pts',(2.46099690008598,138.123042070629,12.2230656659651));
#83960=CARTESIAN_POINT('Ctrl Pts',(2.54024650436136,139.426917865036,11.97853506971));
#83961=CARTESIAN_POINT('Ctrl Pts',(2.61949610863673,140.341179346336,12.9396663490336));
#83962=CARTESIAN_POINT('Ctrl Pts',(2.69874571291211,140.031685112994,14.2296574500578));
#83963=CARTESIAN_POINT('Ctrl Pts',(2.77799531718748,138.780793381982,14.6713314520748));
#83964=CARTESIAN_POINT('Ctrl Pts',(2.85724492146286,137.729928563852,13.8617211617591));
#83965=CARTESIAN_POINT('Ctrl Pts',(2.93649452573823,137.837963167611,12.5395492895927));
#83966=CARTESIAN_POINT('Ctrl Pts',(3.0157441300136,139.006324030715,11.9112700258293));
#83967=CARTESIAN_POINT('Ctrl Pts',(3.09499373428898,140.1689135722,12.5501644007656));
#83968=CARTESIAN_POINT('Ctrl Pts',(3.17424333856435,140.264904144072,13.8732626308543));
#83969=CARTESIAN_POINT('Ctrl Pts',(3.25349294283972,139.206706567366,14.6732751021918));
#83970=CARTESIAN_POINT('Ctrl Pts',(3.3327425471151,137.959895401132,14.2202144960755));
#83971=CARTESIAN_POINT('Ctrl Pts',(3.41199215139047,137.662149147884,12.9274850393596));
#83972=CARTESIAN_POINT('Ctrl Pts',(3.49124175566585,138.585152603743,11.9746646117082));
#83973=CARTESIAN_POINT('Ctrl Pts',(3.57049135994122,139.88669213785,12.2311738545576));
#83974=CARTESIAN_POINT('Ctrl Pts',(3.6497409642166,140.37915109236,13.4629556363033));
#83975=CARTESIAN_POINT('Ctrl Pts',(3.72899056849197,139.613175098719,14.5460451712212));
#83976=CARTESIAN_POINT('Ctrl Pts',(3.80824017276735,138.287694802302,14.4921550144606));
#83977=CARTESIAN_POINT('Ctrl Pts',(3.88748977704271,137.612172118871,13.350458350602));
#83978=CARTESIAN_POINT('Ctrl Pts',(3.9667393813181,138.203001696784,12.1627199214744));
#83979=CARTESIAN_POINT('Ctrl Pts',(4.04598898559346,139.521068864365,12.0127162273781));
#83980=CARTESIAN_POINT('Ctrl Pts',(4.12523858986884,140.363675967023,13.0373212426534));
#83981=CARTESIAN_POINT('Ctrl Pts',(4.20448819414421,139.961968722265,14.3016129242096));
#83982=CARTESIAN_POINT('Ctrl Pts',(4.28373779841958,138.682493215994,14.651962172073));
#83983=CARTESIAN_POINT('Ctrl Pts',(4.36298740269496,137.692733343272,13.768685567056));
#83984=CARTESIAN_POINT('Ctrl Pts',(4.44223700697033,137.895815975755,12.4577471203976));
#83985=CARTESIAN_POINT('Ctrl Pts',(4.52148661124571,139.106434164211,11.9153397379301));
#83986=CARTESIAN_POINT('Ctrl Pts',(4.60073621552108,140.219934297536,12.6363942570796));
#83987=CARTESIAN_POINT('Ctrl Pts',(4.67998581979646,140.220280143731,13.9629695646115));
#83988=CARTESIAN_POINT('Ctrl Pts',(4.75923542407183,139.107156127504,14.6846045780327));
#83989=CARTESIAN_POINT('Ctrl Pts',(4.8384850283472,137.896255287007,14.1428284991337));
#83990=CARTESIAN_POINT('Ctrl Pts',(4.91773463262258,137.692489141553,12.831996121806));
#83991=CARTESIAN_POINT('Ctrl Pts',(4.99698423689795,138.681788332849,11.9482035614062));
#83992=CARTESIAN_POINT('Ctrl Pts',(5.07623384117334,139.961446333378,12.2978856344331));
#83993=CARTESIAN_POINT('Ctrl Pts',(5.1554834454487,140.363812756586,13.5619676762128));
#83994=CARTESIAN_POINT('Ctrl Pts',(5.23473304972408,139.521739975356,14.5870119243775));
#83995=CARTESIAN_POINT('Ctrl Pts',(5.31398265399944,138.203594843837,14.4376954506937));
#83996=CARTESIAN_POINT('Ctrl Pts',(5.39323225827483,137.612145899761,13.2502653634066));
#83997=CARTESIAN_POINT('Ctrl Pts',(5.4724818625502,138.287073498288,12.1082163919956));
#83998=CARTESIAN_POINT('Ctrl Pts',(5.55173146682557,139.612524894117,12.0536356116246));
#83999=CARTESIAN_POINT('Ctrl Pts',(5.63098107110095,140.379066802497,13.136324598549));
#84000=CARTESIAN_POINT('Ctrl Pts',(5.71023067537633,139.887247530433,14.3683650762867));
#84001=CARTESIAN_POINT('Ctrl Pts',(5.78948027965169,138.585847392298,14.6255486073194));
#84002=CARTESIAN_POINT('Ctrl Pts',(5.86872988392707,137.662335950312,13.6732184842583));
#84003=CARTESIAN_POINT('Ctrl Pts',(5.94797948820244,137.959431452842,12.3803155553536));
#84004=CARTESIAN_POINT('Ctrl Pts',(6.02722909247781,139.205958033989,11.9266429037905));
#84005=CARTESIAN_POINT('Ctrl Pts',(6.10647869675319,140.264672103334,12.7260250521515));
#84006=CARTESIAN_POINT('Ctrl Pts',(6.18572830102857,140.169165954932,14.0493352002535));
#84007=CARTESIAN_POINT('Ctrl Pts',(6.26497790530394,139.007334066938,14.6885012930766));
#84008=CARTESIAN_POINT('Ctrl Pts',(6.34422750957932,137.837768914846,14.0615294542845));
#84009=CARTESIAN_POINT('Ctrl Pts',(6.42348490357732,137.730866756214,12.7378788281818));
#84010=CARTESIAN_POINT('Ctrl Pts',(6.47632576281685,138.428718003605,12.2008877962723));
#84011=CARTESIAN_POINT('Ctrl Pts',(6.50275008729793,138.814176657679,12.1391924426906));
#84012=CARTESIAN_POINT('Ctrl Pts',(2.06350000000012,139.657803339705,14.6073358467789));
#84013=CARTESIAN_POINT('Ctrl Pts',(2.06364329234591,139.653977763695,14.6094211449295));
#84014=CARTESIAN_POINT('Ctrl Pts',(2.06378605389376,139.650142629059,14.6114889008338));
#84015=CARTESIAN_POINT('Ctrl Pts',(2.06407023080022,139.642462904297,14.6155842536617));
#84016=CARTESIAN_POINT('Ctrl Pts',(2.06421164723845,139.638618396783,14.6176119166426));
#84017=CARTESIAN_POINT('Ctrl Pts',(2.06435259587952,139.634764697661,14.6196220306061));
#84018=CARTESIAN_POINT('Origin',(6.5,139.,13.3));
#84019=CARTESIAN_POINT('',(6.4,138.189703570316,13.3965254145956));
#84020=CARTESIAN_POINT('',(6.45000000000003,138.133974596216,13.3));
#84021=CARTESIAN_POINT('Ctrl Pts',(6.4,138.189703570316,13.3965254145956));
#84022=CARTESIAN_POINT('Ctrl Pts',(6.42130722384788,138.162667372368,13.3496973461057));
#84023=CARTESIAN_POINT('Ctrl Pts',(6.45000000000003,138.133974596216,13.3));
#84024=CARTESIAN_POINT('',(6.4,138.511258324007,13.9534745854044));
#84025=CARTESIAN_POINT('Origin',(6.4,139.,13.3));
#84026=CARTESIAN_POINT('',(6.45000000000001,138.566987298108,14.05));
#84027=CARTESIAN_POINT('Ctrl Pts',(6.45000000000001,138.566987298108,14.05));
#84028=CARTESIAN_POINT('Ctrl Pts',(6.42130722384786,138.538294521956,14.0003026538943));
#84029=CARTESIAN_POINT('Ctrl Pts',(6.4,138.511258324007,13.9534745854044));
#84030=CARTESIAN_POINT('',(6.4,138.678445246309,14.05));
#84031=CARTESIAN_POINT('Ctrl Pts',(6.4,138.678445246309,14.05));
#84032=CARTESIAN_POINT('Ctrl Pts',(6.42130722384789,138.624372850412,14.05));
#84033=CARTESIAN_POINT('Ctrl Pts',(6.45000000000001,138.566987298108,14.05));
#84034=CARTESIAN_POINT('',(6.4,139.321554753691,14.05));
#84035=CARTESIAN_POINT('Origin',(6.4,139.,13.3));
#84036=CARTESIAN_POINT('',(6.45,139.433012701892,14.05));
#84037=CARTESIAN_POINT('Ctrl Pts',(6.45,139.433012701892,14.05));
#84038=CARTESIAN_POINT('Ctrl Pts',(6.42130722384791,139.375627149588,14.05));
#84039=CARTESIAN_POINT('Ctrl Pts',(6.4,139.321554753691,14.05));
#84040=CARTESIAN_POINT('',(6.4,139.488741675993,13.9534745854044));
#84041=CARTESIAN_POINT('Ctrl Pts',(6.4,139.488741675993,13.9534745854044));
#84042=CARTESIAN_POINT('Ctrl Pts',(6.4213072238479,139.461705478044,14.0003026538944));
#84043=CARTESIAN_POINT('Ctrl Pts',(6.45,139.433012701892,14.05));
#84044=CARTESIAN_POINT('',(6.4,139.810296429684,13.3965254145956));
#84045=CARTESIAN_POINT('Origin',(6.4,139.,13.3));
#84046=CARTESIAN_POINT('',(6.45000000000003,139.866025403784,13.3));
#84047=CARTESIAN_POINT('Ctrl Pts',(6.45000000000003,139.866025403784,13.3));
#84048=CARTESIAN_POINT('Ctrl Pts',(6.42130722384793,139.837332627632,13.3496973461056));
#84049=CARTESIAN_POINT('Ctrl Pts',(6.4,139.810296429684,13.3965254145956));
#84050=CARTESIAN_POINT('',(6.4,139.810296429684,13.2034745854044));
#84051=CARTESIAN_POINT('Ctrl Pts',(6.4,139.810296429684,13.2034745854044));
#84052=CARTESIAN_POINT('Ctrl Pts',(6.42130722384792,139.837332627632,13.2503026538944));
#84053=CARTESIAN_POINT('Ctrl Pts',(6.45000000000003,139.866025403784,13.3));
#84054=CARTESIAN_POINT('',(6.4,139.488741675993,12.6465254145956));
#84055=CARTESIAN_POINT('Origin',(6.4,139.,13.3));
#84056=CARTESIAN_POINT('',(6.45,139.433012701892,12.55));
#84057=CARTESIAN_POINT('Ctrl Pts',(6.45,139.433012701892,12.55));
#84058=CARTESIAN_POINT('Ctrl Pts',(6.42130722384787,139.461705478044,12.5996973461056));
#84059=CARTESIAN_POINT('Ctrl Pts',(6.4,139.488741675993,12.6465254145956));
#84060=CARTESIAN_POINT('',(6.4,139.321554753691,12.55));
#84061=CARTESIAN_POINT('Ctrl Pts',(6.4,139.321554753691,12.55));
#84062=CARTESIAN_POINT('Ctrl Pts',(6.4213072238479,139.375627149588,12.55));
#84063=CARTESIAN_POINT('Ctrl Pts',(6.45,139.433012701892,12.55));
#84064=CARTESIAN_POINT('',(6.4,138.678445246309,12.55));
#84065=CARTESIAN_POINT('Origin',(6.4,139.,13.3));
#84066=CARTESIAN_POINT('',(6.45000000000001,138.566987298108,12.55));
#84067=CARTESIAN_POINT('Ctrl Pts',(6.45000000000001,138.566987298108,12.55));
#84068=CARTESIAN_POINT('Ctrl Pts',(6.4213072238479,138.624372850412,12.55));
#84069=CARTESIAN_POINT('Ctrl Pts',(6.4,138.678445246309,12.55));
#84070=CARTESIAN_POINT('',(6.4,138.511258324007,12.6465254145956));
#84071=CARTESIAN_POINT('Ctrl Pts',(6.39999999999999,138.511258324007,12.6465254145956));
#84072=CARTESIAN_POINT('Ctrl Pts',(6.42130722384788,138.538294521956,12.5996973461056));
#84073=CARTESIAN_POINT('Ctrl Pts',(6.45000000000001,138.566987298108,12.55));
#84074=CARTESIAN_POINT('',(6.4,138.189703570316,13.2034745854044));
#84075=CARTESIAN_POINT('Origin',(6.4,139.,13.3));
#84076=CARTESIAN_POINT('Ctrl Pts',(6.45000000000003,138.133974596216,13.3));
#84077=CARTESIAN_POINT('Ctrl Pts',(6.42130722384786,138.162667372368,13.2503026538943));
#84078=CARTESIAN_POINT('Ctrl Pts',(6.4,138.189703570316,13.2034745854043));
#84079=CARTESIAN_POINT('',(6.6,137.983974596216,13.3));
#84080=CARTESIAN_POINT('',(6.5,138.083974596216,13.3));
#84081=CARTESIAN_POINT('Origin',(6.6,139.,13.3));
#84082=CARTESIAN_POINT('Origin',(6.5,139.,13.3));
#84083=CARTESIAN_POINT('',(6.6,138.678445246309,12.55));
#84084=CARTESIAN_POINT('',(6.5,138.678445246309,12.55));
#84085=CARTESIAN_POINT('',(6.6,139.321554753691,12.55));
#84086=CARTESIAN_POINT('',(6.5,139.321554753691,12.55));
#84087=CARTESIAN_POINT('Origin',(6.6,139.,13.3));
#84088=CARTESIAN_POINT('Origin',(6.5,139.,13.3));
#84089=CARTESIAN_POINT('',(6.6,139.810296429684,13.2034745854044));
#84090=CARTESIAN_POINT('',(6.5,139.810296429684,13.2034745854044));
#84091=CARTESIAN_POINT('',(6.6,139.488741675993,12.6465254145956));
#84092=CARTESIAN_POINT('Origin',(6.6,139.,13.3));
#84093=CARTESIAN_POINT('',(6.5,139.488741675993,12.6465254145956));
#84094=CARTESIAN_POINT('Origin',(6.5,139.,13.3));
#84095=CARTESIAN_POINT('',(6.6,138.189703570316,13.2034745854044));
#84096=CARTESIAN_POINT('',(6.5,138.189703570316,13.2034745854044));
#84097=CARTESIAN_POINT('',(6.6,138.511258324007,12.6465254145956));
#84098=CARTESIAN_POINT('',(6.5,138.511258324007,12.6465254145956));
#84099=CARTESIAN_POINT('Origin',(6.6,139.,13.3));
#84100=CARTESIAN_POINT('Origin',(6.5,139.,13.3));
#84101=CARTESIAN_POINT('',(6.6,139.488741675993,13.9534745854044));
#84102=CARTESIAN_POINT('',(6.5,139.488741675993,13.9534745854044));
#84103=CARTESIAN_POINT('',(6.6,139.810296429684,13.3965254145956));
#84104=CARTESIAN_POINT('Origin',(6.6,139.,13.3));
#84105=CARTESIAN_POINT('',(6.5,139.810296429684,13.3965254145956));
#84106=CARTESIAN_POINT('Origin',(6.5,139.,13.3));
#84107=CARTESIAN_POINT('',(6.6,138.511258324007,13.9534745854044));
#84108=CARTESIAN_POINT('',(6.5,138.511258324007,13.9534745854044));
#84109=CARTESIAN_POINT('',(6.6,138.189703570316,13.3965254145956));
#84110=CARTESIAN_POINT('',(6.5,138.189703570316,13.3965254145956));
#84111=CARTESIAN_POINT('Origin',(6.6,139.,13.3));
#84112=CARTESIAN_POINT('Origin',(6.5,139.,13.3));
#84113=CARTESIAN_POINT('',(6.6,138.678445246309,14.05));
#84114=CARTESIAN_POINT('',(6.5,138.678445246309,14.05));
#84115=CARTESIAN_POINT('',(6.6,139.321554753691,14.05));
#84116=CARTESIAN_POINT('Origin',(6.6,139.,13.3));
#84117=CARTESIAN_POINT('',(6.5,139.321554753691,14.05));
#84118=CARTESIAN_POINT('Origin',(6.6,138.133974596216,13.3));
#84119=CARTESIAN_POINT('',(6.6,138.242227771689,13.4875));
#84120=CARTESIAN_POINT('',(5.1,138.133974596216,13.3));
#84121=CARTESIAN_POINT('',(6.6,138.133974596216,13.3));
#84122=CARTESIAN_POINT('',(5.1,138.566987298108,14.05));
#84123=CARTESIAN_POINT('',(5.1,138.566987298108,14.05));
#84124=CARTESIAN_POINT('',(6.6,138.566987298108,14.05));
#84125=CARTESIAN_POINT('Origin',(6.6,138.566987298108,12.55));
#84126=CARTESIAN_POINT('',(6.6,138.458734122635,12.7375));
#84127=CARTESIAN_POINT('',(5.1,138.566987298108,12.55));
#84128=CARTESIAN_POINT('',(6.6,138.566987298108,12.55));
#84129=CARTESIAN_POINT('',(5.1,138.133974596216,13.3));
#84130=CARTESIAN_POINT('Origin',(6.6,139.433012701892,12.55));
#84131=CARTESIAN_POINT('',(6.6,139.216506350946,12.55));
#84132=CARTESIAN_POINT('',(5.1,139.433012701892,12.55));
#84133=CARTESIAN_POINT('',(6.6,139.433012701892,12.55));
#84134=CARTESIAN_POINT('',(5.1,138.566987298108,12.55));
#84135=CARTESIAN_POINT('Origin',(6.6,139.,13.3));
#84136=CARTESIAN_POINT('Origin',(6.6,139.,13.3));
#84137=CARTESIAN_POINT('Origin',(6.6,139.,13.3));
#84138=CARTESIAN_POINT('',(6.6,139.757772228311,13.1125));
#84139=CARTESIAN_POINT('Origin',(6.6,139.,13.3));
#84140=CARTESIAN_POINT('Origin',(6.6,139.,13.3));
#84141=CARTESIAN_POINT('',(6.6,139.541265877365,13.8625));
#84142=CARTESIAN_POINT('Origin',(6.6,139.,13.3));
#84143=CARTESIAN_POINT('',(6.6,138.783493649054,14.05));
#84144=CARTESIAN_POINT('Origin',(5.1,139.,13.3));
#84145=CARTESIAN_POINT('',(5.1,139.433012701892,14.05));
#84146=CARTESIAN_POINT('',(5.1,139.866025403784,13.3));
#84147=CARTESIAN_POINT('',(5.1,139.866025403784,13.3));
#84148=CARTESIAN_POINT('Origin',(5.1,139.,13.3));
#84149=CARTESIAN_POINT('Origin',(5.1,139.,13.3));
#84150=CARTESIAN_POINT('',(5.1,139.433012701892,12.55));
#84151=CARTESIAN_POINT('Origin',(5.1,139.,13.3));
#84152=CARTESIAN_POINT('Origin',(5.1,139.,13.3));
#84153=CARTESIAN_POINT('Origin',(5.1,139.,13.3));
#84154=CARTESIAN_POINT('Origin',(5.1,139.,13.3));
#84155=CARTESIAN_POINT('Origin',(5.1,139.,13.3));
#84156=CARTESIAN_POINT('Origin',(5.1,139.,13.3));
#84157=CARTESIAN_POINT('Origin',(5.1,139.,13.3));
#84158=CARTESIAN_POINT('Origin',(5.1,139.,13.3));
#84159=CARTESIAN_POINT('',(5.1,139.433012701892,14.05));
#84160=CARTESIAN_POINT('Origin',(5.1,139.,13.3));
#84161=CARTESIAN_POINT('Origin',(4.83981971989424,139.,13.3));
#84162=CARTESIAN_POINT('',(4.57963943978849,139.,13.3));
#84163=CARTESIAN_POINT('',(4.83981971989424,138.566987298108,13.3));
#84164=CARTESIAN_POINT('Origin',(6.6,139.433012701892,14.05));
#84165=CARTESIAN_POINT('',(6.6,139.433012701892,14.05));
#84166=CARTESIAN_POINT('',(6.6,139.866025403784,13.3));
#84167=CARTESIAN_POINT('Origin',(6.6,138.566987298108,14.05));
#84168=CARTESIAN_POINT('Origin',(6.6,139.866025403784,13.3));
#84169=CARTESIAN_POINT('Origin',(1.6,140.,13.3));
#84170=CARTESIAN_POINT('',(1.6,138.,13.3));
#84171=CARTESIAN_POINT('Origin',(1.6,139.,13.3));
#84172=CARTESIAN_POINT('Origin',(1.85,139.,13.3));
#84173=CARTESIAN_POINT('',(1.85,137.75,13.3));
#84174=CARTESIAN_POINT('Origin',(6.45,139.,13.3));
#84175=CARTESIAN_POINT('',(6.6,137.8,13.3));
#84176=CARTESIAN_POINT('',(6.45,137.65,13.3));
#84177=CARTESIAN_POINT('Origin',(6.6,139.,13.3));
#84178=CARTESIAN_POINT('Origin',(6.6,139.,13.3));
#135262=UNCERTAINTY_MEASURE_WITH_UNIT(LENGTH_MEASURE(0.01),#135283,
'DISTANCE_ACCURACY_VALUE',
'Maximum model space distance between geometric entities at asserted c
onnectivities');
#135267=UNCERTAINTY_MEASURE_WITH_UNIT(LENGTH_MEASURE(0.01),#135283,
'DISTANCE_ACCURACY_VALUE',
'Maximum model space distance between geometric entities at asserted c
onnectivities');
#135277=(
GEOMETRIC_REPRESENTATION_CONTEXT(3)
GLOBAL_UNCERTAINTY_ASSIGNED_CONTEXT((#135262))
GLOBAL_UNIT_ASSIGNED_CONTEXT((#135283,#135285,#135286))
REPRESENTATION_CONTEXT('','3D')
);
#135282=(
GEOMETRIC_REPRESENTATION_CONTEXT(3)
GLOBAL_UNCERTAINTY_ASSIGNED_CONTEXT((#135267))
GLOBAL_UNIT_ASSIGNED_CONTEXT((#135283,#135285,#135286))
REPRESENTATION_CONTEXT('','3D')
);
#135283=(
LENGTH_UNIT()
NAMED_UNIT(*)
SI_UNIT(.MILLI.,.METRE.)
);
#135285=(
NAMED_UNIT(*)
PLANE_ANGLE_UNIT()
SI_UNIT($,.RADIAN.)
);
#135286=(
NAMED_UNIT(*)
SI_UNIT($,.STERADIAN.)
SOLID_ANGLE_UNIT()
);
#135296=SHAPE_DEFINITION_REPRESENTATION(#135310,#135345);
#135310=PRODUCT_DEFINITION_SHAPE('',$,#135360);
#135345=SHAPE_REPRESENTATION('',(#33412),#135277);
#135350=PRODUCT_DEFINITION_CONTEXT('part definition',#135394,'design');
#135360=PRODUCT_DEFINITION('2026-10-15-19-09-11-267',
'ISO 4026 - M3 x 5 - 45H',#135374,#135350);
#135374=PRODUCT_DEFINITION_FORMATION('',$,#135405);
#135394=APPLICATION_CONTEXT(
'Core Data for Automotive Mechanical Design Process');
#135395=PRODUCT_CONTEXT('part definition',#135394,'mechanical');
#135405=PRODUCT('2026-10-15-19-09-11-267','ISO 4026 - M3 x 5 - 45H',$,(#135395));
#135419=PRESENTATION_STYLE_ASSIGNMENT((#135433));
#135433=SURFACE_STYLE_USAGE(.BOTH.,#135447);
#135447=SURFACE_SIDE_STYLE('',(#135461));
#135461=SURFACE_STYLE_FILL_AREA(#135475);
#135475=FILL_AREA_STYLE('Opaque(196,201,207)',(#135489));
#135489=FILL_AREA_STYLE_COLOUR('Opaque(196,201,207)',#135503);
#135503=COLOUR_RGB('Opaque(196,201,207)', 0.31764706, 0.68627451, 0.89019608);
ENDSEC;
END-ISO-10303-21;
